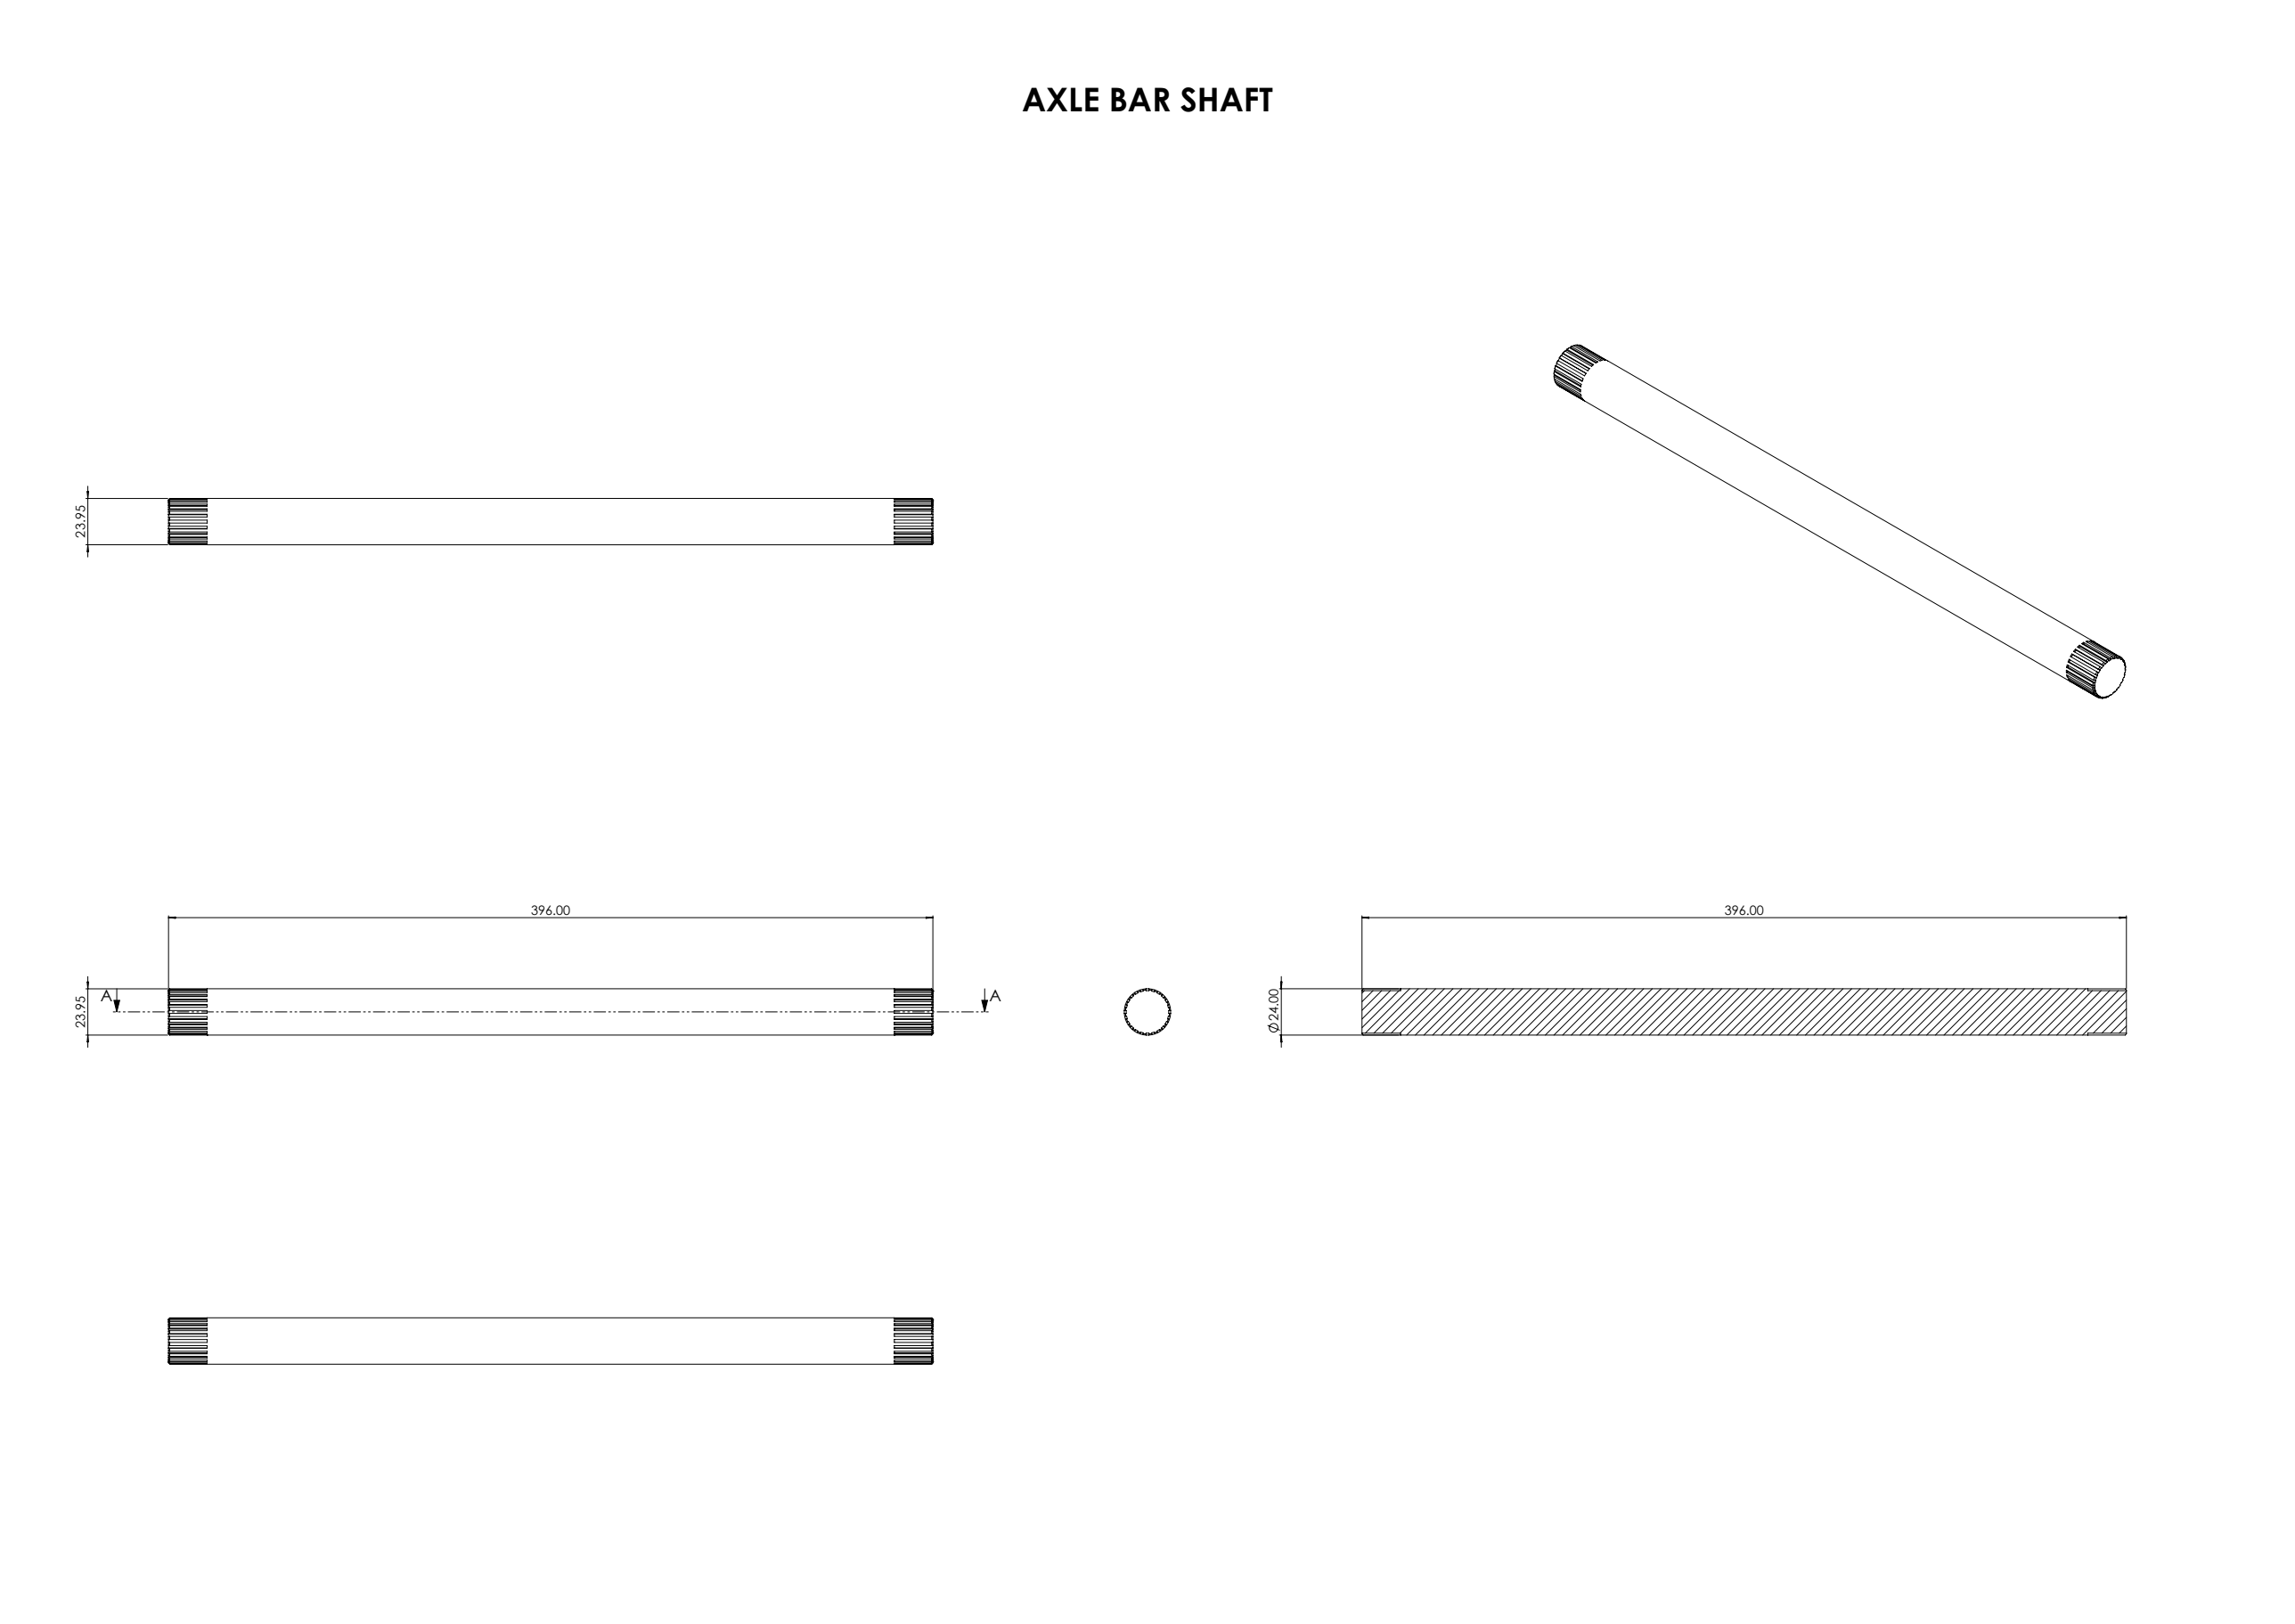
ISO-10303-21;
HEADER;
/* Generated by software containing ST-Developer
 * from STEP Tools, Inc. (www.steptools.com) 
 */

FILE_DESCRIPTION(
/* description */ (''),
/* implementation_level */ '2;1');

FILE_NAME(
/* name */ '10_Axle_Bar_Shaft.step',
/* time_stamp */ '2026-10-11T12:57:03-07:00',
/* author */ (''),
/* organization */ (''),
/* preprocessor_version */ 'ST-DEVELOPER v20.2',
/* originating_system */ 'Autodesk Translation Framework v15.15.0.0',
/* authorisation */ '');

FILE_SCHEMA (('AUTOMOTIVE_DESIGN { 1 0 10303 214 3 1 1 }'));
ENDSEC;

DATA;
#10=MECHANICAL_DESIGN_GEOMETRIC_PRESENTATION_REPRESENTATION('',(#265),#90374);
#231=SHAPE_REPRESENTATION_RELATIONSHIP('SRR','None',#90450,#248);
#248=ADVANCED_BREP_SHAPE_REPRESENTATION('',(#282),#90366);
#265=STYLED_ITEM('',(#90687),#282);
#282=MANIFOLD_SOLID_BREP('Body1',#40354);
#693=CONICAL_SURFACE('',#43949,11.7,0.785398163397428);
#694=CONICAL_SURFACE('',#43951,11.7,0.785398163397428);
#695=CONICAL_SURFACE('',#43957,11.7,0.785398163397428);
#696=CONICAL_SURFACE('',#43963,11.7,0.785398163397428);
#697=CONICAL_SURFACE('',#43969,11.7,0.785398163397428);
#698=CONICAL_SURFACE('',#43975,11.7,0.785398163397428);
#699=CONICAL_SURFACE('',#43981,11.7,0.785398163397428);
#700=CONICAL_SURFACE('',#43987,11.7,0.785398163397428);
#701=CONICAL_SURFACE('',#43993,11.7,0.785398163397428);
#702=CONICAL_SURFACE('',#43999,11.7,0.785398163397428);
#703=CONICAL_SURFACE('',#44005,11.7,0.785398163397428);
#704=CONICAL_SURFACE('',#44011,11.7,0.785398163397428);
#705=CONICAL_SURFACE('',#44017,11.7,0.785398163397428);
#706=CONICAL_SURFACE('',#44023,11.7,0.785398163397428);
#707=CONICAL_SURFACE('',#44029,11.7,0.785398163397428);
#708=CONICAL_SURFACE('',#44035,11.7,0.785398163397428);
#709=CONICAL_SURFACE('',#44041,11.7,0.785398163397428);
#710=CONICAL_SURFACE('',#44047,11.7,0.785398163397428);
#711=CONICAL_SURFACE('',#44053,11.7,0.785398163397428);
#712=CONICAL_SURFACE('',#44059,11.7,0.785398163397428);
#713=CONICAL_SURFACE('',#44065,11.7,0.785398163397428);
#714=CONICAL_SURFACE('',#44071,11.7,0.785398163397428);
#715=CONICAL_SURFACE('',#44077,11.7,0.785398163397428);
#716=CONICAL_SURFACE('',#44083,11.7,0.785398163397428);
#717=CONICAL_SURFACE('',#44118,11.7,0.785398163397457);
#718=CONICAL_SURFACE('',#44119,11.7,0.785398163397457);
#719=CONICAL_SURFACE('',#44124,11.7,0.785398163397457);
#720=CONICAL_SURFACE('',#44129,11.7,0.785398163397457);
#721=CONICAL_SURFACE('',#44134,11.7,0.785398163397457);
#722=CONICAL_SURFACE('',#44139,11.7,0.785398163397457);
#723=CONICAL_SURFACE('',#44144,11.7,0.785398163397457);
#724=CONICAL_SURFACE('',#44149,11.7,0.785398163397457);
#725=CONICAL_SURFACE('',#44154,11.7,0.785398163397457);
#726=CONICAL_SURFACE('',#44159,11.7,0.785398163397457);
#727=CONICAL_SURFACE('',#44164,11.7,0.785398163397457);
#728=CONICAL_SURFACE('',#44169,11.7,0.785398163397457);
#729=CONICAL_SURFACE('',#44174,11.7,0.785398163397457);
#730=CONICAL_SURFACE('',#44179,11.7,0.785398163397457);
#731=CONICAL_SURFACE('',#44184,11.7,0.785398163397457);
#732=CONICAL_SURFACE('',#44189,11.7,0.785398163397457);
#733=CONICAL_SURFACE('',#44194,11.7,0.785398163397457);
#734=CONICAL_SURFACE('',#44199,11.7,0.785398163397457);
#735=CONICAL_SURFACE('',#44204,11.7,0.785398163397457);
#736=CONICAL_SURFACE('',#44209,11.7,0.785398163397457);
#737=CONICAL_SURFACE('',#44214,11.7,0.785398163397457);
#738=CONICAL_SURFACE('',#44219,11.7,0.785398163397457);
#739=CONICAL_SURFACE('',#44224,11.7,0.785398163397457);
#740=CONICAL_SURFACE('',#44229,11.7,0.785398163397457);
#1443=PLANE('',#43846);
#1444=PLANE('',#43847);
#1445=PLANE('',#43849);
#1446=PLANE('',#43850);
#1447=PLANE('',#43953);
#1448=PLANE('',#43954);
#1449=PLANE('',#43955);
#1450=PLANE('',#43956);
#1451=PLANE('',#43959);
#1452=PLANE('',#43960);
#1453=PLANE('',#43961);
#1454=PLANE('',#43962);
#1455=PLANE('',#43965);
#1456=PLANE('',#43966);
#1457=PLANE('',#43967);
#1458=PLANE('',#43968);
#1459=PLANE('',#43971);
#1460=PLANE('',#43972);
#1461=PLANE('',#43973);
#1462=PLANE('',#43974);
#1463=PLANE('',#43977);
#1464=PLANE('',#43978);
#1465=PLANE('',#43979);
#1466=PLANE('',#43980);
#1467=PLANE('',#43983);
#1468=PLANE('',#43984);
#1469=PLANE('',#43985);
#1470=PLANE('',#43986);
#1471=PLANE('',#43989);
#1472=PLANE('',#43990);
#1473=PLANE('',#43991);
#1474=PLANE('',#43992);
#1475=PLANE('',#43995);
#1476=PLANE('',#43996);
#1477=PLANE('',#43997);
#1478=PLANE('',#43998);
#1479=PLANE('',#44001);
#1480=PLANE('',#44002);
#1481=PLANE('',#44003);
#1482=PLANE('',#44004);
#1483=PLANE('',#44007);
#1484=PLANE('',#44008);
#1485=PLANE('',#44009);
#1486=PLANE('',#44010);
#1487=PLANE('',#44013);
#1488=PLANE('',#44014);
#1489=PLANE('',#44015);
#1490=PLANE('',#44016);
#1491=PLANE('',#44019);
#1492=PLANE('',#44020);
#1493=PLANE('',#44021);
#1494=PLANE('',#44022);
#1495=PLANE('',#44025);
#1496=PLANE('',#44026);
#1497=PLANE('',#44027);
#1498=PLANE('',#44028);
#1499=PLANE('',#44031);
#1500=PLANE('',#44032);
#1501=PLANE('',#44033);
#1502=PLANE('',#44034);
#1503=PLANE('',#44037);
#1504=PLANE('',#44038);
#1505=PLANE('',#44039);
#1506=PLANE('',#44040);
#1507=PLANE('',#44043);
#1508=PLANE('',#44044);
#1509=PLANE('',#44045);
#1510=PLANE('',#44046);
#1511=PLANE('',#44049);
#1512=PLANE('',#44050);
#1513=PLANE('',#44051);
#1514=PLANE('',#44052);
#1515=PLANE('',#44055);
#1516=PLANE('',#44056);
#1517=PLANE('',#44057);
#1518=PLANE('',#44058);
#1519=PLANE('',#44061);
#1520=PLANE('',#44062);
#1521=PLANE('',#44063);
#1522=PLANE('',#44064);
#1523=PLANE('',#44067);
#1524=PLANE('',#44068);
#1525=PLANE('',#44069);
#1526=PLANE('',#44070);
#1527=PLANE('',#44073);
#1528=PLANE('',#44074);
#1529=PLANE('',#44075);
#1530=PLANE('',#44076);
#1531=PLANE('',#44079);
#1532=PLANE('',#44080);
#1533=PLANE('',#44081);
#1534=PLANE('',#44082);
#1535=PLANE('',#44085);
#1536=PLANE('',#44086);
#1537=PLANE('',#44087);
#1538=PLANE('',#44088);
#1539=PLANE('',#44089);
#1540=PLANE('',#44090);
#1541=PLANE('',#44091);
#1542=PLANE('',#44092);
#1543=PLANE('',#44093);
#1544=PLANE('',#44120);
#1545=PLANE('',#44121);
#1546=PLANE('',#44122);
#1547=PLANE('',#44123);
#1548=PLANE('',#44125);
#1549=PLANE('',#44126);
#1550=PLANE('',#44127);
#1551=PLANE('',#44128);
#1552=PLANE('',#44130);
#1553=PLANE('',#44131);
#1554=PLANE('',#44132);
#1555=PLANE('',#44133);
#1556=PLANE('',#44135);
#1557=PLANE('',#44136);
#1558=PLANE('',#44137);
#1559=PLANE('',#44138);
#1560=PLANE('',#44140);
#1561=PLANE('',#44141);
#1562=PLANE('',#44142);
#1563=PLANE('',#44143);
#1564=PLANE('',#44145);
#1565=PLANE('',#44146);
#1566=PLANE('',#44147);
#1567=PLANE('',#44148);
#1568=PLANE('',#44150);
#1569=PLANE('',#44151);
#1570=PLANE('',#44152);
#1571=PLANE('',#44153);
#1572=PLANE('',#44155);
#1573=PLANE('',#44156);
#1574=PLANE('',#44157);
#1575=PLANE('',#44158);
#1576=PLANE('',#44160);
#1577=PLANE('',#44161);
#1578=PLANE('',#44162);
#1579=PLANE('',#44163);
#1580=PLANE('',#44165);
#1581=PLANE('',#44166);
#1582=PLANE('',#44167);
#1583=PLANE('',#44168);
#1584=PLANE('',#44170);
#1585=PLANE('',#44171);
#1586=PLANE('',#44172);
#1587=PLANE('',#44173);
#1588=PLANE('',#44175);
#1589=PLANE('',#44176);
#1590=PLANE('',#44177);
#1591=PLANE('',#44178);
#1592=PLANE('',#44180);
#1593=PLANE('',#44181);
#1594=PLANE('',#44182);
#1595=PLANE('',#44183);
#1596=PLANE('',#44185);
#1597=PLANE('',#44186);
#1598=PLANE('',#44187);
#1599=PLANE('',#44188);
#1600=PLANE('',#44190);
#1601=PLANE('',#44191);
#1602=PLANE('',#44192);
#1603=PLANE('',#44193);
#1604=PLANE('',#44195);
#1605=PLANE('',#44196);
#1606=PLANE('',#44197);
#1607=PLANE('',#44198);
#1608=PLANE('',#44200);
#1609=PLANE('',#44201);
#1610=PLANE('',#44202);
#1611=PLANE('',#44203);
#1612=PLANE('',#44205);
#1613=PLANE('',#44206);
#1614=PLANE('',#44207);
#1615=PLANE('',#44208);
#1616=PLANE('',#44210);
#1617=PLANE('',#44211);
#1618=PLANE('',#44212);
#1619=PLANE('',#44213);
#1620=PLANE('',#44215);
#1621=PLANE('',#44216);
#1622=PLANE('',#44217);
#1623=PLANE('',#44218);
#1624=PLANE('',#44220);
#1625=PLANE('',#44221);
#1626=PLANE('',#44222);
#1627=PLANE('',#44223);
#1628=PLANE('',#44225);
#1629=PLANE('',#44226);
#1630=PLANE('',#44227);
#1631=PLANE('',#44228);
#1632=PLANE('',#44230);
#1633=PLANE('',#44231);
#1634=PLANE('',#44232);
#1635=PLANE('',#44233);
#1636=PLANE('',#44234);
#1833=(
BOUNDED_CURVE()
B_SPLINE_CURVE(2,(#83032,#83033,#83034),.UNSPECIFIED.,.F.,.F.)
B_SPLINE_CURVE_WITH_KNOTS((3,3),(0.,0.0849403543350642),.UNSPECIFIED.)
CURVE()
GEOMETRIC_REPRESENTATION_ITEM()
RATIONAL_B_SPLINE_CURVE((1.,1.00033025160276,1.))
REPRESENTATION_ITEM('')
);
#1834=(
BOUNDED_CURVE()
B_SPLINE_CURVE(2,(#83046,#83047,#83048),.UNSPECIFIED.,.F.,.F.)
B_SPLINE_CURVE_WITH_KNOTS((3,3),(0.,0.0849403543350645),.UNSPECIFIED.)
CURVE()
GEOMETRIC_REPRESENTATION_ITEM()
RATIONAL_B_SPLINE_CURVE((1.,1.00033025241417,1.))
REPRESENTATION_ITEM('')
);
#1835=(
BOUNDED_CURVE()
B_SPLINE_CURVE(2,(#83439,#83440,#83441),.UNSPECIFIED.,.F.,.F.)
B_SPLINE_CURVE_WITH_KNOTS((3,3),(0.,0.0849403543350642),.UNSPECIFIED.)
CURVE()
GEOMETRIC_REPRESENTATION_ITEM()
RATIONAL_B_SPLINE_CURVE((1.,1.00033025173132,1.))
REPRESENTATION_ITEM('')
);
#1836=(
BOUNDED_CURVE()
B_SPLINE_CURVE(2,(#83444,#83445,#83446),.UNSPECIFIED.,.F.,.F.)
B_SPLINE_CURVE_WITH_KNOTS((3,3),(0.,0.0849403543350642),.UNSPECIFIED.)
CURVE()
GEOMETRIC_REPRESENTATION_ITEM()
RATIONAL_B_SPLINE_CURVE((1.,1.00033025019403,1.))
REPRESENTATION_ITEM('')
);
#1837=(
BOUNDED_CURVE()
B_SPLINE_CURVE(2,(#83462,#83463,#83464),.UNSPECIFIED.,.F.,.F.)
B_SPLINE_CURVE_WITH_KNOTS((3,3),(0.,0.0849403543350642),.UNSPECIFIED.)
CURVE()
GEOMETRIC_REPRESENTATION_ITEM()
RATIONAL_B_SPLINE_CURVE((1.,1.00033025228575,1.))
REPRESENTATION_ITEM('')
);
#1838=(
BOUNDED_CURVE()
B_SPLINE_CURVE(2,(#83471,#83472,#83473),.UNSPECIFIED.,.F.,.F.)
B_SPLINE_CURVE_WITH_KNOTS((3,3),(0.,0.0849403543350642),.UNSPECIFIED.)
CURVE()
GEOMETRIC_REPRESENTATION_ITEM()
RATIONAL_B_SPLINE_CURVE((1.,1.00033024976505,1.))
REPRESENTATION_ITEM('')
);
#1839=(
BOUNDED_CURVE()
B_SPLINE_CURVE(2,(#83488,#83489,#83490),.UNSPECIFIED.,.F.,.F.)
B_SPLINE_CURVE_WITH_KNOTS((3,3),(0.,0.0849403543350642),.UNSPECIFIED.)
CURVE()
GEOMETRIC_REPRESENTATION_ITEM()
RATIONAL_B_SPLINE_CURVE((1.,1.00033025048873,1.))
REPRESENTATION_ITEM('')
);
#1840=(
BOUNDED_CURVE()
B_SPLINE_CURVE(2,(#83497,#83498,#83499),.UNSPECIFIED.,.F.,.F.)
B_SPLINE_CURVE_WITH_KNOTS((3,3),(0.,0.0849403543350643),.UNSPECIFIED.)
CURVE()
GEOMETRIC_REPRESENTATION_ITEM()
RATIONAL_B_SPLINE_CURVE((1.,1.00033025205034,1.))
REPRESENTATION_ITEM('')
);
#1841=(
BOUNDED_CURVE()
B_SPLINE_CURVE(2,(#83514,#83515,#83516),.UNSPECIFIED.,.F.,.F.)
B_SPLINE_CURVE_WITH_KNOTS((3,3),(0.,0.084940354335064),.UNSPECIFIED.)
CURVE()
GEOMETRIC_REPRESENTATION_ITEM()
RATIONAL_B_SPLINE_CURVE((1.,1.00033025029154,1.))
REPRESENTATION_ITEM('')
);
#1842=(
BOUNDED_CURVE()
B_SPLINE_CURVE(2,(#83523,#83524,#83525),.UNSPECIFIED.,.F.,.F.)
B_SPLINE_CURVE_WITH_KNOTS((3,3),(0.,0.0849403543350643),.UNSPECIFIED.)
CURVE()
GEOMETRIC_REPRESENTATION_ITEM()
RATIONAL_B_SPLINE_CURVE((1.,1.00033025291298,1.))
REPRESENTATION_ITEM('')
);
#1843=(
BOUNDED_CURVE()
B_SPLINE_CURVE(2,(#83540,#83541,#83542),.UNSPECIFIED.,.F.,.F.)
B_SPLINE_CURVE_WITH_KNOTS((3,3),(0.,0.0849403543350644),.UNSPECIFIED.)
CURVE()
GEOMETRIC_REPRESENTATION_ITEM()
RATIONAL_B_SPLINE_CURVE((1.,1.00033025022527,1.))
REPRESENTATION_ITEM('')
);
#1844=(
BOUNDED_CURVE()
B_SPLINE_CURVE(2,(#83549,#83550,#83551),.UNSPECIFIED.,.F.,.F.)
B_SPLINE_CURVE_WITH_KNOTS((3,3),(0.,0.0849403543350642),.UNSPECIFIED.)
CURVE()
GEOMETRIC_REPRESENTATION_ITEM()
RATIONAL_B_SPLINE_CURVE((1.,1.00033025176016,1.))
REPRESENTATION_ITEM('')
);
#1845=(
BOUNDED_CURVE()
B_SPLINE_CURVE(2,(#83566,#83567,#83568),.UNSPECIFIED.,.F.,.F.)
B_SPLINE_CURVE_WITH_KNOTS((3,3),(0.,0.0849403543350642),.UNSPECIFIED.)
CURVE()
GEOMETRIC_REPRESENTATION_ITEM()
RATIONAL_B_SPLINE_CURVE((1.,1.00033025172446,1.))
REPRESENTATION_ITEM('')
);
#1846=(
BOUNDED_CURVE()
B_SPLINE_CURVE(2,(#83575,#83576,#83577),.UNSPECIFIED.,.F.,.F.)
B_SPLINE_CURVE_WITH_KNOTS((3,3),(0.,0.0849403543350642),.UNSPECIFIED.)
CURVE()
GEOMETRIC_REPRESENTATION_ITEM()
RATIONAL_B_SPLINE_CURVE((1.,1.00033025024162,1.))
REPRESENTATION_ITEM('')
);
#1847=(
BOUNDED_CURVE()
B_SPLINE_CURVE(2,(#83592,#83593,#83594),.UNSPECIFIED.,.F.,.F.)
B_SPLINE_CURVE_WITH_KNOTS((3,3),(0.,0.0849403543350645),.UNSPECIFIED.)
CURVE()
GEOMETRIC_REPRESENTATION_ITEM()
RATIONAL_B_SPLINE_CURVE((1.,1.00033025047704,1.))
REPRESENTATION_ITEM('')
);
#1848=(
BOUNDED_CURVE()
B_SPLINE_CURVE(2,(#83601,#83602,#83603),.UNSPECIFIED.,.F.,.F.)
B_SPLINE_CURVE_WITH_KNOTS((3,3),(0.,0.0849403543350642),.UNSPECIFIED.)
CURVE()
GEOMETRIC_REPRESENTATION_ITEM()
RATIONAL_B_SPLINE_CURVE((1.,1.0003302538932,1.))
REPRESENTATION_ITEM('')
);
#1849=(
BOUNDED_CURVE()
B_SPLINE_CURVE(2,(#83618,#83619,#83620),.UNSPECIFIED.,.F.,.F.)
B_SPLINE_CURVE_WITH_KNOTS((3,3),(0.,0.0849403543350642),.UNSPECIFIED.)
CURVE()
GEOMETRIC_REPRESENTATION_ITEM()
RATIONAL_B_SPLINE_CURVE((1.,1.00033025055311,1.))
REPRESENTATION_ITEM('')
);
#1850=(
BOUNDED_CURVE()
B_SPLINE_CURVE(2,(#83627,#83628,#83629),.UNSPECIFIED.,.F.,.F.)
B_SPLINE_CURVE_WITH_KNOTS((3,3),(0.,0.0849403543350642),.UNSPECIFIED.)
CURVE()
GEOMETRIC_REPRESENTATION_ITEM()
RATIONAL_B_SPLINE_CURVE((1.,1.00033025068821,1.))
REPRESENTATION_ITEM('')
);
#1851=(
BOUNDED_CURVE()
B_SPLINE_CURVE(2,(#83644,#83645,#83646),.UNSPECIFIED.,.F.,.F.)
B_SPLINE_CURVE_WITH_KNOTS((3,3),(0.,0.0849403543350642),.UNSPECIFIED.)
CURVE()
GEOMETRIC_REPRESENTATION_ITEM()
RATIONAL_B_SPLINE_CURVE((1.,1.00033025088247,1.))
REPRESENTATION_ITEM('')
);
#1852=(
BOUNDED_CURVE()
B_SPLINE_CURVE(2,(#83653,#83654,#83655),.UNSPECIFIED.,.F.,.F.)
B_SPLINE_CURVE_WITH_KNOTS((3,3),(0.,0.0849403543350642),.UNSPECIFIED.)
CURVE()
GEOMETRIC_REPRESENTATION_ITEM()
RATIONAL_B_SPLINE_CURVE((1.,1.00033025566741,1.))
REPRESENTATION_ITEM('')
);
#1853=(
BOUNDED_CURVE()
B_SPLINE_CURVE(2,(#83670,#83671,#83672),.UNSPECIFIED.,.F.,.F.)
B_SPLINE_CURVE_WITH_KNOTS((3,3),(0.,0.0849403543350643),.UNSPECIFIED.)
CURVE()
GEOMETRIC_REPRESENTATION_ITEM()
RATIONAL_B_SPLINE_CURVE((1.,1.00033025086662,1.))
REPRESENTATION_ITEM('')
);
#1854=(
BOUNDED_CURVE()
B_SPLINE_CURVE(2,(#83679,#83680,#83681),.UNSPECIFIED.,.F.,.F.)
B_SPLINE_CURVE_WITH_KNOTS((3,3),(0.,0.0849403543350643),.UNSPECIFIED.)
CURVE()
GEOMETRIC_REPRESENTATION_ITEM()
RATIONAL_B_SPLINE_CURVE((1.,1.00033025126855,1.))
REPRESENTATION_ITEM('')
);
#1855=(
BOUNDED_CURVE()
B_SPLINE_CURVE(2,(#83696,#83697,#83698),.UNSPECIFIED.,.F.,.F.)
B_SPLINE_CURVE_WITH_KNOTS((3,3),(0.,0.0849403543350644),.UNSPECIFIED.)
CURVE()
GEOMETRIC_REPRESENTATION_ITEM()
RATIONAL_B_SPLINE_CURVE((1.,1.00033025048324,1.))
REPRESENTATION_ITEM('')
);
#1856=(
BOUNDED_CURVE()
B_SPLINE_CURVE(2,(#83705,#83706,#83707),.UNSPECIFIED.,.F.,.F.)
B_SPLINE_CURVE_WITH_KNOTS((3,3),(0.,0.0849403543350642),.UNSPECIFIED.)
CURVE()
GEOMETRIC_REPRESENTATION_ITEM()
RATIONAL_B_SPLINE_CURVE((1.,1.00033025019805,1.))
REPRESENTATION_ITEM('')
);
#1857=(
BOUNDED_CURVE()
B_SPLINE_CURVE(2,(#83722,#83723,#83724),.UNSPECIFIED.,.F.,.F.)
B_SPLINE_CURVE_WITH_KNOTS((3,3),(0.,0.0849403543350642),.UNSPECIFIED.)
CURVE()
GEOMETRIC_REPRESENTATION_ITEM()
RATIONAL_B_SPLINE_CURVE((1.,1.00033025018713,1.))
REPRESENTATION_ITEM('')
);
#1858=(
BOUNDED_CURVE()
B_SPLINE_CURVE(2,(#83731,#83732,#83733),.UNSPECIFIED.,.F.,.F.)
B_SPLINE_CURVE_WITH_KNOTS((3,3),(0.,0.0849403543350641),.UNSPECIFIED.)
CURVE()
GEOMETRIC_REPRESENTATION_ITEM()
RATIONAL_B_SPLINE_CURVE((1.,1.00033025306809,1.))
REPRESENTATION_ITEM('')
);
#1859=(
BOUNDED_CURVE()
B_SPLINE_CURVE(2,(#83748,#83749,#83750),.UNSPECIFIED.,.F.,.F.)
B_SPLINE_CURVE_WITH_KNOTS((3,3),(0.,0.0849403543350642),.UNSPECIFIED.)
CURVE()
GEOMETRIC_REPRESENTATION_ITEM()
RATIONAL_B_SPLINE_CURVE((1.,1.00033025283671,1.))
REPRESENTATION_ITEM('')
);
#1860=(
BOUNDED_CURVE()
B_SPLINE_CURVE(2,(#83757,#83758,#83759),.UNSPECIFIED.,.F.,.F.)
B_SPLINE_CURVE_WITH_KNOTS((3,3),(0.,0.0849403543350642),.UNSPECIFIED.)
CURVE()
GEOMETRIC_REPRESENTATION_ITEM()
RATIONAL_B_SPLINE_CURVE((1.,1.00033025201275,1.))
REPRESENTATION_ITEM('')
);
#1861=(
BOUNDED_CURVE()
B_SPLINE_CURVE(2,(#83774,#83775,#83776),.UNSPECIFIED.,.F.,.F.)
B_SPLINE_CURVE_WITH_KNOTS((3,3),(0.,0.0849403543350643),.UNSPECIFIED.)
CURVE()
GEOMETRIC_REPRESENTATION_ITEM()
RATIONAL_B_SPLINE_CURVE((1.,1.0003302506393,1.))
REPRESENTATION_ITEM('')
);
#1862=(
BOUNDED_CURVE()
B_SPLINE_CURVE(2,(#83783,#83784,#83785),.UNSPECIFIED.,.F.,.F.)
B_SPLINE_CURVE_WITH_KNOTS((3,3),(0.,0.0849403543350642),.UNSPECIFIED.)
CURVE()
GEOMETRIC_REPRESENTATION_ITEM()
RATIONAL_B_SPLINE_CURVE((1.,1.00033025057128,1.))
REPRESENTATION_ITEM('')
);
#1863=(
BOUNDED_CURVE()
B_SPLINE_CURVE(2,(#83800,#83801,#83802),.UNSPECIFIED.,.F.,.F.)
B_SPLINE_CURVE_WITH_KNOTS((3,3),(0.,0.0849403543350642),.UNSPECIFIED.)
CURVE()
GEOMETRIC_REPRESENTATION_ITEM()
RATIONAL_B_SPLINE_CURVE((1.,1.00033025068354,1.))
REPRESENTATION_ITEM('')
);
#1864=(
BOUNDED_CURVE()
B_SPLINE_CURVE(2,(#83809,#83810,#83811),.UNSPECIFIED.,.F.,.F.)
B_SPLINE_CURVE_WITH_KNOTS((3,3),(0.,0.0849403543350641),.UNSPECIFIED.)
CURVE()
GEOMETRIC_REPRESENTATION_ITEM()
RATIONAL_B_SPLINE_CURVE((1.,1.0003302507014,1.))
REPRESENTATION_ITEM('')
);
#1865=(
BOUNDED_CURVE()
B_SPLINE_CURVE(2,(#83826,#83827,#83828),.UNSPECIFIED.,.F.,.F.)
B_SPLINE_CURVE_WITH_KNOTS((3,3),(0.,0.0849403543350642),.UNSPECIFIED.)
CURVE()
GEOMETRIC_REPRESENTATION_ITEM()
RATIONAL_B_SPLINE_CURVE((1.,1.00033024942034,1.))
REPRESENTATION_ITEM('')
);
#1866=(
BOUNDED_CURVE()
B_SPLINE_CURVE(2,(#83835,#83836,#83837),.UNSPECIFIED.,.F.,.F.)
B_SPLINE_CURVE_WITH_KNOTS((3,3),(0.,0.0849403543350642),.UNSPECIFIED.)
CURVE()
GEOMETRIC_REPRESENTATION_ITEM()
RATIONAL_B_SPLINE_CURVE((1.,1.00033025025859,1.))
REPRESENTATION_ITEM('')
);
#1867=(
BOUNDED_CURVE()
B_SPLINE_CURVE(2,(#83852,#83853,#83854),.UNSPECIFIED.,.F.,.F.)
B_SPLINE_CURVE_WITH_KNOTS((3,3),(0.,0.0849403543350642),.UNSPECIFIED.)
CURVE()
GEOMETRIC_REPRESENTATION_ITEM()
RATIONAL_B_SPLINE_CURVE((1.,1.00033025417478,1.))
REPRESENTATION_ITEM('')
);
#1868=(
BOUNDED_CURVE()
B_SPLINE_CURVE(2,(#83861,#83862,#83863),.UNSPECIFIED.,.F.,.F.)
B_SPLINE_CURVE_WITH_KNOTS((3,3),(0.,0.0849403543350642),.UNSPECIFIED.)
CURVE()
GEOMETRIC_REPRESENTATION_ITEM()
RATIONAL_B_SPLINE_CURVE((1.,1.00033025175498,1.))
REPRESENTATION_ITEM('')
);
#1869=(
BOUNDED_CURVE()
B_SPLINE_CURVE(2,(#83878,#83879,#83880),.UNSPECIFIED.,.F.,.F.)
B_SPLINE_CURVE_WITH_KNOTS((3,3),(0.,0.0849403543350642),.UNSPECIFIED.)
CURVE()
GEOMETRIC_REPRESENTATION_ITEM()
RATIONAL_B_SPLINE_CURVE((1.,1.00033025172964,1.))
REPRESENTATION_ITEM('')
);
#1870=(
BOUNDED_CURVE()
B_SPLINE_CURVE(2,(#83887,#83888,#83889),.UNSPECIFIED.,.F.,.F.)
B_SPLINE_CURVE_WITH_KNOTS((3,3),(0.,0.0849403543350641),.UNSPECIFIED.)
CURVE()
GEOMETRIC_REPRESENTATION_ITEM()
RATIONAL_B_SPLINE_CURVE((1.,1.00033025185005,1.))
REPRESENTATION_ITEM('')
);
#1871=(
BOUNDED_CURVE()
B_SPLINE_CURVE(2,(#83904,#83905,#83906),.UNSPECIFIED.,.F.,.F.)
B_SPLINE_CURVE_WITH_KNOTS((3,3),(0.,0.0849403543350642),.UNSPECIFIED.)
CURVE()
GEOMETRIC_REPRESENTATION_ITEM()
RATIONAL_B_SPLINE_CURVE((1.,1.00033024993968,1.))
REPRESENTATION_ITEM('')
);
#1872=(
BOUNDED_CURVE()
B_SPLINE_CURVE(2,(#83913,#83914,#83915),.UNSPECIFIED.,.F.,.F.)
B_SPLINE_CURVE_WITH_KNOTS((3,3),(0.,0.084940354335064),.UNSPECIFIED.)
CURVE()
GEOMETRIC_REPRESENTATION_ITEM()
RATIONAL_B_SPLINE_CURVE((1.,1.00033025201589,1.))
REPRESENTATION_ITEM('')
);
#1873=(
BOUNDED_CURVE()
B_SPLINE_CURVE(2,(#83930,#83931,#83932),.UNSPECIFIED.,.F.,.F.)
B_SPLINE_CURVE_WITH_KNOTS((3,3),(0.,0.0849403543350641),.UNSPECIFIED.)
CURVE()
GEOMETRIC_REPRESENTATION_ITEM()
RATIONAL_B_SPLINE_CURVE((1.,1.00033025407768,1.))
REPRESENTATION_ITEM('')
);
#1874=(
BOUNDED_CURVE()
B_SPLINE_CURVE(2,(#83939,#83940,#83941),.UNSPECIFIED.,.F.,.F.)
B_SPLINE_CURVE_WITH_KNOTS((3,3),(0.,0.0849403543350642),.UNSPECIFIED.)
CURVE()
GEOMETRIC_REPRESENTATION_ITEM()
RATIONAL_B_SPLINE_CURVE((1.,1.00033025202778,1.))
REPRESENTATION_ITEM('')
);
#1875=(
BOUNDED_CURVE()
B_SPLINE_CURVE(2,(#83956,#83957,#83958),.UNSPECIFIED.,.F.,.F.)
B_SPLINE_CURVE_WITH_KNOTS((3,3),(0.,0.0849403543350642),.UNSPECIFIED.)
CURVE()
GEOMETRIC_REPRESENTATION_ITEM()
RATIONAL_B_SPLINE_CURVE((1.,1.00033025202127,1.))
REPRESENTATION_ITEM('')
);
#1876=(
BOUNDED_CURVE()
B_SPLINE_CURVE(2,(#83965,#83966,#83967),.UNSPECIFIED.,.F.,.F.)
B_SPLINE_CURVE_WITH_KNOTS((3,3),(0.,0.0849403543350642),.UNSPECIFIED.)
CURVE()
GEOMETRIC_REPRESENTATION_ITEM()
RATIONAL_B_SPLINE_CURVE((1.,1.0003302492308,1.))
REPRESENTATION_ITEM('')
);
#1877=(
BOUNDED_CURVE()
B_SPLINE_CURVE(2,(#83982,#83983,#83984),.UNSPECIFIED.,.F.,.F.)
B_SPLINE_CURVE_WITH_KNOTS((3,3),(0.,0.0849403543350642),.UNSPECIFIED.)
CURVE()
GEOMETRIC_REPRESENTATION_ITEM()
RATIONAL_B_SPLINE_CURVE((1.,1.00033024979139,1.))
REPRESENTATION_ITEM('')
);
#1878=(
BOUNDED_CURVE()
B_SPLINE_CURVE(2,(#83991,#83992,#83993),.UNSPECIFIED.,.F.,.F.)
B_SPLINE_CURVE_WITH_KNOTS((3,3),(0.,0.0849403543350642),.UNSPECIFIED.)
CURVE()
GEOMETRIC_REPRESENTATION_ITEM()
RATIONAL_B_SPLINE_CURVE((1.,1.00033024938276,1.))
REPRESENTATION_ITEM('')
);
#1879=(
BOUNDED_CURVE()
B_SPLINE_CURVE(2,(#84008,#84009,#84010),.UNSPECIFIED.,.F.,.F.)
B_SPLINE_CURVE_WITH_KNOTS((3,3),(0.,0.0849403543350641),.UNSPECIFIED.)
CURVE()
GEOMETRIC_REPRESENTATION_ITEM()
RATIONAL_B_SPLINE_CURVE((1.,1.00033025441577,1.))
REPRESENTATION_ITEM('')
);
#1880=(
BOUNDED_CURVE()
B_SPLINE_CURVE(2,(#84017,#84018,#84019),.UNSPECIFIED.,.F.,.F.)
B_SPLINE_CURVE_WITH_KNOTS((3,3),(0.,0.0849403543350642),.UNSPECIFIED.)
CURVE()
GEOMETRIC_REPRESENTATION_ITEM()
RATIONAL_B_SPLINE_CURVE((1.,1.00033025019403,1.))
REPRESENTATION_ITEM('')
);
#1881=(
BOUNDED_CURVE()
B_SPLINE_CURVE(2,(#84043,#84044,#84045),.UNSPECIFIED.,.F.,.F.)
B_SPLINE_CURVE_WITH_KNOTS((3,3),(0.,0.0849403543350617),.UNSPECIFIED.)
CURVE()
GEOMETRIC_REPRESENTATION_ITEM()
RATIONAL_B_SPLINE_CURVE((1.,1.00033025151332,1.))
REPRESENTATION_ITEM('')
);
#1882=(
BOUNDED_CURVE()
B_SPLINE_CURVE(2,(#84054,#84055,#84056),.UNSPECIFIED.,.F.,.F.)
B_SPLINE_CURVE_WITH_KNOTS((3,3),(0.,0.0849403543350617),.UNSPECIFIED.)
CURVE()
GEOMETRIC_REPRESENTATION_ITEM()
RATIONAL_B_SPLINE_CURVE((1.,1.00033025246357,1.))
REPRESENTATION_ITEM('')
);
#1883=(
BOUNDED_CURVE()
B_SPLINE_CURVE(2,(#84247,#84248,#84249),.UNSPECIFIED.,.F.,.F.)
B_SPLINE_CURVE_WITH_KNOTS((3,3),(0.,0.0849403543350617),.UNSPECIFIED.)
CURVE()
GEOMETRIC_REPRESENTATION_ITEM()
RATIONAL_B_SPLINE_CURVE((1.,1.0003302512864,1.))
REPRESENTATION_ITEM('')
);
#1884=(
BOUNDED_CURVE()
B_SPLINE_CURVE(2,(#84251,#84252,#84253),.UNSPECIFIED.,.F.,.F.)
B_SPLINE_CURVE_WITH_KNOTS((3,3),(0.,0.0849403543350617),.UNSPECIFIED.)
CURVE()
GEOMETRIC_REPRESENTATION_ITEM()
RATIONAL_B_SPLINE_CURVE((1.,1.00033025136034,1.))
REPRESENTATION_ITEM('')
);
#1885=(
BOUNDED_CURVE()
B_SPLINE_CURVE(2,(#84263,#84264,#84265),.UNSPECIFIED.,.F.,.F.)
B_SPLINE_CURVE_WITH_KNOTS((3,3),(0.,0.0849403543350619),.UNSPECIFIED.)
CURVE()
GEOMETRIC_REPRESENTATION_ITEM()
RATIONAL_B_SPLINE_CURVE((1.,1.00033025257346,1.))
REPRESENTATION_ITEM('')
);
#1886=(
BOUNDED_CURVE()
B_SPLINE_CURVE(2,(#84269,#84270,#84271),.UNSPECIFIED.,.F.,.F.)
B_SPLINE_CURVE_WITH_KNOTS((3,3),(0.,0.0849403543350618),.UNSPECIFIED.)
CURVE()
GEOMETRIC_REPRESENTATION_ITEM()
RATIONAL_B_SPLINE_CURVE((1.,1.00033025219394,1.))
REPRESENTATION_ITEM('')
);
#1887=(
BOUNDED_CURVE()
B_SPLINE_CURVE(2,(#84281,#84282,#84283),.UNSPECIFIED.,.F.,.F.)
B_SPLINE_CURVE_WITH_KNOTS((3,3),(0.,0.0849403543350616),.UNSPECIFIED.)
CURVE()
GEOMETRIC_REPRESENTATION_ITEM()
RATIONAL_B_SPLINE_CURVE((1.,1.00033025178113,1.))
REPRESENTATION_ITEM('')
);
#1888=(
BOUNDED_CURVE()
B_SPLINE_CURVE(2,(#84287,#84288,#84289),.UNSPECIFIED.,.F.,.F.)
B_SPLINE_CURVE_WITH_KNOTS((3,3),(0.,0.0849403543350617),.UNSPECIFIED.)
CURVE()
GEOMETRIC_REPRESENTATION_ITEM()
RATIONAL_B_SPLINE_CURVE((1.,1.00033025122766,1.))
REPRESENTATION_ITEM('')
);
#1889=(
BOUNDED_CURVE()
B_SPLINE_CURVE(2,(#84299,#84300,#84301),.UNSPECIFIED.,.F.,.F.)
B_SPLINE_CURVE_WITH_KNOTS((3,3),(0.,0.0849403543350618),.UNSPECIFIED.)
CURVE()
GEOMETRIC_REPRESENTATION_ITEM()
RATIONAL_B_SPLINE_CURVE((1.,1.00033025251487,1.))
REPRESENTATION_ITEM('')
);
#1890=(
BOUNDED_CURVE()
B_SPLINE_CURVE(2,(#84305,#84306,#84307),.UNSPECIFIED.,.F.,.F.)
B_SPLINE_CURVE_WITH_KNOTS((3,3),(0.,0.0849403543350618),.UNSPECIFIED.)
CURVE()
GEOMETRIC_REPRESENTATION_ITEM()
RATIONAL_B_SPLINE_CURVE((1.,1.00033025272764,1.))
REPRESENTATION_ITEM('')
);
#1891=(
BOUNDED_CURVE()
B_SPLINE_CURVE(2,(#84317,#84318,#84319),.UNSPECIFIED.,.F.,.F.)
B_SPLINE_CURVE_WITH_KNOTS((3,3),(0.,0.0849403543350617),.UNSPECIFIED.)
CURVE()
GEOMETRIC_REPRESENTATION_ITEM()
RATIONAL_B_SPLINE_CURVE((1.,1.00033025312403,1.))
REPRESENTATION_ITEM('')
);
#1892=(
BOUNDED_CURVE()
B_SPLINE_CURVE(2,(#84323,#84324,#84325),.UNSPECIFIED.,.F.,.F.)
B_SPLINE_CURVE_WITH_KNOTS((3,3),(0.,0.0849403543350617),.UNSPECIFIED.)
CURVE()
GEOMETRIC_REPRESENTATION_ITEM()
RATIONAL_B_SPLINE_CURVE((1.,1.00033025173859,1.))
REPRESENTATION_ITEM('')
);
#1893=(
BOUNDED_CURVE()
B_SPLINE_CURVE(2,(#84335,#84336,#84337),.UNSPECIFIED.,.F.,.F.)
B_SPLINE_CURVE_WITH_KNOTS((3,3),(0.,0.0849403543350618),.UNSPECIFIED.)
CURVE()
GEOMETRIC_REPRESENTATION_ITEM()
RATIONAL_B_SPLINE_CURVE((1.,1.00033025134825,1.))
REPRESENTATION_ITEM('')
);
#1894=(
BOUNDED_CURVE()
B_SPLINE_CURVE(2,(#84341,#84342,#84343),.UNSPECIFIED.,.F.,.F.)
B_SPLINE_CURVE_WITH_KNOTS((3,3),(0.,0.0849403543350617),.UNSPECIFIED.)
CURVE()
GEOMETRIC_REPRESENTATION_ITEM()
RATIONAL_B_SPLINE_CURVE((1.,1.0003302517462,1.))
REPRESENTATION_ITEM('')
);
#1895=(
BOUNDED_CURVE()
B_SPLINE_CURVE(2,(#84353,#84354,#84355),.UNSPECIFIED.,.F.,.F.)
B_SPLINE_CURVE_WITH_KNOTS((3,3),(0.,0.0849403543350617),.UNSPECIFIED.)
CURVE()
GEOMETRIC_REPRESENTATION_ITEM()
RATIONAL_B_SPLINE_CURVE((1.,1.00033025081262,1.))
REPRESENTATION_ITEM('')
);
#1896=(
BOUNDED_CURVE()
B_SPLINE_CURVE(2,(#84359,#84360,#84361),.UNSPECIFIED.,.F.,.F.)
B_SPLINE_CURVE_WITH_KNOTS((3,3),(0.,0.0849403543350616),.UNSPECIFIED.)
CURVE()
GEOMETRIC_REPRESENTATION_ITEM()
RATIONAL_B_SPLINE_CURVE((1.,1.00033025056284,1.))
REPRESENTATION_ITEM('')
);
#1897=(
BOUNDED_CURVE()
B_SPLINE_CURVE(2,(#84371,#84372,#84373),.UNSPECIFIED.,.F.,.F.)
B_SPLINE_CURVE_WITH_KNOTS((3,3),(0.,0.0849403543350619),.UNSPECIFIED.)
CURVE()
GEOMETRIC_REPRESENTATION_ITEM()
RATIONAL_B_SPLINE_CURVE((1.,1.00033025256946,1.))
REPRESENTATION_ITEM('')
);
#1898=(
BOUNDED_CURVE()
B_SPLINE_CURVE(2,(#84377,#84378,#84379),.UNSPECIFIED.,.F.,.F.)
B_SPLINE_CURVE_WITH_KNOTS((3,3),(0.,0.0849403543350618),.UNSPECIFIED.)
CURVE()
GEOMETRIC_REPRESENTATION_ITEM()
RATIONAL_B_SPLINE_CURVE((1.,1.00033025159291,1.))
REPRESENTATION_ITEM('')
);
#1899=(
BOUNDED_CURVE()
B_SPLINE_CURVE(2,(#84389,#84390,#84391),.UNSPECIFIED.,.F.,.F.)
B_SPLINE_CURVE_WITH_KNOTS((3,3),(0.,0.0849403543350618),.UNSPECIFIED.)
CURVE()
GEOMETRIC_REPRESENTATION_ITEM()
RATIONAL_B_SPLINE_CURVE((1.,1.00033025329707,1.))
REPRESENTATION_ITEM('')
);
#1900=(
BOUNDED_CURVE()
B_SPLINE_CURVE(2,(#84395,#84396,#84397),.UNSPECIFIED.,.F.,.F.)
B_SPLINE_CURVE_WITH_KNOTS((3,3),(0.,0.0849403543350619),.UNSPECIFIED.)
CURVE()
GEOMETRIC_REPRESENTATION_ITEM()
RATIONAL_B_SPLINE_CURVE((1.,1.00033025019522,1.))
REPRESENTATION_ITEM('')
);
#1901=(
BOUNDED_CURVE()
B_SPLINE_CURVE(2,(#84407,#84408,#84409),.UNSPECIFIED.,.F.,.F.)
B_SPLINE_CURVE_WITH_KNOTS((3,3),(0.,0.0849403543350617),.UNSPECIFIED.)
CURVE()
GEOMETRIC_REPRESENTATION_ITEM()
RATIONAL_B_SPLINE_CURVE((1.,1.00033025277557,1.))
REPRESENTATION_ITEM('')
);
#1902=(
BOUNDED_CURVE()
B_SPLINE_CURVE(2,(#84413,#84414,#84415),.UNSPECIFIED.,.F.,.F.)
B_SPLINE_CURVE_WITH_KNOTS((3,3),(0.,0.0849403543350618),.UNSPECIFIED.)
CURVE()
GEOMETRIC_REPRESENTATION_ITEM()
RATIONAL_B_SPLINE_CURVE((1.,1.0003302523686,1.))
REPRESENTATION_ITEM('')
);
#1903=(
BOUNDED_CURVE()
B_SPLINE_CURVE(2,(#84425,#84426,#84427),.UNSPECIFIED.,.F.,.F.)
B_SPLINE_CURVE_WITH_KNOTS((3,3),(0.,0.0849403543350618),.UNSPECIFIED.)
CURVE()
GEOMETRIC_REPRESENTATION_ITEM()
RATIONAL_B_SPLINE_CURVE((1.,1.00033025290925,1.))
REPRESENTATION_ITEM('')
);
#1904=(
BOUNDED_CURVE()
B_SPLINE_CURVE(2,(#84431,#84432,#84433),.UNSPECIFIED.,.F.,.F.)
B_SPLINE_CURVE_WITH_KNOTS((3,3),(0.,0.0849403543350617),.UNSPECIFIED.)
CURVE()
GEOMETRIC_REPRESENTATION_ITEM()
RATIONAL_B_SPLINE_CURVE((1.,1.00033025137531,1.))
REPRESENTATION_ITEM('')
);
#1905=(
BOUNDED_CURVE()
B_SPLINE_CURVE(2,(#84443,#84444,#84445),.UNSPECIFIED.,.F.,.F.)
B_SPLINE_CURVE_WITH_KNOTS((3,3),(0.,0.0849403543350617),.UNSPECIFIED.)
CURVE()
GEOMETRIC_REPRESENTATION_ITEM()
RATIONAL_B_SPLINE_CURVE((1.,1.00033025135055,1.))
REPRESENTATION_ITEM('')
);
#1906=(
BOUNDED_CURVE()
B_SPLINE_CURVE(2,(#84449,#84450,#84451),.UNSPECIFIED.,.F.,.F.)
B_SPLINE_CURVE_WITH_KNOTS((3,3),(0.,0.0849403543350615),.UNSPECIFIED.)
CURVE()
GEOMETRIC_REPRESENTATION_ITEM()
RATIONAL_B_SPLINE_CURVE((1.,1.00033025140385,1.))
REPRESENTATION_ITEM('')
);
#1907=(
BOUNDED_CURVE()
B_SPLINE_CURVE(2,(#84461,#84462,#84463),.UNSPECIFIED.,.F.,.F.)
B_SPLINE_CURVE_WITH_KNOTS((3,3),(0.,0.0849403543350617),.UNSPECIFIED.)
CURVE()
GEOMETRIC_REPRESENTATION_ITEM()
RATIONAL_B_SPLINE_CURVE((1.,1.00033025153413,1.))
REPRESENTATION_ITEM('')
);
#1908=(
BOUNDED_CURVE()
B_SPLINE_CURVE(2,(#84467,#84468,#84469),.UNSPECIFIED.,.F.,.F.)
B_SPLINE_CURVE_WITH_KNOTS((3,3),(0.,0.0849403543350615),.UNSPECIFIED.)
CURVE()
GEOMETRIC_REPRESENTATION_ITEM()
RATIONAL_B_SPLINE_CURVE((1.,1.00033025092142,1.))
REPRESENTATION_ITEM('')
);
#1909=(
BOUNDED_CURVE()
B_SPLINE_CURVE(2,(#84479,#84480,#84481),.UNSPECIFIED.,.F.,.F.)
B_SPLINE_CURVE_WITH_KNOTS((3,3),(0.,0.0849403543350618),.UNSPECIFIED.)
CURVE()
GEOMETRIC_REPRESENTATION_ITEM()
RATIONAL_B_SPLINE_CURVE((1.,1.000330251177,1.))
REPRESENTATION_ITEM('')
);
#1910=(
BOUNDED_CURVE()
B_SPLINE_CURVE(2,(#84485,#84486,#84487),.UNSPECIFIED.,.F.,.F.)
B_SPLINE_CURVE_WITH_KNOTS((3,3),(0.,0.0849403543350618),.UNSPECIFIED.)
CURVE()
GEOMETRIC_REPRESENTATION_ITEM()
RATIONAL_B_SPLINE_CURVE((1.,1.00033025300405,1.))
REPRESENTATION_ITEM('')
);
#1911=(
BOUNDED_CURVE()
B_SPLINE_CURVE(2,(#84497,#84498,#84499),.UNSPECIFIED.,.F.,.F.)
B_SPLINE_CURVE_WITH_KNOTS((3,3),(0.,0.0849403543350618),.UNSPECIFIED.)
CURVE()
GEOMETRIC_REPRESENTATION_ITEM()
RATIONAL_B_SPLINE_CURVE((1.,1.00033025163674,1.))
REPRESENTATION_ITEM('')
);
#1912=(
BOUNDED_CURVE()
B_SPLINE_CURVE(2,(#84503,#84504,#84505),.UNSPECIFIED.,.F.,.F.)
B_SPLINE_CURVE_WITH_KNOTS((3,3),(0.,0.0849403543350619),.UNSPECIFIED.)
CURVE()
GEOMETRIC_REPRESENTATION_ITEM()
RATIONAL_B_SPLINE_CURVE((1.,1.00033025048646,1.))
REPRESENTATION_ITEM('')
);
#1913=(
BOUNDED_CURVE()
B_SPLINE_CURVE(2,(#84515,#84516,#84517),.UNSPECIFIED.,.F.,.F.)
B_SPLINE_CURVE_WITH_KNOTS((3,3),(0.,0.0849403543350617),.UNSPECIFIED.)
CURVE()
GEOMETRIC_REPRESENTATION_ITEM()
RATIONAL_B_SPLINE_CURVE((1.,1.00033025119026,1.))
REPRESENTATION_ITEM('')
);
#1914=(
BOUNDED_CURVE()
B_SPLINE_CURVE(2,(#84521,#84522,#84523),.UNSPECIFIED.,.F.,.F.)
B_SPLINE_CURVE_WITH_KNOTS((3,3),(0.,0.0849403543350617),.UNSPECIFIED.)
CURVE()
GEOMETRIC_REPRESENTATION_ITEM()
RATIONAL_B_SPLINE_CURVE((1.,1.00033025150196,1.))
REPRESENTATION_ITEM('')
);
#1915=(
BOUNDED_CURVE()
B_SPLINE_CURVE(2,(#84533,#84534,#84535),.UNSPECIFIED.,.F.,.F.)
B_SPLINE_CURVE_WITH_KNOTS((3,3),(0.,0.0849403543350618),.UNSPECIFIED.)
CURVE()
GEOMETRIC_REPRESENTATION_ITEM()
RATIONAL_B_SPLINE_CURVE((1.,1.00033025273958,1.))
REPRESENTATION_ITEM('')
);
#1916=(
BOUNDED_CURVE()
B_SPLINE_CURVE(2,(#84539,#84540,#84541),.UNSPECIFIED.,.F.,.F.)
B_SPLINE_CURVE_WITH_KNOTS((3,3),(0.,0.0849403543350617),.UNSPECIFIED.)
CURVE()
GEOMETRIC_REPRESENTATION_ITEM()
RATIONAL_B_SPLINE_CURVE((1.,1.00033025172765,1.))
REPRESENTATION_ITEM('')
);
#1917=(
BOUNDED_CURVE()
B_SPLINE_CURVE(2,(#84551,#84552,#84553),.UNSPECIFIED.,.F.,.F.)
B_SPLINE_CURVE_WITH_KNOTS((3,3),(0.,0.0849403543350618),.UNSPECIFIED.)
CURVE()
GEOMETRIC_REPRESENTATION_ITEM()
RATIONAL_B_SPLINE_CURVE((1.,1.00033025171672,1.))
REPRESENTATION_ITEM('')
);
#1918=(
BOUNDED_CURVE()
B_SPLINE_CURVE(2,(#84557,#84558,#84559),.UNSPECIFIED.,.F.,.F.)
B_SPLINE_CURVE_WITH_KNOTS((3,3),(0.,0.0849403543350615),.UNSPECIFIED.)
CURVE()
GEOMETRIC_REPRESENTATION_ITEM()
RATIONAL_B_SPLINE_CURVE((1.,1.00033025219597,1.))
REPRESENTATION_ITEM('')
);
#1919=(
BOUNDED_CURVE()
B_SPLINE_CURVE(2,(#84569,#84570,#84571),.UNSPECIFIED.,.F.,.F.)
B_SPLINE_CURVE_WITH_KNOTS((3,3),(0.,0.0849403543350617),.UNSPECIFIED.)
CURVE()
GEOMETRIC_REPRESENTATION_ITEM()
RATIONAL_B_SPLINE_CURVE((1.,1.00033025202292,1.))
REPRESENTATION_ITEM('')
);
#1920=(
BOUNDED_CURVE()
B_SPLINE_CURVE(2,(#84575,#84576,#84577),.UNSPECIFIED.,.F.,.F.)
B_SPLINE_CURVE_WITH_KNOTS((3,3),(0.,0.0849403543350616),.UNSPECIFIED.)
CURVE()
GEOMETRIC_REPRESENTATION_ITEM()
RATIONAL_B_SPLINE_CURVE((1.,1.00033025287801,1.))
REPRESENTATION_ITEM('')
);
#1921=(
BOUNDED_CURVE()
B_SPLINE_CURVE(2,(#84587,#84588,#84589),.UNSPECIFIED.,.F.,.F.)
B_SPLINE_CURVE_WITH_KNOTS((3,3),(0.,0.0849403543350616),.UNSPECIFIED.)
CURVE()
GEOMETRIC_REPRESENTATION_ITEM()
RATIONAL_B_SPLINE_CURVE((1.,1.00033025091841,1.))
REPRESENTATION_ITEM('')
);
#1922=(
BOUNDED_CURVE()
B_SPLINE_CURVE(2,(#84593,#84594,#84595),.UNSPECIFIED.,.F.,.F.)
B_SPLINE_CURVE_WITH_KNOTS((3,3),(0.,0.0849403543350617),.UNSPECIFIED.)
CURVE()
GEOMETRIC_REPRESENTATION_ITEM()
RATIONAL_B_SPLINE_CURVE((1.,1.00033025267027,1.))
REPRESENTATION_ITEM('')
);
#1923=(
BOUNDED_CURVE()
B_SPLINE_CURVE(2,(#84605,#84606,#84607),.UNSPECIFIED.,.F.,.F.)
B_SPLINE_CURVE_WITH_KNOTS((3,3),(0.,0.0849403543350617),.UNSPECIFIED.)
CURVE()
GEOMETRIC_REPRESENTATION_ITEM()
RATIONAL_B_SPLINE_CURVE((1.,1.00033025267027,1.))
REPRESENTATION_ITEM('')
);
#1924=(
BOUNDED_CURVE()
B_SPLINE_CURVE(2,(#84611,#84612,#84613),.UNSPECIFIED.,.F.,.F.)
B_SPLINE_CURVE_WITH_KNOTS((3,3),(0.,0.0849403543350618),.UNSPECIFIED.)
CURVE()
GEOMETRIC_REPRESENTATION_ITEM()
RATIONAL_B_SPLINE_CURVE((1.,1.00033025117682,1.))
REPRESENTATION_ITEM('')
);
#1925=(
BOUNDED_CURVE()
B_SPLINE_CURVE(2,(#84623,#84624,#84625),.UNSPECIFIED.,.F.,.F.)
B_SPLINE_CURVE_WITH_KNOTS((3,3),(0.,0.0849403543350617),.UNSPECIFIED.)
CURVE()
GEOMETRIC_REPRESENTATION_ITEM()
RATIONAL_B_SPLINE_CURVE((1.,1.00033025218034,1.))
REPRESENTATION_ITEM('')
);
#1926=(
BOUNDED_CURVE()
B_SPLINE_CURVE(2,(#84629,#84630,#84631),.UNSPECIFIED.,.F.,.F.)
B_SPLINE_CURVE_WITH_KNOTS((3,3),(0.,0.0849403543350617),.UNSPECIFIED.)
CURVE()
GEOMETRIC_REPRESENTATION_ITEM()
RATIONAL_B_SPLINE_CURVE((1.,1.00033025187435,1.))
REPRESENTATION_ITEM('')
);
#1927=(
BOUNDED_CURVE()
B_SPLINE_CURVE(2,(#84641,#84642,#84643),.UNSPECIFIED.,.F.,.F.)
B_SPLINE_CURVE_WITH_KNOTS((3,3),(0.,0.0849403543350617),.UNSPECIFIED.)
CURVE()
GEOMETRIC_REPRESENTATION_ITEM()
RATIONAL_B_SPLINE_CURVE((1.,1.00033025297806,1.))
REPRESENTATION_ITEM('')
);
#1928=(
BOUNDED_CURVE()
B_SPLINE_CURVE(2,(#84647,#84648,#84649),.UNSPECIFIED.,.F.,.F.)
B_SPLINE_CURVE_WITH_KNOTS((3,3),(0.,0.0849403543350617),.UNSPECIFIED.)
CURVE()
GEOMETRIC_REPRESENTATION_ITEM()
RATIONAL_B_SPLINE_CURVE((1.,1.00033025136034,1.))
REPRESENTATION_ITEM('')
);
#3829=FACE_OUTER_BOUND('',#6259,.T.);
#3830=FACE_OUTER_BOUND('',#6260,.T.);
#3831=FACE_OUTER_BOUND('',#6261,.T.);
#3832=FACE_OUTER_BOUND('',#6262,.T.);
#3833=FACE_OUTER_BOUND('',#6263,.T.);
#3834=FACE_OUTER_BOUND('',#6264,.T.);
#3835=FACE_OUTER_BOUND('',#6265,.T.);
#3836=FACE_OUTER_BOUND('',#6266,.T.);
#3837=FACE_OUTER_BOUND('',#6267,.T.);
#3838=FACE_OUTER_BOUND('',#6268,.T.);
#3839=FACE_OUTER_BOUND('',#6269,.T.);
#3840=FACE_OUTER_BOUND('',#6270,.T.);
#3841=FACE_OUTER_BOUND('',#6271,.T.);
#3842=FACE_OUTER_BOUND('',#6272,.T.);
#3843=FACE_OUTER_BOUND('',#6273,.T.);
#3844=FACE_OUTER_BOUND('',#6274,.T.);
#3845=FACE_OUTER_BOUND('',#6275,.T.);
#3846=FACE_OUTER_BOUND('',#6276,.T.);
#3847=FACE_OUTER_BOUND('',#6277,.T.);
#3848=FACE_OUTER_BOUND('',#6278,.T.);
#3849=FACE_OUTER_BOUND('',#6279,.T.);
#3850=FACE_OUTER_BOUND('',#6280,.T.);
#3851=FACE_OUTER_BOUND('',#6281,.T.);
#3852=FACE_OUTER_BOUND('',#6282,.T.);
#3853=FACE_OUTER_BOUND('',#6283,.T.);
#3854=FACE_OUTER_BOUND('',#6284,.T.);
#3855=FACE_OUTER_BOUND('',#6285,.T.);
#3856=FACE_OUTER_BOUND('',#6286,.T.);
#3857=FACE_OUTER_BOUND('',#6287,.T.);
#3858=FACE_OUTER_BOUND('',#6288,.T.);
#3859=FACE_OUTER_BOUND('',#6289,.T.);
#3860=FACE_OUTER_BOUND('',#6290,.T.);
#3861=FACE_OUTER_BOUND('',#6291,.T.);
#3862=FACE_OUTER_BOUND('',#6292,.T.);
#3863=FACE_OUTER_BOUND('',#6293,.T.);
#3864=FACE_OUTER_BOUND('',#6294,.T.);
#3865=FACE_OUTER_BOUND('',#6295,.T.);
#3866=FACE_OUTER_BOUND('',#6296,.T.);
#3867=FACE_OUTER_BOUND('',#6297,.T.);
#3868=FACE_OUTER_BOUND('',#6298,.T.);
#3869=FACE_OUTER_BOUND('',#6299,.T.);
#3870=FACE_OUTER_BOUND('',#6300,.T.);
#3871=FACE_OUTER_BOUND('',#6301,.T.);
#3872=FACE_OUTER_BOUND('',#6302,.T.);
#3873=FACE_OUTER_BOUND('',#6303,.T.);
#3874=FACE_OUTER_BOUND('',#6304,.T.);
#3875=FACE_OUTER_BOUND('',#6305,.T.);
#3876=FACE_OUTER_BOUND('',#6306,.T.);
#3877=FACE_OUTER_BOUND('',#6307,.T.);
#3878=FACE_OUTER_BOUND('',#6308,.T.);
#3879=FACE_OUTER_BOUND('',#6309,.T.);
#3880=FACE_OUTER_BOUND('',#6310,.T.);
#3881=FACE_OUTER_BOUND('',#6311,.T.);
#3882=FACE_OUTER_BOUND('',#6312,.T.);
#3883=FACE_OUTER_BOUND('',#6313,.T.);
#3884=FACE_OUTER_BOUND('',#6314,.T.);
#3885=FACE_OUTER_BOUND('',#6315,.T.);
#3886=FACE_OUTER_BOUND('',#6316,.T.);
#3887=FACE_OUTER_BOUND('',#6317,.T.);
#3888=FACE_OUTER_BOUND('',#6318,.T.);
#3889=FACE_OUTER_BOUND('',#6319,.T.);
#3890=FACE_OUTER_BOUND('',#6320,.T.);
#3891=FACE_OUTER_BOUND('',#6321,.T.);
#3892=FACE_OUTER_BOUND('',#6322,.T.);
#3893=FACE_OUTER_BOUND('',#6323,.T.);
#3894=FACE_OUTER_BOUND('',#6324,.T.);
#3895=FACE_OUTER_BOUND('',#6325,.T.);
#3896=FACE_OUTER_BOUND('',#6326,.T.);
#3897=FACE_OUTER_BOUND('',#6327,.T.);
#3898=FACE_OUTER_BOUND('',#6328,.T.);
#3899=FACE_OUTER_BOUND('',#6329,.T.);
#3900=FACE_OUTER_BOUND('',#6330,.T.);
#3901=FACE_OUTER_BOUND('',#6331,.T.);
#3902=FACE_OUTER_BOUND('',#6332,.T.);
#3903=FACE_OUTER_BOUND('',#6333,.T.);
#3904=FACE_OUTER_BOUND('',#6334,.T.);
#3905=FACE_OUTER_BOUND('',#6335,.T.);
#3906=FACE_OUTER_BOUND('',#6336,.T.);
#3907=FACE_OUTER_BOUND('',#6337,.T.);
#3908=FACE_OUTER_BOUND('',#6338,.T.);
#3909=FACE_OUTER_BOUND('',#6339,.T.);
#3910=FACE_OUTER_BOUND('',#6340,.T.);
#3911=FACE_OUTER_BOUND('',#6341,.T.);
#3912=FACE_OUTER_BOUND('',#6342,.T.);
#3913=FACE_OUTER_BOUND('',#6343,.T.);
#3914=FACE_OUTER_BOUND('',#6344,.T.);
#3915=FACE_OUTER_BOUND('',#6345,.T.);
#3916=FACE_OUTER_BOUND('',#6346,.T.);
#3917=FACE_OUTER_BOUND('',#6347,.T.);
#3918=FACE_OUTER_BOUND('',#6348,.T.);
#3919=FACE_OUTER_BOUND('',#6349,.T.);
#3920=FACE_OUTER_BOUND('',#6350,.T.);
#3921=FACE_OUTER_BOUND('',#6351,.T.);
#3922=FACE_OUTER_BOUND('',#6352,.T.);
#3923=FACE_OUTER_BOUND('',#6353,.T.);
#3924=FACE_OUTER_BOUND('',#6354,.T.);
#3925=FACE_OUTER_BOUND('',#6355,.T.);
#3926=FACE_OUTER_BOUND('',#6356,.T.);
#3927=FACE_OUTER_BOUND('',#6357,.T.);
#3928=FACE_OUTER_BOUND('',#6358,.T.);
#3929=FACE_OUTER_BOUND('',#6359,.T.);
#3930=FACE_OUTER_BOUND('',#6360,.T.);
#3931=FACE_OUTER_BOUND('',#6361,.T.);
#3932=FACE_OUTER_BOUND('',#6362,.T.);
#3933=FACE_OUTER_BOUND('',#6363,.T.);
#3934=FACE_OUTER_BOUND('',#6364,.T.);
#3935=FACE_OUTER_BOUND('',#6365,.T.);
#3936=FACE_OUTER_BOUND('',#6366,.T.);
#3937=FACE_OUTER_BOUND('',#6367,.T.);
#3938=FACE_OUTER_BOUND('',#6368,.T.);
#3939=FACE_OUTER_BOUND('',#6369,.T.);
#3940=FACE_OUTER_BOUND('',#6370,.T.);
#3941=FACE_OUTER_BOUND('',#6371,.T.);
#3942=FACE_OUTER_BOUND('',#6372,.T.);
#3943=FACE_OUTER_BOUND('',#6373,.T.);
#3944=FACE_OUTER_BOUND('',#6374,.T.);
#3945=FACE_OUTER_BOUND('',#6375,.T.);
#3946=FACE_OUTER_BOUND('',#6376,.T.);
#3947=FACE_OUTER_BOUND('',#6377,.T.);
#3948=FACE_OUTER_BOUND('',#6378,.T.);
#3949=FACE_OUTER_BOUND('',#6379,.T.);
#3950=FACE_OUTER_BOUND('',#6380,.T.);
#3951=FACE_OUTER_BOUND('',#6381,.T.);
#3952=FACE_OUTER_BOUND('',#6382,.T.);
#3953=FACE_OUTER_BOUND('',#6383,.T.);
#3954=FACE_OUTER_BOUND('',#6384,.T.);
#3955=FACE_OUTER_BOUND('',#6385,.T.);
#3956=FACE_OUTER_BOUND('',#6386,.T.);
#3957=FACE_OUTER_BOUND('',#6387,.T.);
#3958=FACE_OUTER_BOUND('',#6388,.T.);
#3959=FACE_OUTER_BOUND('',#6389,.T.);
#3960=FACE_OUTER_BOUND('',#6390,.T.);
#3961=FACE_OUTER_BOUND('',#6391,.T.);
#3962=FACE_OUTER_BOUND('',#6392,.T.);
#3963=FACE_OUTER_BOUND('',#6393,.T.);
#3964=FACE_OUTER_BOUND('',#6394,.T.);
#3965=FACE_OUTER_BOUND('',#6395,.T.);
#3966=FACE_OUTER_BOUND('',#6396,.T.);
#3967=FACE_OUTER_BOUND('',#6397,.T.);
#3968=FACE_OUTER_BOUND('',#6398,.T.);
#3969=FACE_OUTER_BOUND('',#6399,.T.);
#3970=FACE_OUTER_BOUND('',#6400,.T.);
#3971=FACE_OUTER_BOUND('',#6401,.T.);
#3972=FACE_OUTER_BOUND('',#6402,.T.);
#3973=FACE_OUTER_BOUND('',#6403,.T.);
#3974=FACE_OUTER_BOUND('',#6404,.T.);
#3975=FACE_OUTER_BOUND('',#6405,.T.);
#3976=FACE_OUTER_BOUND('',#6406,.T.);
#3977=FACE_OUTER_BOUND('',#6407,.T.);
#3978=FACE_OUTER_BOUND('',#6408,.T.);
#3979=FACE_OUTER_BOUND('',#6409,.T.);
#3980=FACE_OUTER_BOUND('',#6410,.T.);
#3981=FACE_OUTER_BOUND('',#6411,.T.);
#3982=FACE_OUTER_BOUND('',#6412,.T.);
#3983=FACE_OUTER_BOUND('',#6413,.T.);
#3984=FACE_OUTER_BOUND('',#6414,.T.);
#3985=FACE_OUTER_BOUND('',#6415,.T.);
#3986=FACE_OUTER_BOUND('',#6416,.T.);
#3987=FACE_OUTER_BOUND('',#6417,.T.);
#3988=FACE_OUTER_BOUND('',#6418,.T.);
#3989=FACE_OUTER_BOUND('',#6419,.T.);
#3990=FACE_OUTER_BOUND('',#6420,.T.);
#3991=FACE_OUTER_BOUND('',#6421,.T.);
#3992=FACE_OUTER_BOUND('',#6422,.T.);
#3993=FACE_OUTER_BOUND('',#6423,.T.);
#3994=FACE_OUTER_BOUND('',#6424,.T.);
#3995=FACE_OUTER_BOUND('',#6425,.T.);
#3996=FACE_OUTER_BOUND('',#6426,.T.);
#3997=FACE_OUTER_BOUND('',#6427,.T.);
#3998=FACE_OUTER_BOUND('',#6428,.T.);
#3999=FACE_OUTER_BOUND('',#6429,.T.);
#4000=FACE_OUTER_BOUND('',#6430,.T.);
#4001=FACE_OUTER_BOUND('',#6431,.T.);
#4002=FACE_OUTER_BOUND('',#6432,.T.);
#4003=FACE_OUTER_BOUND('',#6433,.T.);
#4004=FACE_OUTER_BOUND('',#6434,.T.);
#4005=FACE_OUTER_BOUND('',#6435,.T.);
#4006=FACE_OUTER_BOUND('',#6436,.T.);
#4007=FACE_OUTER_BOUND('',#6437,.T.);
#4008=FACE_OUTER_BOUND('',#6438,.T.);
#4009=FACE_OUTER_BOUND('',#6439,.T.);
#4010=FACE_OUTER_BOUND('',#6440,.T.);
#4011=FACE_OUTER_BOUND('',#6441,.T.);
#4012=FACE_OUTER_BOUND('',#6442,.T.);
#4013=FACE_OUTER_BOUND('',#6443,.T.);
#4014=FACE_OUTER_BOUND('',#6444,.T.);
#4015=FACE_OUTER_BOUND('',#6445,.T.);
#4016=FACE_OUTER_BOUND('',#6446,.T.);
#4017=FACE_OUTER_BOUND('',#6447,.T.);
#4018=FACE_OUTER_BOUND('',#6448,.T.);
#4019=FACE_OUTER_BOUND('',#6449,.T.);
#4020=FACE_OUTER_BOUND('',#6450,.T.);
#4021=FACE_OUTER_BOUND('',#6451,.T.);
#4022=FACE_OUTER_BOUND('',#6452,.T.);
#4023=FACE_OUTER_BOUND('',#6453,.T.);
#4024=FACE_OUTER_BOUND('',#6454,.T.);
#4025=FACE_OUTER_BOUND('',#6455,.T.);
#4026=FACE_OUTER_BOUND('',#6456,.T.);
#4027=FACE_OUTER_BOUND('',#6457,.T.);
#4028=FACE_OUTER_BOUND('',#6458,.T.);
#4029=FACE_OUTER_BOUND('',#6459,.T.);
#4030=FACE_OUTER_BOUND('',#6460,.T.);
#4031=FACE_OUTER_BOUND('',#6461,.T.);
#4032=FACE_OUTER_BOUND('',#6462,.T.);
#4033=FACE_OUTER_BOUND('',#6463,.T.);
#4034=FACE_OUTER_BOUND('',#6464,.T.);
#4035=FACE_OUTER_BOUND('',#6465,.T.);
#4036=FACE_OUTER_BOUND('',#6466,.T.);
#4037=FACE_OUTER_BOUND('',#6467,.T.);
#4038=FACE_OUTER_BOUND('',#6468,.T.);
#4039=FACE_OUTER_BOUND('',#6469,.T.);
#4040=FACE_OUTER_BOUND('',#6470,.T.);
#4041=FACE_OUTER_BOUND('',#6471,.T.);
#4042=FACE_OUTER_BOUND('',#6472,.T.);
#4043=FACE_OUTER_BOUND('',#6473,.T.);
#4044=FACE_OUTER_BOUND('',#6474,.T.);
#4045=FACE_OUTER_BOUND('',#6475,.T.);
#4046=FACE_OUTER_BOUND('',#6476,.T.);
#4047=FACE_OUTER_BOUND('',#6477,.T.);
#4048=FACE_OUTER_BOUND('',#6478,.T.);
#4049=FACE_OUTER_BOUND('',#6479,.T.);
#4050=FACE_OUTER_BOUND('',#6480,.T.);
#4051=FACE_OUTER_BOUND('',#6481,.T.);
#4052=FACE_OUTER_BOUND('',#6482,.T.);
#4053=FACE_OUTER_BOUND('',#6483,.T.);
#4054=FACE_OUTER_BOUND('',#6484,.T.);
#4055=FACE_OUTER_BOUND('',#6485,.T.);
#4056=FACE_OUTER_BOUND('',#6486,.T.);
#4057=FACE_OUTER_BOUND('',#6487,.T.);
#4058=FACE_OUTER_BOUND('',#6488,.T.);
#4059=FACE_OUTER_BOUND('',#6489,.T.);
#4060=FACE_OUTER_BOUND('',#6490,.T.);
#4061=FACE_OUTER_BOUND('',#6491,.T.);
#4062=FACE_OUTER_BOUND('',#6492,.T.);
#4063=FACE_OUTER_BOUND('',#6493,.T.);
#4064=FACE_OUTER_BOUND('',#6494,.T.);
#4065=FACE_OUTER_BOUND('',#6495,.T.);
#4066=FACE_OUTER_BOUND('',#6496,.T.);
#4067=FACE_OUTER_BOUND('',#6497,.T.);
#4068=FACE_OUTER_BOUND('',#6498,.T.);
#4069=FACE_OUTER_BOUND('',#6499,.T.);
#4070=FACE_OUTER_BOUND('',#6500,.T.);
#4071=FACE_OUTER_BOUND('',#6501,.T.);
#6259=EDGE_LOOP('',(#33351,#33352,#33353,#33354,#33355));
#6260=EDGE_LOOP('',(#33356,#33357,#33358,#33359));
#6261=EDGE_LOOP('',(#33360,#33361,#33362,#33363,#33364));
#6262=EDGE_LOOP('',(#33365,#33366,#33367,#33368));
#6263=EDGE_LOOP('',(#33369,#33370,#33371,#33372,#33373,#33374,#33375,#33376,
#33377,#33378,#33379,#33380,#33381,#33382,#33383,#33384,#33385,#33386,#33387,
#33388,#33389,#33390,#33391,#33392,#33393,#33394,#33395,#33396,#33397,#33398,
#33399,#33400,#33401,#33402,#33403,#33404,#33405,#33406,#33407,#33408,#33409,
#33410,#33411,#33412,#33413,#33414,#33415,#33416,#33417,#33418,#33419,#33420,
#33421,#33422,#33423,#33424,#33425,#33426,#33427,#33428,#33429,#33430,#33431,
#33432,#33433,#33434,#33435,#33436,#33437,#33438,#33439,#33440,#33441,#33442,
#33443,#33444,#33445,#33446,#33447,#33448,#33449,#33450,#33451,#33452,#33453,
#33454,#33455,#33456,#33457,#33458,#33459,#33460,#33461,#33462,#33463,#33464,
#33465,#33466,#33467,#33468,#33469,#33470,#33471,#33472,#33473,#33474,#33475,
#33476,#33477,#33478,#33479,#33480,#33481,#33482,#33483,#33484,#33485,#33486,
#33487,#33488,#33489,#33490,#33491,#33492,#33493,#33494,#33495,#33496,#33497,
#33498,#33499,#33500,#33501,#33502,#33503,#33504,#33505,#33506,#33507,#33508,
#33509,#33510,#33511,#33512,#33513,#33514,#33515,#33516,#33517,#33518,#33519,
#33520,#33521,#33522,#33523,#33524,#33525,#33526,#33527,#33528,#33529,#33530,
#33531,#33532,#33533,#33534,#33535,#33536,#33537,#33538,#33539,#33540,#33541,
#33542,#33543,#33544,#33545,#33546,#33547,#33548,#33549,#33550,#33551,#33552,
#33553,#33554,#33555,#33556,#33557,#33558,#33559,#33560,#33561,#33562,#33563,
#33564));
#6264=EDGE_LOOP('',(#33565,#33566,#33567,#33568));
#6265=EDGE_LOOP('',(#33569,#33570,#33571,#33572));
#6266=EDGE_LOOP('',(#33573,#33574,#33575,#33576,#33577));
#6267=EDGE_LOOP('',(#33578,#33579,#33580,#33581));
#6268=EDGE_LOOP('',(#33582,#33583,#33584,#33585,#33586));
#6269=EDGE_LOOP('',(#33587,#33588,#33589,#33590));
#6270=EDGE_LOOP('',(#33591,#33592,#33593,#33594));
#6271=EDGE_LOOP('',(#33595,#33596,#33597,#33598,#33599));
#6272=EDGE_LOOP('',(#33600,#33601,#33602,#33603));
#6273=EDGE_LOOP('',(#33604,#33605,#33606,#33607,#33608));
#6274=EDGE_LOOP('',(#33609,#33610,#33611,#33612));
#6275=EDGE_LOOP('',(#33613,#33614,#33615,#33616));
#6276=EDGE_LOOP('',(#33617,#33618,#33619,#33620,#33621));
#6277=EDGE_LOOP('',(#33622,#33623,#33624,#33625));
#6278=EDGE_LOOP('',(#33626,#33627,#33628,#33629,#33630));
#6279=EDGE_LOOP('',(#33631,#33632,#33633,#33634));
#6280=EDGE_LOOP('',(#33635,#33636,#33637,#33638));
#6281=EDGE_LOOP('',(#33639,#33640,#33641,#33642,#33643));
#6282=EDGE_LOOP('',(#33644,#33645,#33646,#33647));
#6283=EDGE_LOOP('',(#33648,#33649,#33650,#33651,#33652));
#6284=EDGE_LOOP('',(#33653,#33654,#33655,#33656));
#6285=EDGE_LOOP('',(#33657,#33658,#33659,#33660));
#6286=EDGE_LOOP('',(#33661,#33662,#33663,#33664,#33665));
#6287=EDGE_LOOP('',(#33666,#33667,#33668,#33669));
#6288=EDGE_LOOP('',(#33670,#33671,#33672,#33673,#33674));
#6289=EDGE_LOOP('',(#33675,#33676,#33677,#33678));
#6290=EDGE_LOOP('',(#33679,#33680,#33681,#33682));
#6291=EDGE_LOOP('',(#33683,#33684,#33685,#33686,#33687));
#6292=EDGE_LOOP('',(#33688,#33689,#33690,#33691));
#6293=EDGE_LOOP('',(#33692,#33693,#33694,#33695,#33696));
#6294=EDGE_LOOP('',(#33697,#33698,#33699,#33700));
#6295=EDGE_LOOP('',(#33701,#33702,#33703,#33704));
#6296=EDGE_LOOP('',(#33705,#33706,#33707,#33708,#33709));
#6297=EDGE_LOOP('',(#33710,#33711,#33712,#33713));
#6298=EDGE_LOOP('',(#33714,#33715,#33716,#33717,#33718));
#6299=EDGE_LOOP('',(#33719,#33720,#33721,#33722));
#6300=EDGE_LOOP('',(#33723,#33724,#33725,#33726));
#6301=EDGE_LOOP('',(#33727,#33728,#33729,#33730,#33731));
#6302=EDGE_LOOP('',(#33732,#33733,#33734,#33735));
#6303=EDGE_LOOP('',(#33736,#33737,#33738,#33739,#33740));
#6304=EDGE_LOOP('',(#33741,#33742,#33743,#33744));
#6305=EDGE_LOOP('',(#33745,#33746,#33747,#33748));
#6306=EDGE_LOOP('',(#33749,#33750,#33751,#33752,#33753));
#6307=EDGE_LOOP('',(#33754,#33755,#33756,#33757));
#6308=EDGE_LOOP('',(#33758,#33759,#33760,#33761,#33762));
#6309=EDGE_LOOP('',(#33763,#33764,#33765,#33766));
#6310=EDGE_LOOP('',(#33767,#33768,#33769,#33770));
#6311=EDGE_LOOP('',(#33771,#33772,#33773,#33774,#33775));
#6312=EDGE_LOOP('',(#33776,#33777,#33778,#33779));
#6313=EDGE_LOOP('',(#33780,#33781,#33782,#33783,#33784));
#6314=EDGE_LOOP('',(#33785,#33786,#33787,#33788));
#6315=EDGE_LOOP('',(#33789,#33790,#33791,#33792));
#6316=EDGE_LOOP('',(#33793,#33794,#33795,#33796,#33797));
#6317=EDGE_LOOP('',(#33798,#33799,#33800,#33801,#33802));
#6318=EDGE_LOOP('',(#33803,#33804,#33805,#33806,#33807));
#6319=EDGE_LOOP('',(#33808,#33809,#33810,#33811));
#6320=EDGE_LOOP('',(#33812,#33813,#33814,#33815));
#6321=EDGE_LOOP('',(#33816,#33817,#33818,#33819,#33820));
#6322=EDGE_LOOP('',(#33821,#33822,#33823,#33824));
#6323=EDGE_LOOP('',(#33825,#33826,#33827,#33828,#33829));
#6324=EDGE_LOOP('',(#33830,#33831,#33832,#33833));
#6325=EDGE_LOOP('',(#33834,#33835,#33836,#33837));
#6326=EDGE_LOOP('',(#33838,#33839,#33840,#33841,#33842));
#6327=EDGE_LOOP('',(#33843,#33844,#33845,#33846));
#6328=EDGE_LOOP('',(#33847,#33848,#33849,#33850,#33851));
#6329=EDGE_LOOP('',(#33852,#33853,#33854,#33855));
#6330=EDGE_LOOP('',(#33856,#33857,#33858,#33859));
#6331=EDGE_LOOP('',(#33860,#33861,#33862,#33863,#33864));
#6332=EDGE_LOOP('',(#33865,#33866,#33867,#33868));
#6333=EDGE_LOOP('',(#33869,#33870,#33871,#33872,#33873));
#6334=EDGE_LOOP('',(#33874,#33875,#33876,#33877));
#6335=EDGE_LOOP('',(#33878,#33879,#33880,#33881));
#6336=EDGE_LOOP('',(#33882,#33883,#33884,#33885,#33886));
#6337=EDGE_LOOP('',(#33887,#33888,#33889,#33890));
#6338=EDGE_LOOP('',(#33891,#33892,#33893,#33894,#33895));
#6339=EDGE_LOOP('',(#33896,#33897,#33898,#33899));
#6340=EDGE_LOOP('',(#33900,#33901,#33902,#33903));
#6341=EDGE_LOOP('',(#33904,#33905,#33906,#33907,#33908));
#6342=EDGE_LOOP('',(#33909,#33910,#33911,#33912));
#6343=EDGE_LOOP('',(#33913,#33914,#33915,#33916,#33917));
#6344=EDGE_LOOP('',(#33918,#33919,#33920,#33921));
#6345=EDGE_LOOP('',(#33922,#33923,#33924,#33925));
#6346=EDGE_LOOP('',(#33926,#33927,#33928,#33929,#33930));
#6347=EDGE_LOOP('',(#33931,#33932,#33933,#33934));
#6348=EDGE_LOOP('',(#33935,#33936,#33937,#33938,#33939));
#6349=EDGE_LOOP('',(#33940,#33941,#33942,#33943));
#6350=EDGE_LOOP('',(#33944,#33945,#33946,#33947));
#6351=EDGE_LOOP('',(#33948,#33949,#33950,#33951,#33952));
#6352=EDGE_LOOP('',(#33953,#33954,#33955,#33956));
#6353=EDGE_LOOP('',(#33957,#33958,#33959,#33960,#33961));
#6354=EDGE_LOOP('',(#33962,#33963,#33964,#33965));
#6355=EDGE_LOOP('',(#33966,#33967,#33968,#33969));
#6356=EDGE_LOOP('',(#33970,#33971,#33972,#33973,#33974));
#6357=EDGE_LOOP('',(#33975,#33976,#33977,#33978));
#6358=EDGE_LOOP('',(#33979,#33980,#33981,#33982,#33983));
#6359=EDGE_LOOP('',(#33984,#33985,#33986,#33987));
#6360=EDGE_LOOP('',(#33988,#33989,#33990,#33991));
#6361=EDGE_LOOP('',(#33992,#33993,#33994,#33995,#33996));
#6362=EDGE_LOOP('',(#33997,#33998,#33999,#34000));
#6363=EDGE_LOOP('',(#34001,#34002,#34003,#34004,#34005));
#6364=EDGE_LOOP('',(#34006,#34007,#34008,#34009));
#6365=EDGE_LOOP('',(#34010,#34011,#34012,#34013));
#6366=EDGE_LOOP('',(#34014,#34015,#34016,#34017,#34018));
#6367=EDGE_LOOP('',(#34019,#34020,#34021,#34022));
#6368=EDGE_LOOP('',(#34023,#34024,#34025,#34026,#34027));
#6369=EDGE_LOOP('',(#34028,#34029,#34030,#34031));
#6370=EDGE_LOOP('',(#34032,#34033,#34034,#34035));
#6371=EDGE_LOOP('',(#34036,#34037,#34038,#34039,#34040));
#6372=EDGE_LOOP('',(#34041,#34042,#34043,#34044));
#6373=EDGE_LOOP('',(#34045,#34046,#34047,#34048,#34049));
#6374=EDGE_LOOP('',(#34050,#34051,#34052,#34053));
#6375=EDGE_LOOP('',(#34054,#34055,#34056,#34057));
#6376=EDGE_LOOP('',(#34058,#34059,#34060,#34061,#34062));
#6377=EDGE_LOOP('',(#34063,#34064,#34065,#34066));
#6378=EDGE_LOOP('',(#34067,#34068,#34069,#34070,#34071));
#6379=EDGE_LOOP('',(#34072,#34073,#34074,#34075));
#6380=EDGE_LOOP('',(#34076,#34077,#34078,#34079,#34080));
#6381=EDGE_LOOP('',(#34081,#34082,#34083,#34084));
#6382=EDGE_LOOP('',(#34085,#34086,#34087,#34088,#34089));
#6383=EDGE_LOOP('',(#34090,#34091,#34092,#34093));
#6384=EDGE_LOOP('',(#34094,#34095,#34096,#34097,#34098,#34099,#34100,#34101,
#34102,#34103,#34104,#34105,#34106,#34107,#34108,#34109,#34110,#34111,#34112,
#34113,#34114,#34115,#34116,#34117,#34118,#34119,#34120,#34121,#34122,#34123,
#34124,#34125,#34126,#34127,#34128,#34129,#34130,#34131,#34132,#34133,#34134,
#34135,#34136,#34137,#34138,#34139,#34140,#34141,#34142,#34143,#34144,#34145,
#34146,#34147,#34148,#34149,#34150,#34151,#34152,#34153,#34154,#34155,#34156,
#34157,#34158,#34159,#34160,#34161,#34162,#34163,#34164,#34165,#34166,#34167,
#34168,#34169,#34170,#34171,#34172,#34173,#34174,#34175,#34176,#34177,#34178,
#34179,#34180,#34181,#34182,#34183,#34184,#34185,#34186,#34187,#34188,#34189));
#6385=EDGE_LOOP('',(#34190,#34191,#34192,#34193));
#6386=EDGE_LOOP('',(#34194,#34195,#34196,#34197));
#6387=EDGE_LOOP('',(#34198,#34199,#34200,#34201,#34202));
#6388=EDGE_LOOP('',(#34203,#34204,#34205,#34206));
#6389=EDGE_LOOP('',(#34207,#34208,#34209,#34210,#34211));
#6390=EDGE_LOOP('',(#34212,#34213,#34214,#34215));
#6391=EDGE_LOOP('',(#34216,#34217,#34218,#34219));
#6392=EDGE_LOOP('',(#34220,#34221,#34222,#34223,#34224));
#6393=EDGE_LOOP('',(#34225,#34226,#34227,#34228));
#6394=EDGE_LOOP('',(#34229,#34230,#34231,#34232,#34233));
#6395=EDGE_LOOP('',(#34234,#34235,#34236,#34237));
#6396=EDGE_LOOP('',(#34238,#34239,#34240,#34241));
#6397=EDGE_LOOP('',(#34242,#34243,#34244,#34245,#34246));
#6398=EDGE_LOOP('',(#34247,#34248,#34249,#34250));
#6399=EDGE_LOOP('',(#34251,#34252,#34253,#34254,#34255));
#6400=EDGE_LOOP('',(#34256,#34257,#34258,#34259));
#6401=EDGE_LOOP('',(#34260,#34261,#34262,#34263));
#6402=EDGE_LOOP('',(#34264,#34265,#34266,#34267,#34268));
#6403=EDGE_LOOP('',(#34269,#34270,#34271,#34272));
#6404=EDGE_LOOP('',(#34273,#34274,#34275,#34276,#34277));
#6405=EDGE_LOOP('',(#34278,#34279,#34280,#34281));
#6406=EDGE_LOOP('',(#34282,#34283,#34284,#34285));
#6407=EDGE_LOOP('',(#34286,#34287,#34288,#34289,#34290));
#6408=EDGE_LOOP('',(#34291,#34292,#34293,#34294));
#6409=EDGE_LOOP('',(#34295,#34296,#34297,#34298,#34299));
#6410=EDGE_LOOP('',(#34300,#34301,#34302,#34303));
#6411=EDGE_LOOP('',(#34304,#34305,#34306,#34307));
#6412=EDGE_LOOP('',(#34308,#34309,#34310,#34311,#34312));
#6413=EDGE_LOOP('',(#34313,#34314,#34315,#34316));
#6414=EDGE_LOOP('',(#34317,#34318,#34319,#34320,#34321));
#6415=EDGE_LOOP('',(#34322,#34323,#34324,#34325));
#6416=EDGE_LOOP('',(#34326,#34327,#34328,#34329));
#6417=EDGE_LOOP('',(#34330,#34331,#34332,#34333,#34334));
#6418=EDGE_LOOP('',(#34335,#34336,#34337,#34338));
#6419=EDGE_LOOP('',(#34339,#34340,#34341,#34342,#34343));
#6420=EDGE_LOOP('',(#34344,#34345,#34346,#34347));
#6421=EDGE_LOOP('',(#34348,#34349,#34350,#34351));
#6422=EDGE_LOOP('',(#34352,#34353,#34354,#34355,#34356));
#6423=EDGE_LOOP('',(#34357,#34358,#34359,#34360));
#6424=EDGE_LOOP('',(#34361,#34362,#34363,#34364,#34365));
#6425=EDGE_LOOP('',(#34366,#34367,#34368,#34369));
#6426=EDGE_LOOP('',(#34370,#34371,#34372,#34373));
#6427=EDGE_LOOP('',(#34374,#34375,#34376,#34377,#34378));
#6428=EDGE_LOOP('',(#34379,#34380,#34381,#34382));
#6429=EDGE_LOOP('',(#34383,#34384,#34385,#34386,#34387));
#6430=EDGE_LOOP('',(#34388,#34389,#34390,#34391));
#6431=EDGE_LOOP('',(#34392,#34393,#34394,#34395));
#6432=EDGE_LOOP('',(#34396,#34397,#34398,#34399,#34400));
#6433=EDGE_LOOP('',(#34401,#34402,#34403,#34404));
#6434=EDGE_LOOP('',(#34405,#34406,#34407,#34408,#34409));
#6435=EDGE_LOOP('',(#34410,#34411,#34412,#34413));
#6436=EDGE_LOOP('',(#34414,#34415,#34416,#34417));
#6437=EDGE_LOOP('',(#34418,#34419,#34420,#34421,#34422));
#6438=EDGE_LOOP('',(#34423,#34424,#34425,#34426));
#6439=EDGE_LOOP('',(#34427,#34428,#34429,#34430,#34431));
#6440=EDGE_LOOP('',(#34432,#34433,#34434,#34435,#34436));
#6441=EDGE_LOOP('',(#34437,#34438,#34439,#34440));
#6442=EDGE_LOOP('',(#34441,#34442,#34443,#34444,#34445));
#6443=EDGE_LOOP('',(#34446,#34447,#34448,#34449));
#6444=EDGE_LOOP('',(#34450,#34451,#34452,#34453,#34454));
#6445=EDGE_LOOP('',(#34455,#34456,#34457,#34458));
#6446=EDGE_LOOP('',(#34459,#34460,#34461,#34462));
#6447=EDGE_LOOP('',(#34463,#34464,#34465,#34466,#34467));
#6448=EDGE_LOOP('',(#34468,#34469,#34470,#34471));
#6449=EDGE_LOOP('',(#34472,#34473,#34474,#34475,#34476));
#6450=EDGE_LOOP('',(#34477,#34478,#34479,#34480));
#6451=EDGE_LOOP('',(#34481,#34482,#34483,#34484));
#6452=EDGE_LOOP('',(#34485,#34486,#34487,#34488,#34489));
#6453=EDGE_LOOP('',(#34490,#34491,#34492,#34493));
#6454=EDGE_LOOP('',(#34494,#34495,#34496,#34497,#34498));
#6455=EDGE_LOOP('',(#34499,#34500,#34501,#34502));
#6456=EDGE_LOOP('',(#34503,#34504,#34505,#34506));
#6457=EDGE_LOOP('',(#34507,#34508,#34509,#34510,#34511));
#6458=EDGE_LOOP('',(#34512,#34513,#34514,#34515));
#6459=EDGE_LOOP('',(#34516,#34517,#34518,#34519,#34520));
#6460=EDGE_LOOP('',(#34521,#34522,#34523,#34524));
#6461=EDGE_LOOP('',(#34525,#34526,#34527,#34528));
#6462=EDGE_LOOP('',(#34529,#34530,#34531,#34532,#34533));
#6463=EDGE_LOOP('',(#34534,#34535,#34536,#34537));
#6464=EDGE_LOOP('',(#34538,#34539,#34540,#34541,#34542));
#6465=EDGE_LOOP('',(#34543,#34544,#34545,#34546));
#6466=EDGE_LOOP('',(#34547,#34548,#34549,#34550));
#6467=EDGE_LOOP('',(#34551,#34552,#34553,#34554,#34555));
#6468=EDGE_LOOP('',(#34556,#34557,#34558,#34559));
#6469=EDGE_LOOP('',(#34560,#34561,#34562,#34563,#34564));
#6470=EDGE_LOOP('',(#34565,#34566,#34567,#34568));
#6471=EDGE_LOOP('',(#34569,#34570,#34571,#34572));
#6472=EDGE_LOOP('',(#34573,#34574,#34575,#34576,#34577));
#6473=EDGE_LOOP('',(#34578,#34579,#34580,#34581));
#6474=EDGE_LOOP('',(#34582,#34583,#34584,#34585,#34586));
#6475=EDGE_LOOP('',(#34587,#34588,#34589,#34590));
#6476=EDGE_LOOP('',(#34591,#34592,#34593,#34594));
#6477=EDGE_LOOP('',(#34595,#34596,#34597,#34598,#34599));
#6478=EDGE_LOOP('',(#34600,#34601,#34602,#34603));
#6479=EDGE_LOOP('',(#34604,#34605,#34606,#34607,#34608));
#6480=EDGE_LOOP('',(#34609,#34610,#34611,#34612));
#6481=EDGE_LOOP('',(#34613,#34614,#34615,#34616));
#6482=EDGE_LOOP('',(#34617,#34618,#34619,#34620,#34621));
#6483=EDGE_LOOP('',(#34622,#34623,#34624,#34625));
#6484=EDGE_LOOP('',(#34626,#34627,#34628,#34629,#34630));
#6485=EDGE_LOOP('',(#34631,#34632,#34633,#34634));
#6486=EDGE_LOOP('',(#34635,#34636,#34637,#34638));
#6487=EDGE_LOOP('',(#34639,#34640,#34641,#34642,#34643));
#6488=EDGE_LOOP('',(#34644,#34645,#34646,#34647));
#6489=EDGE_LOOP('',(#34648,#34649,#34650,#34651,#34652));
#6490=EDGE_LOOP('',(#34653,#34654,#34655,#34656));
#6491=EDGE_LOOP('',(#34657,#34658,#34659,#34660));
#6492=EDGE_LOOP('',(#34661,#34662,#34663,#34664,#34665));
#6493=EDGE_LOOP('',(#34666,#34667,#34668,#34669));
#6494=EDGE_LOOP('',(#34670,#34671,#34672,#34673,#34674));
#6495=EDGE_LOOP('',(#34675,#34676,#34677,#34678));
#6496=EDGE_LOOP('',(#34679,#34680,#34681,#34682));
#6497=EDGE_LOOP('',(#34683,#34684,#34685,#34686,#34687));
#6498=EDGE_LOOP('',(#34688,#34689,#34690,#34691));
#6499=EDGE_LOOP('',(#34692,#34693,#34694,#34695,#34696));
#6500=EDGE_LOOP('',(#34697,#34698,#34699,#34700));
#6501=EDGE_LOOP('',(#34701,#34702,#34703,#34704,#34705,#34706,#34707,#34708,
#34709,#34710,#34711,#34712,#34713,#34714,#34715,#34716,#34717,#34718,#34719,
#34720,#34721,#34722,#34723,#34724,#34725,#34726,#34727,#34728,#34729,#34730,
#34731,#34732,#34733,#34734,#34735,#34736,#34737,#34738,#34739,#34740,#34741,
#34742,#34743,#34744,#34745,#34746,#34747,#34748,#34749,#34750,#34751,#34752,
#34753,#34754,#34755,#34756,#34757,#34758,#34759,#34760,#34761,#34762,#34763,
#34764,#34765,#34766,#34767,#34768,#34769,#34770,#34771,#34772,#34773,#34774,
#34775,#34776,#34777,#34778,#34779,#34780,#34781,#34782,#34783,#34784,#34785,
#34786,#34787,#34788,#34789,#34790,#34791,#34792,#34793,#34794,#34795,#34796));
#8705=CIRCLE('',#43848,12.);
#8706=CIRCLE('',#43852,12.);
#8707=CIRCLE('',#43853,12.);
#8708=CIRCLE('',#43854,12.);
#8709=CIRCLE('',#43855,12.);
#8710=CIRCLE('',#43856,12.);
#8711=CIRCLE('',#43857,12.);
#8712=CIRCLE('',#43858,12.);
#8713=CIRCLE('',#43859,12.);
#8714=CIRCLE('',#43860,12.);
#8715=CIRCLE('',#43861,12.);
#8716=CIRCLE('',#43862,12.);
#8717=CIRCLE('',#43863,12.);
#8718=CIRCLE('',#43864,12.);
#8719=CIRCLE('',#43865,12.);
#8720=CIRCLE('',#43866,12.);
#8721=CIRCLE('',#43867,12.);
#8722=CIRCLE('',#43868,12.);
#8723=CIRCLE('',#43869,12.);
#8724=CIRCLE('',#43870,12.);
#8725=CIRCLE('',#43871,12.);
#8726=CIRCLE('',#43872,12.);
#8727=CIRCLE('',#43873,12.);
#8728=CIRCLE('',#43874,12.);
#8729=CIRCLE('',#43875,12.);
#8730=CIRCLE('',#43876,12.);
#8731=CIRCLE('',#43877,12.);
#8732=CIRCLE('',#43878,12.);
#8733=CIRCLE('',#43879,12.);
#8734=CIRCLE('',#43880,12.);
#8735=CIRCLE('',#43881,12.);
#8736=CIRCLE('',#43882,12.);
#8737=CIRCLE('',#43883,12.);
#8738=CIRCLE('',#43884,12.);
#8739=CIRCLE('',#43885,12.);
#8740=CIRCLE('',#43886,12.);
#8741=CIRCLE('',#43887,12.);
#8742=CIRCLE('',#43888,12.);
#8743=CIRCLE('',#43889,12.);
#8744=CIRCLE('',#43890,12.);
#8745=CIRCLE('',#43891,12.);
#8746=CIRCLE('',#43892,12.);
#8747=CIRCLE('',#43893,12.);
#8748=CIRCLE('',#43894,12.);
#8749=CIRCLE('',#43895,12.);
#8750=CIRCLE('',#43896,12.);
#8751=CIRCLE('',#43897,12.);
#8752=CIRCLE('',#43898,12.);
#8753=CIRCLE('',#43899,12.);
#8754=CIRCLE('',#43900,12.);
#8755=CIRCLE('',#43901,12.);
#8756=CIRCLE('',#43902,12.);
#8757=CIRCLE('',#43903,12.);
#8758=CIRCLE('',#43904,12.);
#8759=CIRCLE('',#43905,12.);
#8760=CIRCLE('',#43906,12.);
#8761=CIRCLE('',#43907,12.);
#8762=CIRCLE('',#43908,12.);
#8763=CIRCLE('',#43909,12.);
#8764=CIRCLE('',#43910,12.);
#8765=CIRCLE('',#43911,12.);
#8766=CIRCLE('',#43912,12.);
#8767=CIRCLE('',#43913,12.);
#8768=CIRCLE('',#43914,12.);
#8769=CIRCLE('',#43915,12.);
#8770=CIRCLE('',#43916,12.);
#8771=CIRCLE('',#43917,12.);
#8772=CIRCLE('',#43918,12.);
#8773=CIRCLE('',#43919,12.);
#8774=CIRCLE('',#43920,12.);
#8775=CIRCLE('',#43921,12.);
#8776=CIRCLE('',#43922,12.);
#8777=CIRCLE('',#43923,12.);
#8778=CIRCLE('',#43924,12.);
#8779=CIRCLE('',#43925,12.);
#8780=CIRCLE('',#43926,12.);
#8781=CIRCLE('',#43927,12.);
#8782=CIRCLE('',#43928,12.);
#8783=CIRCLE('',#43929,12.);
#8784=CIRCLE('',#43930,12.);
#8785=CIRCLE('',#43931,12.);
#8786=CIRCLE('',#43932,12.);
#8787=CIRCLE('',#43933,12.);
#8788=CIRCLE('',#43934,12.);
#8789=CIRCLE('',#43935,12.);
#8790=CIRCLE('',#43936,12.);
#8791=CIRCLE('',#43937,12.);
#8792=CIRCLE('',#43938,12.);
#8793=CIRCLE('',#43939,12.);
#8794=CIRCLE('',#43940,12.);
#8795=CIRCLE('',#43941,12.);
#8796=CIRCLE('',#43942,12.);
#8797=CIRCLE('',#43943,12.);
#8798=CIRCLE('',#43944,12.);
#8799=CIRCLE('',#43945,12.);
#8800=CIRCLE('',#43946,12.);
#8801=CIRCLE('',#43947,12.);
#8802=CIRCLE('',#43948,12.);
#8803=CIRCLE('',#43950,11.4);
#8804=CIRCLE('',#43952,11.4);
#8805=CIRCLE('',#43958,11.4);
#8806=CIRCLE('',#43964,11.4);
#8807=CIRCLE('',#43970,11.4);
#8808=CIRCLE('',#43976,11.4);
#8809=CIRCLE('',#43982,11.4);
#8810=CIRCLE('',#43988,11.4);
#8811=CIRCLE('',#43994,11.4);
#8812=CIRCLE('',#44000,11.4);
#8813=CIRCLE('',#44006,11.4);
#8814=CIRCLE('',#44012,11.4);
#8815=CIRCLE('',#44018,11.4);
#8816=CIRCLE('',#44024,11.4);
#8817=CIRCLE('',#44030,11.4);
#8818=CIRCLE('',#44036,11.4);
#8819=CIRCLE('',#44042,11.4);
#8820=CIRCLE('',#44048,11.4);
#8821=CIRCLE('',#44054,11.4);
#8822=CIRCLE('',#44060,11.4);
#8823=CIRCLE('',#44066,11.4);
#8824=CIRCLE('',#44072,11.4);
#8825=CIRCLE('',#44078,11.4);
#8826=CIRCLE('',#44084,11.4);
#8827=CIRCLE('',#44094,11.4);
#8828=CIRCLE('',#44095,11.4);
#8829=CIRCLE('',#44096,11.4);
#8830=CIRCLE('',#44097,11.4);
#8831=CIRCLE('',#44098,11.4);
#8832=CIRCLE('',#44099,11.4);
#8833=CIRCLE('',#44100,11.4);
#8834=CIRCLE('',#44101,11.4);
#8835=CIRCLE('',#44102,11.4);
#8836=CIRCLE('',#44103,11.4);
#8837=CIRCLE('',#44104,11.4);
#8838=CIRCLE('',#44105,11.4);
#8839=CIRCLE('',#44106,11.4);
#8840=CIRCLE('',#44107,11.4);
#8841=CIRCLE('',#44108,11.4);
#8842=CIRCLE('',#44109,11.4);
#8843=CIRCLE('',#44110,11.4);
#8844=CIRCLE('',#44111,11.4);
#8845=CIRCLE('',#44112,11.4);
#8846=CIRCLE('',#44113,11.4);
#8847=CIRCLE('',#44114,11.4);
#8848=CIRCLE('',#44115,11.4);
#8849=CIRCLE('',#44116,11.4);
#8850=CIRCLE('',#44117,11.4);
#11855=LINE('',#83025,#14349);
#11856=LINE('',#83027,#14350);
#11857=LINE('',#83029,#14351);
#11858=LINE('',#83031,#14352);
#11859=LINE('',#83039,#14353);
#11860=LINE('',#83040,#14354);
#11861=LINE('',#83044,#14355);
#11862=LINE('',#83049,#14356);
#11863=LINE('',#83050,#14357);
#11864=LINE('',#83052,#14358);
#11865=LINE('',#83057,#14359);
#11866=LINE('',#83061,#14360);
#11867=LINE('',#83065,#14361);
#11868=LINE('',#83069,#14362);
#11869=LINE('',#83073,#14363);
#11870=LINE('',#83077,#14364);
#11871=LINE('',#83081,#14365);
#11872=LINE('',#83085,#14366);
#11873=LINE('',#83089,#14367);
#11874=LINE('',#83093,#14368);
#11875=LINE('',#83097,#14369);
#11876=LINE('',#83101,#14370);
#11877=LINE('',#83105,#14371);
#11878=LINE('',#83109,#14372);
#11879=LINE('',#83113,#14373);
#11880=LINE('',#83117,#14374);
#11881=LINE('',#83121,#14375);
#11882=LINE('',#83125,#14376);
#11883=LINE('',#83129,#14377);
#11884=LINE('',#83133,#14378);
#11885=LINE('',#83137,#14379);
#11886=LINE('',#83141,#14380);
#11887=LINE('',#83145,#14381);
#11888=LINE('',#83149,#14382);
#11889=LINE('',#83153,#14383);
#11890=LINE('',#83157,#14384);
#11891=LINE('',#83161,#14385);
#11892=LINE('',#83165,#14386);
#11893=LINE('',#83169,#14387);
#11894=LINE('',#83173,#14388);
#11895=LINE('',#83177,#14389);
#11896=LINE('',#83181,#14390);
#11897=LINE('',#83185,#14391);
#11898=LINE('',#83189,#14392);
#11899=LINE('',#83193,#14393);
#11900=LINE('',#83197,#14394);
#11901=LINE('',#83201,#14395);
#11902=LINE('',#83205,#14396);
#11903=LINE('',#83209,#14397);
#11904=LINE('',#83213,#14398);
#11905=LINE('',#83217,#14399);
#11906=LINE('',#83221,#14400);
#11907=LINE('',#83225,#14401);
#11908=LINE('',#83229,#14402);
#11909=LINE('',#83233,#14403);
#11910=LINE('',#83237,#14404);
#11911=LINE('',#83241,#14405);
#11912=LINE('',#83245,#14406);
#11913=LINE('',#83249,#14407);
#11914=LINE('',#83253,#14408);
#11915=LINE('',#83257,#14409);
#11916=LINE('',#83261,#14410);
#11917=LINE('',#83265,#14411);
#11918=LINE('',#83269,#14412);
#11919=LINE('',#83273,#14413);
#11920=LINE('',#83277,#14414);
#11921=LINE('',#83281,#14415);
#11922=LINE('',#83285,#14416);
#11923=LINE('',#83289,#14417);
#11924=LINE('',#83293,#14418);
#11925=LINE('',#83297,#14419);
#11926=LINE('',#83301,#14420);
#11927=LINE('',#83305,#14421);
#11928=LINE('',#83309,#14422);
#11929=LINE('',#83313,#14423);
#11930=LINE('',#83317,#14424);
#11931=LINE('',#83321,#14425);
#11932=LINE('',#83325,#14426);
#11933=LINE('',#83329,#14427);
#11934=LINE('',#83333,#14428);
#11935=LINE('',#83338,#14429);
#11936=LINE('',#83342,#14430);
#11937=LINE('',#83346,#14431);
#11938=LINE('',#83350,#14432);
#11939=LINE('',#83354,#14433);
#11940=LINE('',#83358,#14434);
#11941=LINE('',#83362,#14435);
#11942=LINE('',#83366,#14436);
#11943=LINE('',#83370,#14437);
#11944=LINE('',#83374,#14438);
#11945=LINE('',#83378,#14439);
#11946=LINE('',#83382,#14440);
#11947=LINE('',#83386,#14441);
#11948=LINE('',#83390,#14442);
#11949=LINE('',#83394,#14443);
#11950=LINE('',#83398,#14444);
#11951=LINE('',#83402,#14445);
#11952=LINE('',#83406,#14446);
#11953=LINE('',#83410,#14447);
#11954=LINE('',#83414,#14448);
#11955=LINE('',#83418,#14449);
#11956=LINE('',#83422,#14450);
#11957=LINE('',#83426,#14451);
#11958=LINE('',#83430,#14452);
#11959=LINE('',#83434,#14453);
#11960=LINE('',#83450,#14454);
#11961=LINE('',#83452,#14455);
#11962=LINE('',#83453,#14456);
#11963=LINE('',#83456,#14457);
#11964=LINE('',#83457,#14458);
#11965=LINE('',#83461,#14459);
#11966=LINE('',#83465,#14460);
#11967=LINE('',#83467,#14461);
#11968=LINE('',#83476,#14462);
#11969=LINE('',#83478,#14463);
#11970=LINE('',#83479,#14464);
#11971=LINE('',#83482,#14465);
#11972=LINE('',#83483,#14466);
#11973=LINE('',#83487,#14467);
#11974=LINE('',#83491,#14468);
#11975=LINE('',#83493,#14469);
#11976=LINE('',#83502,#14470);
#11977=LINE('',#83504,#14471);
#11978=LINE('',#83505,#14472);
#11979=LINE('',#83508,#14473);
#11980=LINE('',#83509,#14474);
#11981=LINE('',#83513,#14475);
#11982=LINE('',#83517,#14476);
#11983=LINE('',#83519,#14477);
#11984=LINE('',#83528,#14478);
#11985=LINE('',#83530,#14479);
#11986=LINE('',#83531,#14480);
#11987=LINE('',#83534,#14481);
#11988=LINE('',#83535,#14482);
#11989=LINE('',#83539,#14483);
#11990=LINE('',#83543,#14484);
#11991=LINE('',#83545,#14485);
#11992=LINE('',#83554,#14486);
#11993=LINE('',#83556,#14487);
#11994=LINE('',#83557,#14488);
#11995=LINE('',#83560,#14489);
#11996=LINE('',#83561,#14490);
#11997=LINE('',#83565,#14491);
#11998=LINE('',#83569,#14492);
#11999=LINE('',#83571,#14493);
#12000=LINE('',#83580,#14494);
#12001=LINE('',#83582,#14495);
#12002=LINE('',#83583,#14496);
#12003=LINE('',#83586,#14497);
#12004=LINE('',#83587,#14498);
#12005=LINE('',#83591,#14499);
#12006=LINE('',#83595,#14500);
#12007=LINE('',#83597,#14501);
#12008=LINE('',#83606,#14502);
#12009=LINE('',#83608,#14503);
#12010=LINE('',#83609,#14504);
#12011=LINE('',#83612,#14505);
#12012=LINE('',#83613,#14506);
#12013=LINE('',#83617,#14507);
#12014=LINE('',#83621,#14508);
#12015=LINE('',#83623,#14509);
#12016=LINE('',#83632,#14510);
#12017=LINE('',#83634,#14511);
#12018=LINE('',#83635,#14512);
#12019=LINE('',#83638,#14513);
#12020=LINE('',#83639,#14514);
#12021=LINE('',#83643,#14515);
#12022=LINE('',#83647,#14516);
#12023=LINE('',#83649,#14517);
#12024=LINE('',#83658,#14518);
#12025=LINE('',#83660,#14519);
#12026=LINE('',#83661,#14520);
#12027=LINE('',#83664,#14521);
#12028=LINE('',#83665,#14522);
#12029=LINE('',#83669,#14523);
#12030=LINE('',#83673,#14524);
#12031=LINE('',#83675,#14525);
#12032=LINE('',#83684,#14526);
#12033=LINE('',#83686,#14527);
#12034=LINE('',#83687,#14528);
#12035=LINE('',#83690,#14529);
#12036=LINE('',#83691,#14530);
#12037=LINE('',#83695,#14531);
#12038=LINE('',#83699,#14532);
#12039=LINE('',#83701,#14533);
#12040=LINE('',#83710,#14534);
#12041=LINE('',#83712,#14535);
#12042=LINE('',#83713,#14536);
#12043=LINE('',#83716,#14537);
#12044=LINE('',#83717,#14538);
#12045=LINE('',#83721,#14539);
#12046=LINE('',#83725,#14540);
#12047=LINE('',#83727,#14541);
#12048=LINE('',#83736,#14542);
#12049=LINE('',#83738,#14543);
#12050=LINE('',#83739,#14544);
#12051=LINE('',#83742,#14545);
#12052=LINE('',#83743,#14546);
#12053=LINE('',#83747,#14547);
#12054=LINE('',#83751,#14548);
#12055=LINE('',#83753,#14549);
#12056=LINE('',#83762,#14550);
#12057=LINE('',#83764,#14551);
#12058=LINE('',#83765,#14552);
#12059=LINE('',#83768,#14553);
#12060=LINE('',#83769,#14554);
#12061=LINE('',#83773,#14555);
#12062=LINE('',#83777,#14556);
#12063=LINE('',#83779,#14557);
#12064=LINE('',#83788,#14558);
#12065=LINE('',#83790,#14559);
#12066=LINE('',#83791,#14560);
#12067=LINE('',#83794,#14561);
#12068=LINE('',#83795,#14562);
#12069=LINE('',#83799,#14563);
#12070=LINE('',#83803,#14564);
#12071=LINE('',#83805,#14565);
#12072=LINE('',#83814,#14566);
#12073=LINE('',#83816,#14567);
#12074=LINE('',#83817,#14568);
#12075=LINE('',#83820,#14569);
#12076=LINE('',#83821,#14570);
#12077=LINE('',#83825,#14571);
#12078=LINE('',#83829,#14572);
#12079=LINE('',#83831,#14573);
#12080=LINE('',#83840,#14574);
#12081=LINE('',#83842,#14575);
#12082=LINE('',#83843,#14576);
#12083=LINE('',#83846,#14577);
#12084=LINE('',#83847,#14578);
#12085=LINE('',#83851,#14579);
#12086=LINE('',#83855,#14580);
#12087=LINE('',#83857,#14581);
#12088=LINE('',#83866,#14582);
#12089=LINE('',#83868,#14583);
#12090=LINE('',#83869,#14584);
#12091=LINE('',#83872,#14585);
#12092=LINE('',#83873,#14586);
#12093=LINE('',#83877,#14587);
#12094=LINE('',#83881,#14588);
#12095=LINE('',#83883,#14589);
#12096=LINE('',#83892,#14590);
#12097=LINE('',#83894,#14591);
#12098=LINE('',#83895,#14592);
#12099=LINE('',#83898,#14593);
#12100=LINE('',#83899,#14594);
#12101=LINE('',#83903,#14595);
#12102=LINE('',#83907,#14596);
#12103=LINE('',#83909,#14597);
#12104=LINE('',#83918,#14598);
#12105=LINE('',#83920,#14599);
#12106=LINE('',#83921,#14600);
#12107=LINE('',#83924,#14601);
#12108=LINE('',#83925,#14602);
#12109=LINE('',#83929,#14603);
#12110=LINE('',#83933,#14604);
#12111=LINE('',#83935,#14605);
#12112=LINE('',#83944,#14606);
#12113=LINE('',#83946,#14607);
#12114=LINE('',#83947,#14608);
#12115=LINE('',#83950,#14609);
#12116=LINE('',#83951,#14610);
#12117=LINE('',#83955,#14611);
#12118=LINE('',#83959,#14612);
#12119=LINE('',#83961,#14613);
#12120=LINE('',#83970,#14614);
#12121=LINE('',#83972,#14615);
#12122=LINE('',#83973,#14616);
#12123=LINE('',#83976,#14617);
#12124=LINE('',#83977,#14618);
#12125=LINE('',#83981,#14619);
#12126=LINE('',#83985,#14620);
#12127=LINE('',#83987,#14621);
#12128=LINE('',#83996,#14622);
#12129=LINE('',#83998,#14623);
#12130=LINE('',#83999,#14624);
#12131=LINE('',#84002,#14625);
#12132=LINE('',#84003,#14626);
#12133=LINE('',#84007,#14627);
#12134=LINE('',#84011,#14628);
#12135=LINE('',#84013,#14629);
#12136=LINE('',#84022,#14630);
#12137=LINE('',#84024,#14631);
#12138=LINE('',#84025,#14632);
#12139=LINE('',#84028,#14633);
#12140=LINE('',#84029,#14634);
#12141=LINE('',#84032,#14635);
#12142=LINE('',#84033,#14636);
#12143=LINE('',#84035,#14637);
#12144=LINE('',#84038,#14638);
#12145=LINE('',#84040,#14639);
#12146=LINE('',#84042,#14640);
#12147=LINE('',#84048,#14641);
#12148=LINE('',#84050,#14642);
#12149=LINE('',#84051,#14643);
#12150=LINE('',#84057,#14644);
#12151=LINE('',#84058,#14645);
#12152=LINE('',#84064,#14646);
#12153=LINE('',#84066,#14647);
#12154=LINE('',#84068,#14648);
#12155=LINE('',#84072,#14649);
#12156=LINE('',#84074,#14650);
#12157=LINE('',#84076,#14651);
#12158=LINE('',#84080,#14652);
#12159=LINE('',#84082,#14653);
#12160=LINE('',#84084,#14654);
#12161=LINE('',#84088,#14655);
#12162=LINE('',#84090,#14656);
#12163=LINE('',#84092,#14657);
#12164=LINE('',#84096,#14658);
#12165=LINE('',#84098,#14659);
#12166=LINE('',#84100,#14660);
#12167=LINE('',#84104,#14661);
#12168=LINE('',#84106,#14662);
#12169=LINE('',#84108,#14663);
#12170=LINE('',#84112,#14664);
#12171=LINE('',#84114,#14665);
#12172=LINE('',#84116,#14666);
#12173=LINE('',#84120,#14667);
#12174=LINE('',#84122,#14668);
#12175=LINE('',#84124,#14669);
#12176=LINE('',#84128,#14670);
#12177=LINE('',#84130,#14671);
#12178=LINE('',#84132,#14672);
#12179=LINE('',#84136,#14673);
#12180=LINE('',#84138,#14674);
#12181=LINE('',#84140,#14675);
#12182=LINE('',#84144,#14676);
#12183=LINE('',#84146,#14677);
#12184=LINE('',#84148,#14678);
#12185=LINE('',#84152,#14679);
#12186=LINE('',#84154,#14680);
#12187=LINE('',#84156,#14681);
#12188=LINE('',#84160,#14682);
#12189=LINE('',#84162,#14683);
#12190=LINE('',#84164,#14684);
#12191=LINE('',#84168,#14685);
#12192=LINE('',#84170,#14686);
#12193=LINE('',#84172,#14687);
#12194=LINE('',#84176,#14688);
#12195=LINE('',#84178,#14689);
#12196=LINE('',#84180,#14690);
#12197=LINE('',#84184,#14691);
#12198=LINE('',#84186,#14692);
#12199=LINE('',#84188,#14693);
#12200=LINE('',#84192,#14694);
#12201=LINE('',#84194,#14695);
#12202=LINE('',#84196,#14696);
#12203=LINE('',#84200,#14697);
#12204=LINE('',#84202,#14698);
#12205=LINE('',#84204,#14699);
#12206=LINE('',#84208,#14700);
#12207=LINE('',#84210,#14701);
#12208=LINE('',#84212,#14702);
#12209=LINE('',#84216,#14703);
#12210=LINE('',#84218,#14704);
#12211=LINE('',#84220,#14705);
#12212=LINE('',#84224,#14706);
#12213=LINE('',#84226,#14707);
#12214=LINE('',#84228,#14708);
#12215=LINE('',#84232,#14709);
#12216=LINE('',#84234,#14710);
#12217=LINE('',#84236,#14711);
#12218=LINE('',#84240,#14712);
#12219=LINE('',#84242,#14713);
#12220=LINE('',#84244,#14714);
#12221=LINE('',#84256,#14715);
#12222=LINE('',#84257,#14716);
#12223=LINE('',#84260,#14717);
#12224=LINE('',#84261,#14718);
#12225=LINE('',#84266,#14719);
#12226=LINE('',#84274,#14720);
#12227=LINE('',#84275,#14721);
#12228=LINE('',#84278,#14722);
#12229=LINE('',#84279,#14723);
#12230=LINE('',#84284,#14724);
#12231=LINE('',#84292,#14725);
#12232=LINE('',#84293,#14726);
#12233=LINE('',#84296,#14727);
#12234=LINE('',#84297,#14728);
#12235=LINE('',#84302,#14729);
#12236=LINE('',#84310,#14730);
#12237=LINE('',#84311,#14731);
#12238=LINE('',#84314,#14732);
#12239=LINE('',#84315,#14733);
#12240=LINE('',#84320,#14734);
#12241=LINE('',#84328,#14735);
#12242=LINE('',#84329,#14736);
#12243=LINE('',#84332,#14737);
#12244=LINE('',#84333,#14738);
#12245=LINE('',#84338,#14739);
#12246=LINE('',#84346,#14740);
#12247=LINE('',#84347,#14741);
#12248=LINE('',#84350,#14742);
#12249=LINE('',#84351,#14743);
#12250=LINE('',#84356,#14744);
#12251=LINE('',#84364,#14745);
#12252=LINE('',#84365,#14746);
#12253=LINE('',#84368,#14747);
#12254=LINE('',#84369,#14748);
#12255=LINE('',#84374,#14749);
#12256=LINE('',#84382,#14750);
#12257=LINE('',#84383,#14751);
#12258=LINE('',#84386,#14752);
#12259=LINE('',#84387,#14753);
#12260=LINE('',#84392,#14754);
#12261=LINE('',#84400,#14755);
#12262=LINE('',#84401,#14756);
#12263=LINE('',#84404,#14757);
#12264=LINE('',#84405,#14758);
#12265=LINE('',#84410,#14759);
#12266=LINE('',#84418,#14760);
#12267=LINE('',#84419,#14761);
#12268=LINE('',#84422,#14762);
#12269=LINE('',#84423,#14763);
#12270=LINE('',#84428,#14764);
#12271=LINE('',#84436,#14765);
#12272=LINE('',#84437,#14766);
#12273=LINE('',#84440,#14767);
#12274=LINE('',#84441,#14768);
#12275=LINE('',#84446,#14769);
#12276=LINE('',#84454,#14770);
#12277=LINE('',#84455,#14771);
#12278=LINE('',#84458,#14772);
#12279=LINE('',#84459,#14773);
#12280=LINE('',#84464,#14774);
#12281=LINE('',#84472,#14775);
#12282=LINE('',#84473,#14776);
#12283=LINE('',#84476,#14777);
#12284=LINE('',#84477,#14778);
#12285=LINE('',#84482,#14779);
#12286=LINE('',#84490,#14780);
#12287=LINE('',#84491,#14781);
#12288=LINE('',#84494,#14782);
#12289=LINE('',#84495,#14783);
#12290=LINE('',#84500,#14784);
#12291=LINE('',#84508,#14785);
#12292=LINE('',#84509,#14786);
#12293=LINE('',#84512,#14787);
#12294=LINE('',#84513,#14788);
#12295=LINE('',#84518,#14789);
#12296=LINE('',#84526,#14790);
#12297=LINE('',#84527,#14791);
#12298=LINE('',#84530,#14792);
#12299=LINE('',#84531,#14793);
#12300=LINE('',#84536,#14794);
#12301=LINE('',#84544,#14795);
#12302=LINE('',#84545,#14796);
#12303=LINE('',#84548,#14797);
#12304=LINE('',#84549,#14798);
#12305=LINE('',#84554,#14799);
#12306=LINE('',#84562,#14800);
#12307=LINE('',#84563,#14801);
#12308=LINE('',#84566,#14802);
#12309=LINE('',#84567,#14803);
#12310=LINE('',#84572,#14804);
#12311=LINE('',#84580,#14805);
#12312=LINE('',#84581,#14806);
#12313=LINE('',#84584,#14807);
#12314=LINE('',#84585,#14808);
#12315=LINE('',#84590,#14809);
#12316=LINE('',#84598,#14810);
#12317=LINE('',#84599,#14811);
#12318=LINE('',#84602,#14812);
#12319=LINE('',#84603,#14813);
#12320=LINE('',#84608,#14814);
#12321=LINE('',#84616,#14815);
#12322=LINE('',#84617,#14816);
#12323=LINE('',#84620,#14817);
#12324=LINE('',#84621,#14818);
#12325=LINE('',#84626,#14819);
#12326=LINE('',#84634,#14820);
#12327=LINE('',#84635,#14821);
#12328=LINE('',#84638,#14822);
#12329=LINE('',#84639,#14823);
#12330=LINE('',#84644,#14824);
#12331=LINE('',#84652,#14825);
#12332=LINE('',#84653,#14826);
#12333=LINE('',#84656,#14827);
#12334=LINE('',#84657,#14828);
#12335=LINE('',#84659,#14829);
#14349=VECTOR('',#53387,10.);
#14350=VECTOR('',#53388,10.);
#14351=VECTOR('',#53389,10.);
#14352=VECTOR('',#53390,10.);
#14353=VECTOR('',#53395,10.);
#14354=VECTOR('',#53396,10.);
#14355=VECTOR('',#53399,10.);
#14356=VECTOR('',#53400,10.);
#14357=VECTOR('',#53401,10.);
#14358=VECTOR('',#53404,10.);
#14359=VECTOR('',#53409,10.);
#14360=VECTOR('',#53412,10.);
#14361=VECTOR('',#53415,10.);
#14362=VECTOR('',#53418,10.);
#14363=VECTOR('',#53421,10.);
#14364=VECTOR('',#53424,10.);
#14365=VECTOR('',#53427,10.);
#14366=VECTOR('',#53430,10.);
#14367=VECTOR('',#53433,10.);
#14368=VECTOR('',#53436,10.);
#14369=VECTOR('',#53439,10.);
#14370=VECTOR('',#53442,10.);
#14371=VECTOR('',#53445,10.);
#14372=VECTOR('',#53448,10.);
#14373=VECTOR('',#53451,10.);
#14374=VECTOR('',#53454,10.);
#14375=VECTOR('',#53457,10.);
#14376=VECTOR('',#53460,10.);
#14377=VECTOR('',#53463,10.);
#14378=VECTOR('',#53466,10.);
#14379=VECTOR('',#53469,10.);
#14380=VECTOR('',#53472,12.);
#14381=VECTOR('',#53475,10.);
#14382=VECTOR('',#53478,10.);
#14383=VECTOR('',#53481,10.);
#14384=VECTOR('',#53484,10.);
#14385=VECTOR('',#53487,10.);
#14386=VECTOR('',#53490,10.);
#14387=VECTOR('',#53493,10.);
#14388=VECTOR('',#53496,10.);
#14389=VECTOR('',#53499,10.);
#14390=VECTOR('',#53502,10.);
#14391=VECTOR('',#53505,10.);
#14392=VECTOR('',#53508,10.);
#14393=VECTOR('',#53511,10.);
#14394=VECTOR('',#53514,10.);
#14395=VECTOR('',#53517,10.);
#14396=VECTOR('',#53520,10.);
#14397=VECTOR('',#53523,10.);
#14398=VECTOR('',#53526,10.);
#14399=VECTOR('',#53529,10.);
#14400=VECTOR('',#53532,10.);
#14401=VECTOR('',#53535,10.);
#14402=VECTOR('',#53538,10.);
#14403=VECTOR('',#53541,10.);
#14404=VECTOR('',#53544,10.);
#14405=VECTOR('',#53547,10.);
#14406=VECTOR('',#53550,10.);
#14407=VECTOR('',#53553,10.);
#14408=VECTOR('',#53556,10.);
#14409=VECTOR('',#53559,10.);
#14410=VECTOR('',#53562,10.);
#14411=VECTOR('',#53565,10.);
#14412=VECTOR('',#53568,10.);
#14413=VECTOR('',#53571,10.);
#14414=VECTOR('',#53574,10.);
#14415=VECTOR('',#53577,10.);
#14416=VECTOR('',#53580,10.);
#14417=VECTOR('',#53583,10.);
#14418=VECTOR('',#53586,10.);
#14419=VECTOR('',#53589,10.);
#14420=VECTOR('',#53592,10.);
#14421=VECTOR('',#53595,10.);
#14422=VECTOR('',#53598,10.);
#14423=VECTOR('',#53601,10.);
#14424=VECTOR('',#53604,10.);
#14425=VECTOR('',#53607,10.);
#14426=VECTOR('',#53610,10.);
#14427=VECTOR('',#53613,10.);
#14428=VECTOR('',#53616,10.);
#14429=VECTOR('',#53621,10.);
#14430=VECTOR('',#53624,10.);
#14431=VECTOR('',#53627,10.);
#14432=VECTOR('',#53630,10.);
#14433=VECTOR('',#53633,10.);
#14434=VECTOR('',#53636,10.);
#14435=VECTOR('',#53639,10.);
#14436=VECTOR('',#53642,10.);
#14437=VECTOR('',#53645,10.);
#14438=VECTOR('',#53648,10.);
#14439=VECTOR('',#53651,10.);
#14440=VECTOR('',#53654,10.);
#14441=VECTOR('',#53657,10.);
#14442=VECTOR('',#53660,10.);
#14443=VECTOR('',#53663,10.);
#14444=VECTOR('',#53666,10.);
#14445=VECTOR('',#53669,10.);
#14446=VECTOR('',#53672,10.);
#14447=VECTOR('',#53675,10.);
#14448=VECTOR('',#53678,10.);
#14449=VECTOR('',#53681,10.);
#14450=VECTOR('',#53684,10.);
#14451=VECTOR('',#53687,10.);
#14452=VECTOR('',#53690,10.);
#14453=VECTOR('',#53693,10.);
#14454=VECTOR('',#53706,10.);
#14455=VECTOR('',#53707,10.);
#14456=VECTOR('',#53708,10.);
#14457=VECTOR('',#53711,10.);
#14458=VECTOR('',#53712,10.);
#14459=VECTOR('',#53715,10.);
#14460=VECTOR('',#53716,10.);
#14461=VECTOR('',#53719,10.);
#14462=VECTOR('',#53726,10.);
#14463=VECTOR('',#53727,10.);
#14464=VECTOR('',#53728,10.);
#14465=VECTOR('',#53731,10.);
#14466=VECTOR('',#53732,10.);
#14467=VECTOR('',#53735,10.);
#14468=VECTOR('',#53736,10.);
#14469=VECTOR('',#53739,10.);
#14470=VECTOR('',#53746,10.);
#14471=VECTOR('',#53747,10.);
#14472=VECTOR('',#53748,10.);
#14473=VECTOR('',#53751,10.);
#14474=VECTOR('',#53752,10.);
#14475=VECTOR('',#53755,10.);
#14476=VECTOR('',#53756,10.);
#14477=VECTOR('',#53759,10.);
#14478=VECTOR('',#53766,10.);
#14479=VECTOR('',#53767,10.);
#14480=VECTOR('',#53768,10.);
#14481=VECTOR('',#53771,10.);
#14482=VECTOR('',#53772,10.);
#14483=VECTOR('',#53775,10.);
#14484=VECTOR('',#53776,10.);
#14485=VECTOR('',#53779,10.);
#14486=VECTOR('',#53786,10.);
#14487=VECTOR('',#53787,10.);
#14488=VECTOR('',#53788,10.);
#14489=VECTOR('',#53791,10.);
#14490=VECTOR('',#53792,10.);
#14491=VECTOR('',#53795,10.);
#14492=VECTOR('',#53796,10.);
#14493=VECTOR('',#53799,10.);
#14494=VECTOR('',#53806,10.);
#14495=VECTOR('',#53807,10.);
#14496=VECTOR('',#53808,10.);
#14497=VECTOR('',#53811,10.);
#14498=VECTOR('',#53812,10.);
#14499=VECTOR('',#53815,10.);
#14500=VECTOR('',#53816,10.);
#14501=VECTOR('',#53819,10.);
#14502=VECTOR('',#53826,10.);
#14503=VECTOR('',#53827,10.);
#14504=VECTOR('',#53828,10.);
#14505=VECTOR('',#53831,10.);
#14506=VECTOR('',#53832,10.);
#14507=VECTOR('',#53835,10.);
#14508=VECTOR('',#53836,10.);
#14509=VECTOR('',#53839,10.);
#14510=VECTOR('',#53846,10.);
#14511=VECTOR('',#53847,10.);
#14512=VECTOR('',#53848,10.);
#14513=VECTOR('',#53851,10.);
#14514=VECTOR('',#53852,10.);
#14515=VECTOR('',#53855,10.);
#14516=VECTOR('',#53856,10.);
#14517=VECTOR('',#53859,10.);
#14518=VECTOR('',#53866,10.);
#14519=VECTOR('',#53867,10.);
#14520=VECTOR('',#53868,10.);
#14521=VECTOR('',#53871,10.);
#14522=VECTOR('',#53872,10.);
#14523=VECTOR('',#53875,10.);
#14524=VECTOR('',#53876,10.);
#14525=VECTOR('',#53879,10.);
#14526=VECTOR('',#53886,10.);
#14527=VECTOR('',#53887,10.);
#14528=VECTOR('',#53888,10.);
#14529=VECTOR('',#53891,10.);
#14530=VECTOR('',#53892,10.);
#14531=VECTOR('',#53895,10.);
#14532=VECTOR('',#53896,10.);
#14533=VECTOR('',#53899,10.);
#14534=VECTOR('',#53906,10.);
#14535=VECTOR('',#53907,10.);
#14536=VECTOR('',#53908,10.);
#14537=VECTOR('',#53911,10.);
#14538=VECTOR('',#53912,10.);
#14539=VECTOR('',#53915,10.);
#14540=VECTOR('',#53916,10.);
#14541=VECTOR('',#53919,10.);
#14542=VECTOR('',#53926,10.);
#14543=VECTOR('',#53927,10.);
#14544=VECTOR('',#53928,10.);
#14545=VECTOR('',#53931,10.);
#14546=VECTOR('',#53932,10.);
#14547=VECTOR('',#53935,10.);
#14548=VECTOR('',#53936,10.);
#14549=VECTOR('',#53939,10.);
#14550=VECTOR('',#53946,10.);
#14551=VECTOR('',#53947,10.);
#14552=VECTOR('',#53948,10.);
#14553=VECTOR('',#53951,10.);
#14554=VECTOR('',#53952,10.);
#14555=VECTOR('',#53955,10.);
#14556=VECTOR('',#53956,10.);
#14557=VECTOR('',#53959,10.);
#14558=VECTOR('',#53966,10.);
#14559=VECTOR('',#53967,10.);
#14560=VECTOR('',#53968,10.);
#14561=VECTOR('',#53971,10.);
#14562=VECTOR('',#53972,10.);
#14563=VECTOR('',#53975,10.);
#14564=VECTOR('',#53976,10.);
#14565=VECTOR('',#53979,10.);
#14566=VECTOR('',#53986,10.);
#14567=VECTOR('',#53987,10.);
#14568=VECTOR('',#53988,10.);
#14569=VECTOR('',#53991,10.);
#14570=VECTOR('',#53992,10.);
#14571=VECTOR('',#53995,10.);
#14572=VECTOR('',#53996,10.);
#14573=VECTOR('',#53999,10.);
#14574=VECTOR('',#54006,10.);
#14575=VECTOR('',#54007,10.);
#14576=VECTOR('',#54008,10.);
#14577=VECTOR('',#54011,10.);
#14578=VECTOR('',#54012,10.);
#14579=VECTOR('',#54015,10.);
#14580=VECTOR('',#54016,10.);
#14581=VECTOR('',#54019,10.);
#14582=VECTOR('',#54026,10.);
#14583=VECTOR('',#54027,10.);
#14584=VECTOR('',#54028,10.);
#14585=VECTOR('',#54031,10.);
#14586=VECTOR('',#54032,10.);
#14587=VECTOR('',#54035,10.);
#14588=VECTOR('',#54036,10.);
#14589=VECTOR('',#54039,10.);
#14590=VECTOR('',#54046,10.);
#14591=VECTOR('',#54047,10.);
#14592=VECTOR('',#54048,10.);
#14593=VECTOR('',#54051,10.);
#14594=VECTOR('',#54052,10.);
#14595=VECTOR('',#54055,10.);
#14596=VECTOR('',#54056,10.);
#14597=VECTOR('',#54059,10.);
#14598=VECTOR('',#54066,10.);
#14599=VECTOR('',#54067,10.);
#14600=VECTOR('',#54068,10.);
#14601=VECTOR('',#54071,10.);
#14602=VECTOR('',#54072,10.);
#14603=VECTOR('',#54075,10.);
#14604=VECTOR('',#54076,10.);
#14605=VECTOR('',#54079,10.);
#14606=VECTOR('',#54086,10.);
#14607=VECTOR('',#54087,10.);
#14608=VECTOR('',#54088,10.);
#14609=VECTOR('',#54091,10.);
#14610=VECTOR('',#54092,10.);
#14611=VECTOR('',#54095,10.);
#14612=VECTOR('',#54096,10.);
#14613=VECTOR('',#54099,10.);
#14614=VECTOR('',#54106,10.);
#14615=VECTOR('',#54107,10.);
#14616=VECTOR('',#54108,10.);
#14617=VECTOR('',#54111,10.);
#14618=VECTOR('',#54112,10.);
#14619=VECTOR('',#54115,10.);
#14620=VECTOR('',#54116,10.);
#14621=VECTOR('',#54119,10.);
#14622=VECTOR('',#54126,10.);
#14623=VECTOR('',#54127,10.);
#14624=VECTOR('',#54128,10.);
#14625=VECTOR('',#54131,10.);
#14626=VECTOR('',#54132,10.);
#14627=VECTOR('',#54135,10.);
#14628=VECTOR('',#54136,10.);
#14629=VECTOR('',#54139,10.);
#14630=VECTOR('',#54146,10.);
#14631=VECTOR('',#54147,10.);
#14632=VECTOR('',#54148,10.);
#14633=VECTOR('',#54151,10.);
#14634=VECTOR('',#54152,10.);
#14635=VECTOR('',#54155,10.);
#14636=VECTOR('',#54156,10.);
#14637=VECTOR('',#54159,10.);
#14638=VECTOR('',#54162,10.);
#14639=VECTOR('',#54163,10.);
#14640=VECTOR('',#54164,10.);
#14641=VECTOR('',#54167,10.);
#14642=VECTOR('',#54168,10.);
#14643=VECTOR('',#54169,10.);
#14644=VECTOR('',#54172,10.);
#14645=VECTOR('',#54173,10.);
#14646=VECTOR('',#54180,10.);
#14647=VECTOR('',#54181,10.);
#14648=VECTOR('',#54182,10.);
#14649=VECTOR('',#54185,10.);
#14650=VECTOR('',#54186,10.);
#14651=VECTOR('',#54187,10.);
#14652=VECTOR('',#54190,10.);
#14653=VECTOR('',#54191,10.);
#14654=VECTOR('',#54192,10.);
#14655=VECTOR('',#54195,10.);
#14656=VECTOR('',#54196,10.);
#14657=VECTOR('',#54197,10.);
#14658=VECTOR('',#54200,10.);
#14659=VECTOR('',#54201,10.);
#14660=VECTOR('',#54202,10.);
#14661=VECTOR('',#54205,10.);
#14662=VECTOR('',#54206,10.);
#14663=VECTOR('',#54207,10.);
#14664=VECTOR('',#54210,10.);
#14665=VECTOR('',#54211,10.);
#14666=VECTOR('',#54212,10.);
#14667=VECTOR('',#54215,10.);
#14668=VECTOR('',#54216,10.);
#14669=VECTOR('',#54217,10.);
#14670=VECTOR('',#54220,10.);
#14671=VECTOR('',#54221,10.);
#14672=VECTOR('',#54222,10.);
#14673=VECTOR('',#54225,10.);
#14674=VECTOR('',#54226,10.);
#14675=VECTOR('',#54227,10.);
#14676=VECTOR('',#54230,10.);
#14677=VECTOR('',#54231,10.);
#14678=VECTOR('',#54232,10.);
#14679=VECTOR('',#54235,10.);
#14680=VECTOR('',#54236,10.);
#14681=VECTOR('',#54237,10.);
#14682=VECTOR('',#54240,10.);
#14683=VECTOR('',#54241,10.);
#14684=VECTOR('',#54242,10.);
#14685=VECTOR('',#54245,10.);
#14686=VECTOR('',#54246,10.);
#14687=VECTOR('',#54247,10.);
#14688=VECTOR('',#54250,10.);
#14689=VECTOR('',#54251,10.);
#14690=VECTOR('',#54252,10.);
#14691=VECTOR('',#54255,10.);
#14692=VECTOR('',#54256,10.);
#14693=VECTOR('',#54257,10.);
#14694=VECTOR('',#54260,10.);
#14695=VECTOR('',#54261,10.);
#14696=VECTOR('',#54262,10.);
#14697=VECTOR('',#54265,10.);
#14698=VECTOR('',#54266,10.);
#14699=VECTOR('',#54267,10.);
#14700=VECTOR('',#54270,10.);
#14701=VECTOR('',#54271,10.);
#14702=VECTOR('',#54272,10.);
#14703=VECTOR('',#54275,10.);
#14704=VECTOR('',#54276,10.);
#14705=VECTOR('',#54277,10.);
#14706=VECTOR('',#54280,10.);
#14707=VECTOR('',#54281,10.);
#14708=VECTOR('',#54282,10.);
#14709=VECTOR('',#54285,10.);
#14710=VECTOR('',#54286,10.);
#14711=VECTOR('',#54287,10.);
#14712=VECTOR('',#54290,10.);
#14713=VECTOR('',#54291,10.);
#14714=VECTOR('',#54292,10.);
#14715=VECTOR('',#54301,10.);
#14716=VECTOR('',#54302,10.);
#14717=VECTOR('',#54305,10.);
#14718=VECTOR('',#54306,10.);
#14719=VECTOR('',#54309,10.);
#14720=VECTOR('',#54316,10.);
#14721=VECTOR('',#54317,10.);
#14722=VECTOR('',#54320,10.);
#14723=VECTOR('',#54321,10.);
#14724=VECTOR('',#54324,10.);
#14725=VECTOR('',#54331,10.);
#14726=VECTOR('',#54332,10.);
#14727=VECTOR('',#54335,10.);
#14728=VECTOR('',#54336,10.);
#14729=VECTOR('',#54339,10.);
#14730=VECTOR('',#54346,10.);
#14731=VECTOR('',#54347,10.);
#14732=VECTOR('',#54350,10.);
#14733=VECTOR('',#54351,10.);
#14734=VECTOR('',#54354,10.);
#14735=VECTOR('',#54361,10.);
#14736=VECTOR('',#54362,10.);
#14737=VECTOR('',#54365,10.);
#14738=VECTOR('',#54366,10.);
#14739=VECTOR('',#54369,10.);
#14740=VECTOR('',#54376,10.);
#14741=VECTOR('',#54377,10.);
#14742=VECTOR('',#54380,10.);
#14743=VECTOR('',#54381,10.);
#14744=VECTOR('',#54384,10.);
#14745=VECTOR('',#54391,10.);
#14746=VECTOR('',#54392,10.);
#14747=VECTOR('',#54395,10.);
#14748=VECTOR('',#54396,10.);
#14749=VECTOR('',#54399,10.);
#14750=VECTOR('',#54406,10.);
#14751=VECTOR('',#54407,10.);
#14752=VECTOR('',#54410,10.);
#14753=VECTOR('',#54411,10.);
#14754=VECTOR('',#54414,10.);
#14755=VECTOR('',#54421,10.);
#14756=VECTOR('',#54422,10.);
#14757=VECTOR('',#54425,10.);
#14758=VECTOR('',#54426,10.);
#14759=VECTOR('',#54429,10.);
#14760=VECTOR('',#54436,10.);
#14761=VECTOR('',#54437,10.);
#14762=VECTOR('',#54440,10.);
#14763=VECTOR('',#54441,10.);
#14764=VECTOR('',#54444,10.);
#14765=VECTOR('',#54451,10.);
#14766=VECTOR('',#54452,10.);
#14767=VECTOR('',#54455,10.);
#14768=VECTOR('',#54456,10.);
#14769=VECTOR('',#54459,10.);
#14770=VECTOR('',#54466,10.);
#14771=VECTOR('',#54467,10.);
#14772=VECTOR('',#54470,10.);
#14773=VECTOR('',#54471,10.);
#14774=VECTOR('',#54474,10.);
#14775=VECTOR('',#54481,10.);
#14776=VECTOR('',#54482,10.);
#14777=VECTOR('',#54485,10.);
#14778=VECTOR('',#54486,10.);
#14779=VECTOR('',#54489,10.);
#14780=VECTOR('',#54496,10.);
#14781=VECTOR('',#54497,10.);
#14782=VECTOR('',#54500,10.);
#14783=VECTOR('',#54501,10.);
#14784=VECTOR('',#54504,10.);
#14785=VECTOR('',#54511,10.);
#14786=VECTOR('',#54512,10.);
#14787=VECTOR('',#54515,10.);
#14788=VECTOR('',#54516,10.);
#14789=VECTOR('',#54519,10.);
#14790=VECTOR('',#54526,10.);
#14791=VECTOR('',#54527,10.);
#14792=VECTOR('',#54530,10.);
#14793=VECTOR('',#54531,10.);
#14794=VECTOR('',#54534,10.);
#14795=VECTOR('',#54541,10.);
#14796=VECTOR('',#54542,10.);
#14797=VECTOR('',#54545,10.);
#14798=VECTOR('',#54546,10.);
#14799=VECTOR('',#54549,10.);
#14800=VECTOR('',#54556,10.);
#14801=VECTOR('',#54557,10.);
#14802=VECTOR('',#54560,10.);
#14803=VECTOR('',#54561,10.);
#14804=VECTOR('',#54564,10.);
#14805=VECTOR('',#54571,10.);
#14806=VECTOR('',#54572,10.);
#14807=VECTOR('',#54575,10.);
#14808=VECTOR('',#54576,10.);
#14809=VECTOR('',#54579,10.);
#14810=VECTOR('',#54586,10.);
#14811=VECTOR('',#54587,10.);
#14812=VECTOR('',#54590,10.);
#14813=VECTOR('',#54591,10.);
#14814=VECTOR('',#54594,10.);
#14815=VECTOR('',#54601,10.);
#14816=VECTOR('',#54602,10.);
#14817=VECTOR('',#54605,10.);
#14818=VECTOR('',#54606,10.);
#14819=VECTOR('',#54609,10.);
#14820=VECTOR('',#54616,10.);
#14821=VECTOR('',#54617,10.);
#14822=VECTOR('',#54620,10.);
#14823=VECTOR('',#54621,10.);
#14824=VECTOR('',#54624,10.);
#14825=VECTOR('',#54631,10.);
#14826=VECTOR('',#54632,10.);
#14827=VECTOR('',#54635,10.);
#14828=VECTOR('',#54636,10.);
#14829=VECTOR('',#54639,10.);
#17800=VERTEX_POINT('',#83023);
#17801=VERTEX_POINT('',#83024);
#17802=VERTEX_POINT('',#83026);
#17803=VERTEX_POINT('',#83028);
#17804=VERTEX_POINT('',#83030);
#17805=VERTEX_POINT('',#83036);
#17806=VERTEX_POINT('',#83038);
#17807=VERTEX_POINT('',#83042);
#17808=VERTEX_POINT('',#83043);
#17809=VERTEX_POINT('',#83045);
#17810=VERTEX_POINT('',#83054);
#17811=VERTEX_POINT('',#83056);
#17812=VERTEX_POINT('',#83058);
#17813=VERTEX_POINT('',#83060);
#17814=VERTEX_POINT('',#83062);
#17815=VERTEX_POINT('',#83064);
#17816=VERTEX_POINT('',#83066);
#17817=VERTEX_POINT('',#83068);
#17818=VERTEX_POINT('',#83070);
#17819=VERTEX_POINT('',#83072);
#17820=VERTEX_POINT('',#83074);
#17821=VERTEX_POINT('',#83076);
#17822=VERTEX_POINT('',#83078);
#17823=VERTEX_POINT('',#83080);
#17824=VERTEX_POINT('',#83082);
#17825=VERTEX_POINT('',#83084);
#17826=VERTEX_POINT('',#83086);
#17827=VERTEX_POINT('',#83088);
#17828=VERTEX_POINT('',#83090);
#17829=VERTEX_POINT('',#83092);
#17830=VERTEX_POINT('',#83094);
#17831=VERTEX_POINT('',#83096);
#17832=VERTEX_POINT('',#83098);
#17833=VERTEX_POINT('',#83100);
#17834=VERTEX_POINT('',#83102);
#17835=VERTEX_POINT('',#83104);
#17836=VERTEX_POINT('',#83106);
#17837=VERTEX_POINT('',#83108);
#17838=VERTEX_POINT('',#83110);
#17839=VERTEX_POINT('',#83112);
#17840=VERTEX_POINT('',#83114);
#17841=VERTEX_POINT('',#83116);
#17842=VERTEX_POINT('',#83118);
#17843=VERTEX_POINT('',#83120);
#17844=VERTEX_POINT('',#83122);
#17845=VERTEX_POINT('',#83124);
#17846=VERTEX_POINT('',#83126);
#17847=VERTEX_POINT('',#83128);
#17848=VERTEX_POINT('',#83130);
#17849=VERTEX_POINT('',#83132);
#17850=VERTEX_POINT('',#83134);
#17851=VERTEX_POINT('',#83136);
#17852=VERTEX_POINT('',#83138);
#17853=VERTEX_POINT('',#83140);
#17854=VERTEX_POINT('',#83142);
#17855=VERTEX_POINT('',#83144);
#17856=VERTEX_POINT('',#83146);
#17857=VERTEX_POINT('',#83148);
#17858=VERTEX_POINT('',#83150);
#17859=VERTEX_POINT('',#83152);
#17860=VERTEX_POINT('',#83154);
#17861=VERTEX_POINT('',#83156);
#17862=VERTEX_POINT('',#83158);
#17863=VERTEX_POINT('',#83160);
#17864=VERTEX_POINT('',#83162);
#17865=VERTEX_POINT('',#83164);
#17866=VERTEX_POINT('',#83166);
#17867=VERTEX_POINT('',#83168);
#17868=VERTEX_POINT('',#83170);
#17869=VERTEX_POINT('',#83172);
#17870=VERTEX_POINT('',#83174);
#17871=VERTEX_POINT('',#83176);
#17872=VERTEX_POINT('',#83178);
#17873=VERTEX_POINT('',#83180);
#17874=VERTEX_POINT('',#83182);
#17875=VERTEX_POINT('',#83184);
#17876=VERTEX_POINT('',#83186);
#17877=VERTEX_POINT('',#83188);
#17878=VERTEX_POINT('',#83190);
#17879=VERTEX_POINT('',#83192);
#17880=VERTEX_POINT('',#83194);
#17881=VERTEX_POINT('',#83196);
#17882=VERTEX_POINT('',#83198);
#17883=VERTEX_POINT('',#83200);
#17884=VERTEX_POINT('',#83202);
#17885=VERTEX_POINT('',#83204);
#17886=VERTEX_POINT('',#83206);
#17887=VERTEX_POINT('',#83208);
#17888=VERTEX_POINT('',#83210);
#17889=VERTEX_POINT('',#83212);
#17890=VERTEX_POINT('',#83214);
#17891=VERTEX_POINT('',#83216);
#17892=VERTEX_POINT('',#83218);
#17893=VERTEX_POINT('',#83220);
#17894=VERTEX_POINT('',#83222);
#17895=VERTEX_POINT('',#83224);
#17896=VERTEX_POINT('',#83226);
#17897=VERTEX_POINT('',#83228);
#17898=VERTEX_POINT('',#83230);
#17899=VERTEX_POINT('',#83232);
#17900=VERTEX_POINT('',#83234);
#17901=VERTEX_POINT('',#83236);
#17902=VERTEX_POINT('',#83238);
#17903=VERTEX_POINT('',#83240);
#17904=VERTEX_POINT('',#83242);
#17905=VERTEX_POINT('',#83244);
#17906=VERTEX_POINT('',#83246);
#17907=VERTEX_POINT('',#83248);
#17908=VERTEX_POINT('',#83250);
#17909=VERTEX_POINT('',#83252);
#17910=VERTEX_POINT('',#83254);
#17911=VERTEX_POINT('',#83256);
#17912=VERTEX_POINT('',#83258);
#17913=VERTEX_POINT('',#83260);
#17914=VERTEX_POINT('',#83262);
#17915=VERTEX_POINT('',#83264);
#17916=VERTEX_POINT('',#83266);
#17917=VERTEX_POINT('',#83268);
#17918=VERTEX_POINT('',#83270);
#17919=VERTEX_POINT('',#83272);
#17920=VERTEX_POINT('',#83274);
#17921=VERTEX_POINT('',#83276);
#17922=VERTEX_POINT('',#83278);
#17923=VERTEX_POINT('',#83280);
#17924=VERTEX_POINT('',#83282);
#17925=VERTEX_POINT('',#83284);
#17926=VERTEX_POINT('',#83286);
#17927=VERTEX_POINT('',#83288);
#17928=VERTEX_POINT('',#83290);
#17929=VERTEX_POINT('',#83292);
#17930=VERTEX_POINT('',#83294);
#17931=VERTEX_POINT('',#83296);
#17932=VERTEX_POINT('',#83298);
#17933=VERTEX_POINT('',#83300);
#17934=VERTEX_POINT('',#83302);
#17935=VERTEX_POINT('',#83304);
#17936=VERTEX_POINT('',#83306);
#17937=VERTEX_POINT('',#83308);
#17938=VERTEX_POINT('',#83310);
#17939=VERTEX_POINT('',#83312);
#17940=VERTEX_POINT('',#83314);
#17941=VERTEX_POINT('',#83316);
#17942=VERTEX_POINT('',#83318);
#17943=VERTEX_POINT('',#83320);
#17944=VERTEX_POINT('',#83322);
#17945=VERTEX_POINT('',#83324);
#17946=VERTEX_POINT('',#83326);
#17947=VERTEX_POINT('',#83328);
#17948=VERTEX_POINT('',#83330);
#17949=VERTEX_POINT('',#83332);
#17950=VERTEX_POINT('',#83335);
#17951=VERTEX_POINT('',#83337);
#17952=VERTEX_POINT('',#83339);
#17953=VERTEX_POINT('',#83341);
#17954=VERTEX_POINT('',#83343);
#17955=VERTEX_POINT('',#83345);
#17956=VERTEX_POINT('',#83347);
#17957=VERTEX_POINT('',#83349);
#17958=VERTEX_POINT('',#83351);
#17959=VERTEX_POINT('',#83353);
#17960=VERTEX_POINT('',#83355);
#17961=VERTEX_POINT('',#83357);
#17962=VERTEX_POINT('',#83359);
#17963=VERTEX_POINT('',#83361);
#17964=VERTEX_POINT('',#83363);
#17965=VERTEX_POINT('',#83365);
#17966=VERTEX_POINT('',#83367);
#17967=VERTEX_POINT('',#83369);
#17968=VERTEX_POINT('',#83371);
#17969=VERTEX_POINT('',#83373);
#17970=VERTEX_POINT('',#83375);
#17971=VERTEX_POINT('',#83377);
#17972=VERTEX_POINT('',#83379);
#17973=VERTEX_POINT('',#83381);
#17974=VERTEX_POINT('',#83383);
#17975=VERTEX_POINT('',#83385);
#17976=VERTEX_POINT('',#83387);
#17977=VERTEX_POINT('',#83389);
#17978=VERTEX_POINT('',#83391);
#17979=VERTEX_POINT('',#83393);
#17980=VERTEX_POINT('',#83395);
#17981=VERTEX_POINT('',#83397);
#17982=VERTEX_POINT('',#83399);
#17983=VERTEX_POINT('',#83401);
#17984=VERTEX_POINT('',#83403);
#17985=VERTEX_POINT('',#83405);
#17986=VERTEX_POINT('',#83407);
#17987=VERTEX_POINT('',#83409);
#17988=VERTEX_POINT('',#83411);
#17989=VERTEX_POINT('',#83413);
#17990=VERTEX_POINT('',#83415);
#17991=VERTEX_POINT('',#83417);
#17992=VERTEX_POINT('',#83419);
#17993=VERTEX_POINT('',#83421);
#17994=VERTEX_POINT('',#83423);
#17995=VERTEX_POINT('',#83425);
#17996=VERTEX_POINT('',#83427);
#17997=VERTEX_POINT('',#83429);
#17998=VERTEX_POINT('',#83431);
#17999=VERTEX_POINT('',#83433);
#18000=VERTEX_POINT('',#83437);
#18001=VERTEX_POINT('',#83443);
#18002=VERTEX_POINT('',#83449);
#18003=VERTEX_POINT('',#83451);
#18004=VERTEX_POINT('',#83455);
#18005=VERTEX_POINT('',#83459);
#18006=VERTEX_POINT('',#83460);
#18007=VERTEX_POINT('',#83469);
#18008=VERTEX_POINT('',#83475);
#18009=VERTEX_POINT('',#83477);
#18010=VERTEX_POINT('',#83481);
#18011=VERTEX_POINT('',#83485);
#18012=VERTEX_POINT('',#83486);
#18013=VERTEX_POINT('',#83495);
#18014=VERTEX_POINT('',#83501);
#18015=VERTEX_POINT('',#83503);
#18016=VERTEX_POINT('',#83507);
#18017=VERTEX_POINT('',#83511);
#18018=VERTEX_POINT('',#83512);
#18019=VERTEX_POINT('',#83521);
#18020=VERTEX_POINT('',#83527);
#18021=VERTEX_POINT('',#83529);
#18022=VERTEX_POINT('',#83533);
#18023=VERTEX_POINT('',#83537);
#18024=VERTEX_POINT('',#83538);
#18025=VERTEX_POINT('',#83547);
#18026=VERTEX_POINT('',#83553);
#18027=VERTEX_POINT('',#83555);
#18028=VERTEX_POINT('',#83559);
#18029=VERTEX_POINT('',#83563);
#18030=VERTEX_POINT('',#83564);
#18031=VERTEX_POINT('',#83573);
#18032=VERTEX_POINT('',#83579);
#18033=VERTEX_POINT('',#83581);
#18034=VERTEX_POINT('',#83585);
#18035=VERTEX_POINT('',#83589);
#18036=VERTEX_POINT('',#83590);
#18037=VERTEX_POINT('',#83599);
#18038=VERTEX_POINT('',#83605);
#18039=VERTEX_POINT('',#83607);
#18040=VERTEX_POINT('',#83611);
#18041=VERTEX_POINT('',#83615);
#18042=VERTEX_POINT('',#83616);
#18043=VERTEX_POINT('',#83625);
#18044=VERTEX_POINT('',#83631);
#18045=VERTEX_POINT('',#83633);
#18046=VERTEX_POINT('',#83637);
#18047=VERTEX_POINT('',#83641);
#18048=VERTEX_POINT('',#83642);
#18049=VERTEX_POINT('',#83651);
#18050=VERTEX_POINT('',#83657);
#18051=VERTEX_POINT('',#83659);
#18052=VERTEX_POINT('',#83663);
#18053=VERTEX_POINT('',#83667);
#18054=VERTEX_POINT('',#83668);
#18055=VERTEX_POINT('',#83677);
#18056=VERTEX_POINT('',#83683);
#18057=VERTEX_POINT('',#83685);
#18058=VERTEX_POINT('',#83689);
#18059=VERTEX_POINT('',#83693);
#18060=VERTEX_POINT('',#83694);
#18061=VERTEX_POINT('',#83703);
#18062=VERTEX_POINT('',#83709);
#18063=VERTEX_POINT('',#83711);
#18064=VERTEX_POINT('',#83715);
#18065=VERTEX_POINT('',#83719);
#18066=VERTEX_POINT('',#83720);
#18067=VERTEX_POINT('',#83729);
#18068=VERTEX_POINT('',#83735);
#18069=VERTEX_POINT('',#83737);
#18070=VERTEX_POINT('',#83741);
#18071=VERTEX_POINT('',#83745);
#18072=VERTEX_POINT('',#83746);
#18073=VERTEX_POINT('',#83755);
#18074=VERTEX_POINT('',#83761);
#18075=VERTEX_POINT('',#83763);
#18076=VERTEX_POINT('',#83767);
#18077=VERTEX_POINT('',#83771);
#18078=VERTEX_POINT('',#83772);
#18079=VERTEX_POINT('',#83781);
#18080=VERTEX_POINT('',#83787);
#18081=VERTEX_POINT('',#83789);
#18082=VERTEX_POINT('',#83793);
#18083=VERTEX_POINT('',#83797);
#18084=VERTEX_POINT('',#83798);
#18085=VERTEX_POINT('',#83807);
#18086=VERTEX_POINT('',#83813);
#18087=VERTEX_POINT('',#83815);
#18088=VERTEX_POINT('',#83819);
#18089=VERTEX_POINT('',#83823);
#18090=VERTEX_POINT('',#83824);
#18091=VERTEX_POINT('',#83833);
#18092=VERTEX_POINT('',#83839);
#18093=VERTEX_POINT('',#83841);
#18094=VERTEX_POINT('',#83845);
#18095=VERTEX_POINT('',#83849);
#18096=VERTEX_POINT('',#83850);
#18097=VERTEX_POINT('',#83859);
#18098=VERTEX_POINT('',#83865);
#18099=VERTEX_POINT('',#83867);
#18100=VERTEX_POINT('',#83871);
#18101=VERTEX_POINT('',#83875);
#18102=VERTEX_POINT('',#83876);
#18103=VERTEX_POINT('',#83885);
#18104=VERTEX_POINT('',#83891);
#18105=VERTEX_POINT('',#83893);
#18106=VERTEX_POINT('',#83897);
#18107=VERTEX_POINT('',#83901);
#18108=VERTEX_POINT('',#83902);
#18109=VERTEX_POINT('',#83911);
#18110=VERTEX_POINT('',#83917);
#18111=VERTEX_POINT('',#83919);
#18112=VERTEX_POINT('',#83923);
#18113=VERTEX_POINT('',#83927);
#18114=VERTEX_POINT('',#83928);
#18115=VERTEX_POINT('',#83937);
#18116=VERTEX_POINT('',#83943);
#18117=VERTEX_POINT('',#83945);
#18118=VERTEX_POINT('',#83949);
#18119=VERTEX_POINT('',#83953);
#18120=VERTEX_POINT('',#83954);
#18121=VERTEX_POINT('',#83963);
#18122=VERTEX_POINT('',#83969);
#18123=VERTEX_POINT('',#83971);
#18124=VERTEX_POINT('',#83975);
#18125=VERTEX_POINT('',#83979);
#18126=VERTEX_POINT('',#83980);
#18127=VERTEX_POINT('',#83989);
#18128=VERTEX_POINT('',#83995);
#18129=VERTEX_POINT('',#83997);
#18130=VERTEX_POINT('',#84001);
#18131=VERTEX_POINT('',#84005);
#18132=VERTEX_POINT('',#84006);
#18133=VERTEX_POINT('',#84015);
#18134=VERTEX_POINT('',#84021);
#18135=VERTEX_POINT('',#84023);
#18136=VERTEX_POINT('',#84027);
#18137=VERTEX_POINT('',#84031);
#18138=VERTEX_POINT('',#84037);
#18139=VERTEX_POINT('',#84039);
#18140=VERTEX_POINT('',#84041);
#18141=VERTEX_POINT('',#84047);
#18142=VERTEX_POINT('',#84049);
#18143=VERTEX_POINT('',#84053);
#18144=VERTEX_POINT('',#84061);
#18145=VERTEX_POINT('',#84063);
#18146=VERTEX_POINT('',#84065);
#18147=VERTEX_POINT('',#84067);
#18148=VERTEX_POINT('',#84069);
#18149=VERTEX_POINT('',#84071);
#18150=VERTEX_POINT('',#84073);
#18151=VERTEX_POINT('',#84075);
#18152=VERTEX_POINT('',#84077);
#18153=VERTEX_POINT('',#84079);
#18154=VERTEX_POINT('',#84081);
#18155=VERTEX_POINT('',#84083);
#18156=VERTEX_POINT('',#84085);
#18157=VERTEX_POINT('',#84087);
#18158=VERTEX_POINT('',#84089);
#18159=VERTEX_POINT('',#84091);
#18160=VERTEX_POINT('',#84093);
#18161=VERTEX_POINT('',#84095);
#18162=VERTEX_POINT('',#84097);
#18163=VERTEX_POINT('',#84099);
#18164=VERTEX_POINT('',#84101);
#18165=VERTEX_POINT('',#84103);
#18166=VERTEX_POINT('',#84105);
#18167=VERTEX_POINT('',#84107);
#18168=VERTEX_POINT('',#84109);
#18169=VERTEX_POINT('',#84111);
#18170=VERTEX_POINT('',#84113);
#18171=VERTEX_POINT('',#84115);
#18172=VERTEX_POINT('',#84117);
#18173=VERTEX_POINT('',#84119);
#18174=VERTEX_POINT('',#84121);
#18175=VERTEX_POINT('',#84123);
#18176=VERTEX_POINT('',#84125);
#18177=VERTEX_POINT('',#84127);
#18178=VERTEX_POINT('',#84129);
#18179=VERTEX_POINT('',#84131);
#18180=VERTEX_POINT('',#84133);
#18181=VERTEX_POINT('',#84135);
#18182=VERTEX_POINT('',#84137);
#18183=VERTEX_POINT('',#84139);
#18184=VERTEX_POINT('',#84141);
#18185=VERTEX_POINT('',#84143);
#18186=VERTEX_POINT('',#84145);
#18187=VERTEX_POINT('',#84147);
#18188=VERTEX_POINT('',#84149);
#18189=VERTEX_POINT('',#84151);
#18190=VERTEX_POINT('',#84153);
#18191=VERTEX_POINT('',#84155);
#18192=VERTEX_POINT('',#84157);
#18193=VERTEX_POINT('',#84159);
#18194=VERTEX_POINT('',#84161);
#18195=VERTEX_POINT('',#84163);
#18196=VERTEX_POINT('',#84165);
#18197=VERTEX_POINT('',#84167);
#18198=VERTEX_POINT('',#84169);
#18199=VERTEX_POINT('',#84171);
#18200=VERTEX_POINT('',#84173);
#18201=VERTEX_POINT('',#84175);
#18202=VERTEX_POINT('',#84177);
#18203=VERTEX_POINT('',#84179);
#18204=VERTEX_POINT('',#84181);
#18205=VERTEX_POINT('',#84183);
#18206=VERTEX_POINT('',#84185);
#18207=VERTEX_POINT('',#84187);
#18208=VERTEX_POINT('',#84189);
#18209=VERTEX_POINT('',#84191);
#18210=VERTEX_POINT('',#84193);
#18211=VERTEX_POINT('',#84195);
#18212=VERTEX_POINT('',#84197);
#18213=VERTEX_POINT('',#84199);
#18214=VERTEX_POINT('',#84201);
#18215=VERTEX_POINT('',#84203);
#18216=VERTEX_POINT('',#84205);
#18217=VERTEX_POINT('',#84207);
#18218=VERTEX_POINT('',#84209);
#18219=VERTEX_POINT('',#84211);
#18220=VERTEX_POINT('',#84213);
#18221=VERTEX_POINT('',#84215);
#18222=VERTEX_POINT('',#84217);
#18223=VERTEX_POINT('',#84219);
#18224=VERTEX_POINT('',#84221);
#18225=VERTEX_POINT('',#84223);
#18226=VERTEX_POINT('',#84225);
#18227=VERTEX_POINT('',#84227);
#18228=VERTEX_POINT('',#84229);
#18229=VERTEX_POINT('',#84231);
#18230=VERTEX_POINT('',#84233);
#18231=VERTEX_POINT('',#84235);
#18232=VERTEX_POINT('',#84237);
#18233=VERTEX_POINT('',#84239);
#18234=VERTEX_POINT('',#84241);
#18235=VERTEX_POINT('',#84243);
#18236=VERTEX_POINT('',#84255);
#18237=VERTEX_POINT('',#84259);
#18238=VERTEX_POINT('',#84273);
#18239=VERTEX_POINT('',#84277);
#18240=VERTEX_POINT('',#84291);
#18241=VERTEX_POINT('',#84295);
#18242=VERTEX_POINT('',#84309);
#18243=VERTEX_POINT('',#84313);
#18244=VERTEX_POINT('',#84327);
#18245=VERTEX_POINT('',#84331);
#18246=VERTEX_POINT('',#84345);
#18247=VERTEX_POINT('',#84349);
#18248=VERTEX_POINT('',#84363);
#18249=VERTEX_POINT('',#84367);
#18250=VERTEX_POINT('',#84381);
#18251=VERTEX_POINT('',#84385);
#18252=VERTEX_POINT('',#84399);
#18253=VERTEX_POINT('',#84403);
#18254=VERTEX_POINT('',#84417);
#18255=VERTEX_POINT('',#84421);
#18256=VERTEX_POINT('',#84435);
#18257=VERTEX_POINT('',#84439);
#18258=VERTEX_POINT('',#84453);
#18259=VERTEX_POINT('',#84457);
#18260=VERTEX_POINT('',#84471);
#18261=VERTEX_POINT('',#84475);
#18262=VERTEX_POINT('',#84489);
#18263=VERTEX_POINT('',#84493);
#18264=VERTEX_POINT('',#84507);
#18265=VERTEX_POINT('',#84511);
#18266=VERTEX_POINT('',#84525);
#18267=VERTEX_POINT('',#84529);
#18268=VERTEX_POINT('',#84543);
#18269=VERTEX_POINT('',#84547);
#18270=VERTEX_POINT('',#84561);
#18271=VERTEX_POINT('',#84565);
#18272=VERTEX_POINT('',#84579);
#18273=VERTEX_POINT('',#84583);
#18274=VERTEX_POINT('',#84597);
#18275=VERTEX_POINT('',#84601);
#18276=VERTEX_POINT('',#84615);
#18277=VERTEX_POINT('',#84619);
#18278=VERTEX_POINT('',#84633);
#18279=VERTEX_POINT('',#84637);
#18280=VERTEX_POINT('',#84651);
#18281=VERTEX_POINT('',#84655);
#23187=EDGE_CURVE('',#17800,#17801,#11855,.T.);
#23188=EDGE_CURVE('',#17802,#17800,#11856,.T.);
#23189=EDGE_CURVE('',#17803,#17802,#11857,.T.);
#23190=EDGE_CURVE('',#17804,#17803,#11858,.T.);
#23191=EDGE_CURVE('',#17801,#17804,#1833,.T.);
#23192=EDGE_CURVE('',#17803,#17805,#8705,.T.);
#23193=EDGE_CURVE('',#17802,#17806,#11859,.T.);
#23194=EDGE_CURVE('',#17806,#17805,#11860,.T.);
#23195=EDGE_CURVE('',#17807,#17808,#11861,.T.);
#23196=EDGE_CURVE('',#17809,#17807,#1834,.T.);
#23197=EDGE_CURVE('',#17805,#17809,#11862,.T.);
#23198=EDGE_CURVE('',#17806,#17808,#11863,.T.);
#23199=EDGE_CURVE('',#17808,#17800,#11864,.T.);
#23200=EDGE_CURVE('',#17810,#17809,#8706,.T.);
#23201=EDGE_CURVE('',#17810,#17811,#11865,.T.);
#23202=EDGE_CURVE('',#17811,#17812,#8707,.T.);
#23203=EDGE_CURVE('',#17812,#17813,#11866,.T.);
#23204=EDGE_CURVE('',#17814,#17813,#8708,.T.);
#23205=EDGE_CURVE('',#17814,#17815,#11867,.T.);
#23206=EDGE_CURVE('',#17815,#17816,#8709,.T.);
#23207=EDGE_CURVE('',#17816,#17817,#11868,.T.);
#23208=EDGE_CURVE('',#17818,#17817,#8710,.T.);
#23209=EDGE_CURVE('',#17818,#17819,#11869,.T.);
#23210=EDGE_CURVE('',#17819,#17820,#8711,.T.);
#23211=EDGE_CURVE('',#17820,#17821,#11870,.T.);
#23212=EDGE_CURVE('',#17822,#17821,#8712,.T.);
#23213=EDGE_CURVE('',#17822,#17823,#11871,.T.);
#23214=EDGE_CURVE('',#17823,#17824,#8713,.T.);
#23215=EDGE_CURVE('',#17824,#17825,#11872,.T.);
#23216=EDGE_CURVE('',#17826,#17825,#8714,.T.);
#23217=EDGE_CURVE('',#17826,#17827,#11873,.T.);
#23218=EDGE_CURVE('',#17827,#17828,#8715,.T.);
#23219=EDGE_CURVE('',#17828,#17829,#11874,.T.);
#23220=EDGE_CURVE('',#17830,#17829,#8716,.T.);
#23221=EDGE_CURVE('',#17830,#17831,#11875,.T.);
#23222=EDGE_CURVE('',#17831,#17832,#8717,.T.);
#23223=EDGE_CURVE('',#17832,#17833,#11876,.T.);
#23224=EDGE_CURVE('',#17834,#17833,#8718,.T.);
#23225=EDGE_CURVE('',#17834,#17835,#11877,.T.);
#23226=EDGE_CURVE('',#17835,#17836,#8719,.T.);
#23227=EDGE_CURVE('',#17836,#17837,#11878,.T.);
#23228=EDGE_CURVE('',#17838,#17837,#8720,.T.);
#23229=EDGE_CURVE('',#17838,#17839,#11879,.T.);
#23230=EDGE_CURVE('',#17839,#17840,#8721,.T.);
#23231=EDGE_CURVE('',#17840,#17841,#11880,.T.);
#23232=EDGE_CURVE('',#17842,#17841,#8722,.T.);
#23233=EDGE_CURVE('',#17842,#17843,#11881,.T.);
#23234=EDGE_CURVE('',#17843,#17844,#8723,.T.);
#23235=EDGE_CURVE('',#17844,#17845,#11882,.T.);
#23236=EDGE_CURVE('',#17846,#17845,#8724,.T.);
#23237=EDGE_CURVE('',#17846,#17847,#11883,.T.);
#23238=EDGE_CURVE('',#17847,#17848,#8725,.T.);
#23239=EDGE_CURVE('',#17848,#17849,#11884,.T.);
#23240=EDGE_CURVE('',#17850,#17849,#8726,.T.);
#23241=EDGE_CURVE('',#17850,#17851,#11885,.T.);
#23242=EDGE_CURVE('',#17851,#17852,#8727,.T.);
#23243=EDGE_CURVE('',#17852,#17853,#11886,.T.);
#23244=EDGE_CURVE('',#17853,#17854,#8728,.T.);
#23245=EDGE_CURVE('',#17854,#17855,#11887,.T.);
#23246=EDGE_CURVE('',#17855,#17856,#8729,.T.);
#23247=EDGE_CURVE('',#17856,#17857,#11888,.T.);
#23248=EDGE_CURVE('',#17857,#17858,#8730,.T.);
#23249=EDGE_CURVE('',#17858,#17859,#11889,.T.);
#23250=EDGE_CURVE('',#17859,#17860,#8731,.T.);
#23251=EDGE_CURVE('',#17860,#17861,#11890,.T.);
#23252=EDGE_CURVE('',#17861,#17862,#8732,.T.);
#23253=EDGE_CURVE('',#17862,#17863,#11891,.T.);
#23254=EDGE_CURVE('',#17863,#17864,#8733,.T.);
#23255=EDGE_CURVE('',#17864,#17865,#11892,.T.);
#23256=EDGE_CURVE('',#17865,#17866,#8734,.T.);
#23257=EDGE_CURVE('',#17866,#17867,#11893,.T.);
#23258=EDGE_CURVE('',#17867,#17868,#8735,.T.);
#23259=EDGE_CURVE('',#17868,#17869,#11894,.T.);
#23260=EDGE_CURVE('',#17869,#17870,#8736,.T.);
#23261=EDGE_CURVE('',#17870,#17871,#11895,.T.);
#23262=EDGE_CURVE('',#17871,#17872,#8737,.T.);
#23263=EDGE_CURVE('',#17872,#17873,#11896,.T.);
#23264=EDGE_CURVE('',#17873,#17874,#8738,.T.);
#23265=EDGE_CURVE('',#17874,#17875,#11897,.T.);
#23266=EDGE_CURVE('',#17875,#17876,#8739,.T.);
#23267=EDGE_CURVE('',#17876,#17877,#11898,.T.);
#23268=EDGE_CURVE('',#17877,#17878,#8740,.T.);
#23269=EDGE_CURVE('',#17878,#17879,#11899,.T.);
#23270=EDGE_CURVE('',#17879,#17880,#8741,.T.);
#23271=EDGE_CURVE('',#17880,#17881,#11900,.T.);
#23272=EDGE_CURVE('',#17881,#17882,#8742,.T.);
#23273=EDGE_CURVE('',#17882,#17883,#11901,.T.);
#23274=EDGE_CURVE('',#17883,#17884,#8743,.T.);
#23275=EDGE_CURVE('',#17884,#17885,#11902,.T.);
#23276=EDGE_CURVE('',#17885,#17886,#8744,.T.);
#23277=EDGE_CURVE('',#17886,#17887,#11903,.T.);
#23278=EDGE_CURVE('',#17887,#17888,#8745,.T.);
#23279=EDGE_CURVE('',#17888,#17889,#11904,.T.);
#23280=EDGE_CURVE('',#17889,#17890,#8746,.T.);
#23281=EDGE_CURVE('',#17890,#17891,#11905,.T.);
#23282=EDGE_CURVE('',#17891,#17892,#8747,.T.);
#23283=EDGE_CURVE('',#17892,#17893,#11906,.T.);
#23284=EDGE_CURVE('',#17893,#17894,#8748,.T.);
#23285=EDGE_CURVE('',#17894,#17895,#11907,.T.);
#23286=EDGE_CURVE('',#17895,#17896,#8749,.T.);
#23287=EDGE_CURVE('',#17896,#17897,#11908,.T.);
#23288=EDGE_CURVE('',#17897,#17898,#8750,.T.);
#23289=EDGE_CURVE('',#17898,#17899,#11909,.T.);
#23290=EDGE_CURVE('',#17899,#17900,#8751,.T.);
#23291=EDGE_CURVE('',#17900,#17901,#11910,.T.);
#23292=EDGE_CURVE('',#17901,#17902,#8752,.T.);
#23293=EDGE_CURVE('',#17902,#17903,#11911,.T.);
#23294=EDGE_CURVE('',#17903,#17904,#8753,.T.);
#23295=EDGE_CURVE('',#17904,#17905,#11912,.T.);
#23296=EDGE_CURVE('',#17905,#17906,#8754,.T.);
#23297=EDGE_CURVE('',#17906,#17907,#11913,.T.);
#23298=EDGE_CURVE('',#17907,#17908,#8755,.T.);
#23299=EDGE_CURVE('',#17908,#17909,#11914,.T.);
#23300=EDGE_CURVE('',#17909,#17910,#8756,.T.);
#23301=EDGE_CURVE('',#17910,#17911,#11915,.T.);
#23302=EDGE_CURVE('',#17911,#17912,#8757,.T.);
#23303=EDGE_CURVE('',#17912,#17913,#11916,.T.);
#23304=EDGE_CURVE('',#17913,#17914,#8758,.T.);
#23305=EDGE_CURVE('',#17914,#17915,#11917,.T.);
#23306=EDGE_CURVE('',#17915,#17916,#8759,.T.);
#23307=EDGE_CURVE('',#17916,#17917,#11918,.T.);
#23308=EDGE_CURVE('',#17917,#17918,#8760,.T.);
#23309=EDGE_CURVE('',#17918,#17919,#11919,.T.);
#23310=EDGE_CURVE('',#17919,#17920,#8761,.T.);
#23311=EDGE_CURVE('',#17920,#17921,#11920,.T.);
#23312=EDGE_CURVE('',#17921,#17922,#8762,.T.);
#23313=EDGE_CURVE('',#17922,#17923,#11921,.T.);
#23314=EDGE_CURVE('',#17923,#17924,#8763,.T.);
#23315=EDGE_CURVE('',#17924,#17925,#11922,.T.);
#23316=EDGE_CURVE('',#17925,#17926,#8764,.T.);
#23317=EDGE_CURVE('',#17926,#17927,#11923,.T.);
#23318=EDGE_CURVE('',#17927,#17928,#8765,.T.);
#23319=EDGE_CURVE('',#17928,#17929,#11924,.T.);
#23320=EDGE_CURVE('',#17929,#17930,#8766,.T.);
#23321=EDGE_CURVE('',#17930,#17931,#11925,.T.);
#23322=EDGE_CURVE('',#17931,#17932,#8767,.T.);
#23323=EDGE_CURVE('',#17932,#17933,#11926,.T.);
#23324=EDGE_CURVE('',#17933,#17934,#8768,.T.);
#23325=EDGE_CURVE('',#17934,#17935,#11927,.T.);
#23326=EDGE_CURVE('',#17935,#17936,#8769,.T.);
#23327=EDGE_CURVE('',#17936,#17937,#11928,.T.);
#23328=EDGE_CURVE('',#17937,#17938,#8770,.T.);
#23329=EDGE_CURVE('',#17938,#17939,#11929,.T.);
#23330=EDGE_CURVE('',#17939,#17940,#8771,.T.);
#23331=EDGE_CURVE('',#17940,#17941,#11930,.T.);
#23332=EDGE_CURVE('',#17941,#17942,#8772,.T.);
#23333=EDGE_CURVE('',#17942,#17943,#11931,.T.);
#23334=EDGE_CURVE('',#17943,#17944,#8773,.T.);
#23335=EDGE_CURVE('',#17944,#17945,#11932,.T.);
#23336=EDGE_CURVE('',#17945,#17946,#8774,.T.);
#23337=EDGE_CURVE('',#17946,#17947,#11933,.T.);
#23338=EDGE_CURVE('',#17947,#17948,#8775,.T.);
#23339=EDGE_CURVE('',#17948,#17949,#11934,.T.);
#23340=EDGE_CURVE('',#17949,#17853,#8776,.T.);
#23341=EDGE_CURVE('',#17852,#17950,#8777,.T.);
#23342=EDGE_CURVE('',#17950,#17951,#11935,.T.);
#23343=EDGE_CURVE('',#17952,#17951,#8778,.T.);
#23344=EDGE_CURVE('',#17952,#17953,#11936,.T.);
#23345=EDGE_CURVE('',#17953,#17954,#8779,.T.);
#23346=EDGE_CURVE('',#17954,#17955,#11937,.T.);
#23347=EDGE_CURVE('',#17956,#17955,#8780,.T.);
#23348=EDGE_CURVE('',#17956,#17957,#11938,.T.);
#23349=EDGE_CURVE('',#17957,#17958,#8781,.T.);
#23350=EDGE_CURVE('',#17958,#17959,#11939,.T.);
#23351=EDGE_CURVE('',#17960,#17959,#8782,.T.);
#23352=EDGE_CURVE('',#17960,#17961,#11940,.T.);
#23353=EDGE_CURVE('',#17961,#17962,#8783,.T.);
#23354=EDGE_CURVE('',#17962,#17963,#11941,.T.);
#23355=EDGE_CURVE('',#17964,#17963,#8784,.T.);
#23356=EDGE_CURVE('',#17964,#17965,#11942,.T.);
#23357=EDGE_CURVE('',#17965,#17966,#8785,.T.);
#23358=EDGE_CURVE('',#17966,#17967,#11943,.T.);
#23359=EDGE_CURVE('',#17968,#17967,#8786,.T.);
#23360=EDGE_CURVE('',#17968,#17969,#11944,.T.);
#23361=EDGE_CURVE('',#17969,#17970,#8787,.T.);
#23362=EDGE_CURVE('',#17970,#17971,#11945,.T.);
#23363=EDGE_CURVE('',#17972,#17971,#8788,.T.);
#23364=EDGE_CURVE('',#17972,#17973,#11946,.T.);
#23365=EDGE_CURVE('',#17973,#17974,#8789,.T.);
#23366=EDGE_CURVE('',#17974,#17975,#11947,.T.);
#23367=EDGE_CURVE('',#17976,#17975,#8790,.T.);
#23368=EDGE_CURVE('',#17976,#17977,#11948,.T.);
#23369=EDGE_CURVE('',#17977,#17978,#8791,.T.);
#23370=EDGE_CURVE('',#17978,#17979,#11949,.T.);
#23371=EDGE_CURVE('',#17980,#17979,#8792,.T.);
#23372=EDGE_CURVE('',#17980,#17981,#11950,.T.);
#23373=EDGE_CURVE('',#17981,#17982,#8793,.T.);
#23374=EDGE_CURVE('',#17982,#17983,#11951,.T.);
#23375=EDGE_CURVE('',#17984,#17983,#8794,.T.);
#23376=EDGE_CURVE('',#17984,#17985,#11952,.T.);
#23377=EDGE_CURVE('',#17985,#17986,#8795,.T.);
#23378=EDGE_CURVE('',#17986,#17987,#11953,.T.);
#23379=EDGE_CURVE('',#17988,#17987,#8796,.T.);
#23380=EDGE_CURVE('',#17988,#17989,#11954,.T.);
#23381=EDGE_CURVE('',#17989,#17990,#8797,.T.);
#23382=EDGE_CURVE('',#17990,#17991,#11955,.T.);
#23383=EDGE_CURVE('',#17992,#17991,#8798,.T.);
#23384=EDGE_CURVE('',#17992,#17993,#11956,.T.);
#23385=EDGE_CURVE('',#17993,#17994,#8799,.T.);
#23386=EDGE_CURVE('',#17994,#17995,#11957,.T.);
#23387=EDGE_CURVE('',#17996,#17995,#8800,.T.);
#23388=EDGE_CURVE('',#17996,#17997,#11958,.T.);
#23389=EDGE_CURVE('',#17997,#17998,#8801,.T.);
#23390=EDGE_CURVE('',#17998,#17999,#11959,.T.);
#23391=EDGE_CURVE('',#17804,#17999,#8802,.T.);
#23392=EDGE_CURVE('',#18000,#17807,#8803,.T.);
#23393=EDGE_CURVE('',#18000,#17810,#1835,.T.);
#23394=EDGE_CURVE('',#17999,#18001,#1836,.T.);
#23395=EDGE_CURVE('',#17801,#18001,#8804,.T.);
#23396=EDGE_CURVE('',#18002,#18000,#11960,.T.);
#23397=EDGE_CURVE('',#18003,#18002,#11961,.T.);
#23398=EDGE_CURVE('',#17811,#18003,#11962,.T.);
#23399=EDGE_CURVE('',#18003,#18004,#11963,.T.);
#23400=EDGE_CURVE('',#18004,#17812,#11964,.T.);
#23401=EDGE_CURVE('',#18005,#18006,#11965,.T.);
#23402=EDGE_CURVE('',#17813,#18005,#1837,.T.);
#23403=EDGE_CURVE('',#18004,#18006,#11966,.T.);
#23404=EDGE_CURVE('',#18006,#18002,#11967,.T.);
#23405=EDGE_CURVE('',#18007,#18005,#8805,.T.);
#23406=EDGE_CURVE('',#18007,#17814,#1838,.T.);
#23407=EDGE_CURVE('',#18008,#18007,#11968,.T.);
#23408=EDGE_CURVE('',#18009,#18008,#11969,.T.);
#23409=EDGE_CURVE('',#17815,#18009,#11970,.T.);
#23410=EDGE_CURVE('',#18009,#18010,#11971,.T.);
#23411=EDGE_CURVE('',#18010,#17816,#11972,.T.);
#23412=EDGE_CURVE('',#18011,#18012,#11973,.T.);
#23413=EDGE_CURVE('',#17817,#18011,#1839,.T.);
#23414=EDGE_CURVE('',#18010,#18012,#11974,.T.);
#23415=EDGE_CURVE('',#18012,#18008,#11975,.T.);
#23416=EDGE_CURVE('',#18013,#18011,#8806,.T.);
#23417=EDGE_CURVE('',#18013,#17818,#1840,.T.);
#23418=EDGE_CURVE('',#18014,#18013,#11976,.T.);
#23419=EDGE_CURVE('',#18015,#18014,#11977,.T.);
#23420=EDGE_CURVE('',#17819,#18015,#11978,.T.);
#23421=EDGE_CURVE('',#18015,#18016,#11979,.T.);
#23422=EDGE_CURVE('',#18016,#17820,#11980,.T.);
#23423=EDGE_CURVE('',#18017,#18018,#11981,.T.);
#23424=EDGE_CURVE('',#17821,#18017,#1841,.T.);
#23425=EDGE_CURVE('',#18016,#18018,#11982,.T.);
#23426=EDGE_CURVE('',#18018,#18014,#11983,.T.);
#23427=EDGE_CURVE('',#18019,#18017,#8807,.T.);
#23428=EDGE_CURVE('',#18019,#17822,#1842,.T.);
#23429=EDGE_CURVE('',#18020,#18019,#11984,.T.);
#23430=EDGE_CURVE('',#18021,#18020,#11985,.T.);
#23431=EDGE_CURVE('',#17823,#18021,#11986,.T.);
#23432=EDGE_CURVE('',#18021,#18022,#11987,.T.);
#23433=EDGE_CURVE('',#18022,#17824,#11988,.T.);
#23434=EDGE_CURVE('',#18023,#18024,#11989,.T.);
#23435=EDGE_CURVE('',#17825,#18023,#1843,.T.);
#23436=EDGE_CURVE('',#18022,#18024,#11990,.T.);
#23437=EDGE_CURVE('',#18024,#18020,#11991,.T.);
#23438=EDGE_CURVE('',#18025,#18023,#8808,.T.);
#23439=EDGE_CURVE('',#18025,#17826,#1844,.T.);
#23440=EDGE_CURVE('',#18026,#18025,#11992,.T.);
#23441=EDGE_CURVE('',#18027,#18026,#11993,.T.);
#23442=EDGE_CURVE('',#17827,#18027,#11994,.T.);
#23443=EDGE_CURVE('',#18027,#18028,#11995,.T.);
#23444=EDGE_CURVE('',#18028,#17828,#11996,.T.);
#23445=EDGE_CURVE('',#18029,#18030,#11997,.T.);
#23446=EDGE_CURVE('',#17829,#18029,#1845,.T.);
#23447=EDGE_CURVE('',#18028,#18030,#11998,.T.);
#23448=EDGE_CURVE('',#18030,#18026,#11999,.T.);
#23449=EDGE_CURVE('',#18031,#18029,#8809,.T.);
#23450=EDGE_CURVE('',#18031,#17830,#1846,.T.);
#23451=EDGE_CURVE('',#18032,#18031,#12000,.T.);
#23452=EDGE_CURVE('',#18033,#18032,#12001,.T.);
#23453=EDGE_CURVE('',#17831,#18033,#12002,.T.);
#23454=EDGE_CURVE('',#18033,#18034,#12003,.T.);
#23455=EDGE_CURVE('',#18034,#17832,#12004,.T.);
#23456=EDGE_CURVE('',#18035,#18036,#12005,.T.);
#23457=EDGE_CURVE('',#17833,#18035,#1847,.T.);
#23458=EDGE_CURVE('',#18034,#18036,#12006,.T.);
#23459=EDGE_CURVE('',#18036,#18032,#12007,.T.);
#23460=EDGE_CURVE('',#18037,#18035,#8810,.T.);
#23461=EDGE_CURVE('',#18037,#17834,#1848,.T.);
#23462=EDGE_CURVE('',#18038,#18037,#12008,.T.);
#23463=EDGE_CURVE('',#18039,#18038,#12009,.T.);
#23464=EDGE_CURVE('',#17835,#18039,#12010,.T.);
#23465=EDGE_CURVE('',#18039,#18040,#12011,.T.);
#23466=EDGE_CURVE('',#18040,#17836,#12012,.T.);
#23467=EDGE_CURVE('',#18041,#18042,#12013,.T.);
#23468=EDGE_CURVE('',#17837,#18041,#1849,.T.);
#23469=EDGE_CURVE('',#18040,#18042,#12014,.T.);
#23470=EDGE_CURVE('',#18042,#18038,#12015,.T.);
#23471=EDGE_CURVE('',#18043,#18041,#8811,.T.);
#23472=EDGE_CURVE('',#18043,#17838,#1850,.T.);
#23473=EDGE_CURVE('',#18044,#18043,#12016,.T.);
#23474=EDGE_CURVE('',#18045,#18044,#12017,.T.);
#23475=EDGE_CURVE('',#17839,#18045,#12018,.T.);
#23476=EDGE_CURVE('',#18045,#18046,#12019,.T.);
#23477=EDGE_CURVE('',#18046,#17840,#12020,.T.);
#23478=EDGE_CURVE('',#18047,#18048,#12021,.T.);
#23479=EDGE_CURVE('',#17841,#18047,#1851,.T.);
#23480=EDGE_CURVE('',#18046,#18048,#12022,.T.);
#23481=EDGE_CURVE('',#18048,#18044,#12023,.T.);
#23482=EDGE_CURVE('',#18049,#18047,#8812,.T.);
#23483=EDGE_CURVE('',#18049,#17842,#1852,.T.);
#23484=EDGE_CURVE('',#18050,#18049,#12024,.T.);
#23485=EDGE_CURVE('',#18051,#18050,#12025,.T.);
#23486=EDGE_CURVE('',#17843,#18051,#12026,.T.);
#23487=EDGE_CURVE('',#18051,#18052,#12027,.T.);
#23488=EDGE_CURVE('',#18052,#17844,#12028,.T.);
#23489=EDGE_CURVE('',#18053,#18054,#12029,.T.);
#23490=EDGE_CURVE('',#17845,#18053,#1853,.T.);
#23491=EDGE_CURVE('',#18052,#18054,#12030,.T.);
#23492=EDGE_CURVE('',#18054,#18050,#12031,.T.);
#23493=EDGE_CURVE('',#18055,#18053,#8813,.T.);
#23494=EDGE_CURVE('',#18055,#17846,#1854,.T.);
#23495=EDGE_CURVE('',#18056,#18055,#12032,.T.);
#23496=EDGE_CURVE('',#18057,#18056,#12033,.T.);
#23497=EDGE_CURVE('',#17847,#18057,#12034,.T.);
#23498=EDGE_CURVE('',#18057,#18058,#12035,.T.);
#23499=EDGE_CURVE('',#18058,#17848,#12036,.T.);
#23500=EDGE_CURVE('',#18059,#18060,#12037,.T.);
#23501=EDGE_CURVE('',#17849,#18059,#1855,.T.);
#23502=EDGE_CURVE('',#18058,#18060,#12038,.T.);
#23503=EDGE_CURVE('',#18060,#18056,#12039,.T.);
#23504=EDGE_CURVE('',#18061,#18059,#8814,.T.);
#23505=EDGE_CURVE('',#18061,#17850,#1856,.T.);
#23506=EDGE_CURVE('',#18062,#18061,#12040,.T.);
#23507=EDGE_CURVE('',#18063,#18062,#12041,.T.);
#23508=EDGE_CURVE('',#17851,#18063,#12042,.T.);
#23509=EDGE_CURVE('',#18063,#18064,#12043,.T.);
#23510=EDGE_CURVE('',#18064,#17950,#12044,.T.);
#23511=EDGE_CURVE('',#18065,#18066,#12045,.T.);
#23512=EDGE_CURVE('',#17951,#18065,#1857,.T.);
#23513=EDGE_CURVE('',#18064,#18066,#12046,.T.);
#23514=EDGE_CURVE('',#18066,#18062,#12047,.T.);
#23515=EDGE_CURVE('',#18067,#18065,#8815,.T.);
#23516=EDGE_CURVE('',#18067,#17952,#1858,.T.);
#23517=EDGE_CURVE('',#18068,#18067,#12048,.T.);
#23518=EDGE_CURVE('',#18069,#18068,#12049,.T.);
#23519=EDGE_CURVE('',#17953,#18069,#12050,.T.);
#23520=EDGE_CURVE('',#18069,#18070,#12051,.T.);
#23521=EDGE_CURVE('',#18070,#17954,#12052,.T.);
#23522=EDGE_CURVE('',#18071,#18072,#12053,.T.);
#23523=EDGE_CURVE('',#17955,#18071,#1859,.T.);
#23524=EDGE_CURVE('',#18070,#18072,#12054,.T.);
#23525=EDGE_CURVE('',#18072,#18068,#12055,.T.);
#23526=EDGE_CURVE('',#18073,#18071,#8816,.T.);
#23527=EDGE_CURVE('',#18073,#17956,#1860,.T.);
#23528=EDGE_CURVE('',#18074,#18073,#12056,.T.);
#23529=EDGE_CURVE('',#18075,#18074,#12057,.T.);
#23530=EDGE_CURVE('',#17957,#18075,#12058,.T.);
#23531=EDGE_CURVE('',#18075,#18076,#12059,.T.);
#23532=EDGE_CURVE('',#18076,#17958,#12060,.T.);
#23533=EDGE_CURVE('',#18077,#18078,#12061,.T.);
#23534=EDGE_CURVE('',#17959,#18077,#1861,.T.);
#23535=EDGE_CURVE('',#18076,#18078,#12062,.T.);
#23536=EDGE_CURVE('',#18078,#18074,#12063,.T.);
#23537=EDGE_CURVE('',#18079,#18077,#8817,.T.);
#23538=EDGE_CURVE('',#18079,#17960,#1862,.T.);
#23539=EDGE_CURVE('',#18080,#18079,#12064,.T.);
#23540=EDGE_CURVE('',#18081,#18080,#12065,.T.);
#23541=EDGE_CURVE('',#17961,#18081,#12066,.T.);
#23542=EDGE_CURVE('',#18081,#18082,#12067,.T.);
#23543=EDGE_CURVE('',#18082,#17962,#12068,.T.);
#23544=EDGE_CURVE('',#18083,#18084,#12069,.T.);
#23545=EDGE_CURVE('',#17963,#18083,#1863,.T.);
#23546=EDGE_CURVE('',#18082,#18084,#12070,.T.);
#23547=EDGE_CURVE('',#18084,#18080,#12071,.T.);
#23548=EDGE_CURVE('',#18085,#18083,#8818,.T.);
#23549=EDGE_CURVE('',#18085,#17964,#1864,.T.);
#23550=EDGE_CURVE('',#18086,#18085,#12072,.T.);
#23551=EDGE_CURVE('',#18087,#18086,#12073,.T.);
#23552=EDGE_CURVE('',#17965,#18087,#12074,.T.);
#23553=EDGE_CURVE('',#18087,#18088,#12075,.T.);
#23554=EDGE_CURVE('',#18088,#17966,#12076,.T.);
#23555=EDGE_CURVE('',#18089,#18090,#12077,.T.);
#23556=EDGE_CURVE('',#17967,#18089,#1865,.T.);
#23557=EDGE_CURVE('',#18088,#18090,#12078,.T.);
#23558=EDGE_CURVE('',#18090,#18086,#12079,.T.);
#23559=EDGE_CURVE('',#18091,#18089,#8819,.T.);
#23560=EDGE_CURVE('',#18091,#17968,#1866,.T.);
#23561=EDGE_CURVE('',#18092,#18091,#12080,.T.);
#23562=EDGE_CURVE('',#18093,#18092,#12081,.T.);
#23563=EDGE_CURVE('',#17969,#18093,#12082,.T.);
#23564=EDGE_CURVE('',#18093,#18094,#12083,.T.);
#23565=EDGE_CURVE('',#18094,#17970,#12084,.T.);
#23566=EDGE_CURVE('',#18095,#18096,#12085,.T.);
#23567=EDGE_CURVE('',#17971,#18095,#1867,.T.);
#23568=EDGE_CURVE('',#18094,#18096,#12086,.T.);
#23569=EDGE_CURVE('',#18096,#18092,#12087,.T.);
#23570=EDGE_CURVE('',#18097,#18095,#8820,.T.);
#23571=EDGE_CURVE('',#18097,#17972,#1868,.T.);
#23572=EDGE_CURVE('',#18098,#18097,#12088,.T.);
#23573=EDGE_CURVE('',#18099,#18098,#12089,.T.);
#23574=EDGE_CURVE('',#17973,#18099,#12090,.T.);
#23575=EDGE_CURVE('',#18099,#18100,#12091,.T.);
#23576=EDGE_CURVE('',#18100,#17974,#12092,.T.);
#23577=EDGE_CURVE('',#18101,#18102,#12093,.T.);
#23578=EDGE_CURVE('',#17975,#18101,#1869,.T.);
#23579=EDGE_CURVE('',#18100,#18102,#12094,.T.);
#23580=EDGE_CURVE('',#18102,#18098,#12095,.T.);
#23581=EDGE_CURVE('',#18103,#18101,#8821,.T.);
#23582=EDGE_CURVE('',#18103,#17976,#1870,.T.);
#23583=EDGE_CURVE('',#18104,#18103,#12096,.T.);
#23584=EDGE_CURVE('',#18105,#18104,#12097,.T.);
#23585=EDGE_CURVE('',#17977,#18105,#12098,.T.);
#23586=EDGE_CURVE('',#18105,#18106,#12099,.T.);
#23587=EDGE_CURVE('',#18106,#17978,#12100,.T.);
#23588=EDGE_CURVE('',#18107,#18108,#12101,.T.);
#23589=EDGE_CURVE('',#17979,#18107,#1871,.T.);
#23590=EDGE_CURVE('',#18106,#18108,#12102,.T.);
#23591=EDGE_CURVE('',#18108,#18104,#12103,.T.);
#23592=EDGE_CURVE('',#18109,#18107,#8822,.T.);
#23593=EDGE_CURVE('',#18109,#17980,#1872,.T.);
#23594=EDGE_CURVE('',#18110,#18109,#12104,.T.);
#23595=EDGE_CURVE('',#18111,#18110,#12105,.T.);
#23596=EDGE_CURVE('',#17981,#18111,#12106,.T.);
#23597=EDGE_CURVE('',#18111,#18112,#12107,.T.);
#23598=EDGE_CURVE('',#18112,#17982,#12108,.T.);
#23599=EDGE_CURVE('',#18113,#18114,#12109,.T.);
#23600=EDGE_CURVE('',#17983,#18113,#1873,.T.);
#23601=EDGE_CURVE('',#18112,#18114,#12110,.T.);
#23602=EDGE_CURVE('',#18114,#18110,#12111,.T.);
#23603=EDGE_CURVE('',#18115,#18113,#8823,.T.);
#23604=EDGE_CURVE('',#18115,#17984,#1874,.T.);
#23605=EDGE_CURVE('',#18116,#18115,#12112,.T.);
#23606=EDGE_CURVE('',#18117,#18116,#12113,.T.);
#23607=EDGE_CURVE('',#17985,#18117,#12114,.T.);
#23608=EDGE_CURVE('',#18117,#18118,#12115,.T.);
#23609=EDGE_CURVE('',#18118,#17986,#12116,.T.);
#23610=EDGE_CURVE('',#18119,#18120,#12117,.T.);
#23611=EDGE_CURVE('',#17987,#18119,#1875,.T.);
#23612=EDGE_CURVE('',#18118,#18120,#12118,.T.);
#23613=EDGE_CURVE('',#18120,#18116,#12119,.T.);
#23614=EDGE_CURVE('',#18121,#18119,#8824,.T.);
#23615=EDGE_CURVE('',#18121,#17988,#1876,.T.);
#23616=EDGE_CURVE('',#18122,#18121,#12120,.T.);
#23617=EDGE_CURVE('',#18123,#18122,#12121,.T.);
#23618=EDGE_CURVE('',#17989,#18123,#12122,.T.);
#23619=EDGE_CURVE('',#18123,#18124,#12123,.T.);
#23620=EDGE_CURVE('',#18124,#17990,#12124,.T.);
#23621=EDGE_CURVE('',#18125,#18126,#12125,.T.);
#23622=EDGE_CURVE('',#17991,#18125,#1877,.T.);
#23623=EDGE_CURVE('',#18124,#18126,#12126,.T.);
#23624=EDGE_CURVE('',#18126,#18122,#12127,.T.);
#23625=EDGE_CURVE('',#18127,#18125,#8825,.T.);
#23626=EDGE_CURVE('',#18127,#17992,#1878,.T.);
#23627=EDGE_CURVE('',#18128,#18127,#12128,.T.);
#23628=EDGE_CURVE('',#18129,#18128,#12129,.T.);
#23629=EDGE_CURVE('',#17993,#18129,#12130,.T.);
#23630=EDGE_CURVE('',#18129,#18130,#12131,.T.);
#23631=EDGE_CURVE('',#18130,#17994,#12132,.T.);
#23632=EDGE_CURVE('',#18131,#18132,#12133,.T.);
#23633=EDGE_CURVE('',#17995,#18131,#1879,.T.);
#23634=EDGE_CURVE('',#18130,#18132,#12134,.T.);
#23635=EDGE_CURVE('',#18132,#18128,#12135,.T.);
#23636=EDGE_CURVE('',#18133,#18131,#8826,.T.);
#23637=EDGE_CURVE('',#18133,#17996,#1880,.T.);
#23638=EDGE_CURVE('',#18134,#18133,#12136,.T.);
#23639=EDGE_CURVE('',#18135,#18134,#12137,.T.);
#23640=EDGE_CURVE('',#17997,#18135,#12138,.T.);
#23641=EDGE_CURVE('',#18135,#18136,#12139,.T.);
#23642=EDGE_CURVE('',#18136,#17998,#12140,.T.);
#23643=EDGE_CURVE('',#18001,#18137,#12141,.T.);
#23644=EDGE_CURVE('',#18136,#18137,#12142,.T.);
#23645=EDGE_CURVE('',#18137,#18134,#12143,.T.);
#23646=EDGE_CURVE('',#17898,#18138,#12144,.T.);
#23647=EDGE_CURVE('',#18139,#18138,#12145,.T.);
#23648=EDGE_CURVE('',#18140,#18139,#12146,.T.);
#23649=EDGE_CURVE('',#17899,#18140,#1881,.T.);
#23650=EDGE_CURVE('',#18139,#18141,#12147,.T.);
#23651=EDGE_CURVE('',#18138,#18142,#12148,.T.);
#23652=EDGE_CURVE('',#18141,#18142,#12149,.T.);
#23653=EDGE_CURVE('',#18143,#17896,#1882,.T.);
#23654=EDGE_CURVE('',#18141,#18143,#12150,.T.);
#23655=EDGE_CURVE('',#18142,#17897,#12151,.T.);
#23656=EDGE_CURVE('',#18144,#18143,#8827,.T.);
#23657=EDGE_CURVE('',#18144,#18145,#12152,.T.);
#23658=EDGE_CURVE('',#18145,#18146,#12153,.T.);
#23659=EDGE_CURVE('',#18146,#18147,#12154,.T.);
#23660=EDGE_CURVE('',#18148,#18147,#8828,.T.);
#23661=EDGE_CURVE('',#18148,#18149,#12155,.T.);
#23662=EDGE_CURVE('',#18149,#18150,#12156,.T.);
#23663=EDGE_CURVE('',#18150,#18151,#12157,.T.);
#23664=EDGE_CURVE('',#18152,#18151,#8829,.T.);
#23665=EDGE_CURVE('',#18152,#18153,#12158,.T.);
#23666=EDGE_CURVE('',#18153,#18154,#12159,.T.);
#23667=EDGE_CURVE('',#18154,#18155,#12160,.T.);
#23668=EDGE_CURVE('',#18156,#18155,#8830,.T.);
#23669=EDGE_CURVE('',#18156,#18157,#12161,.T.);
#23670=EDGE_CURVE('',#18157,#18158,#12162,.T.);
#23671=EDGE_CURVE('',#18158,#18159,#12163,.T.);
#23672=EDGE_CURVE('',#18160,#18159,#8831,.T.);
#23673=EDGE_CURVE('',#18160,#18161,#12164,.T.);
#23674=EDGE_CURVE('',#18161,#18162,#12165,.T.);
#23675=EDGE_CURVE('',#18162,#18163,#12166,.T.);
#23676=EDGE_CURVE('',#18164,#18163,#8832,.T.);
#23677=EDGE_CURVE('',#18164,#18165,#12167,.T.);
#23678=EDGE_CURVE('',#18165,#18166,#12168,.T.);
#23679=EDGE_CURVE('',#18166,#18167,#12169,.T.);
#23680=EDGE_CURVE('',#18168,#18167,#8833,.T.);
#23681=EDGE_CURVE('',#18168,#18169,#12170,.T.);
#23682=EDGE_CURVE('',#18169,#18170,#12171,.T.);
#23683=EDGE_CURVE('',#18170,#18171,#12172,.T.);
#23684=EDGE_CURVE('',#18172,#18171,#8834,.T.);
#23685=EDGE_CURVE('',#18172,#18173,#12173,.T.);
#23686=EDGE_CURVE('',#18173,#18174,#12174,.T.);
#23687=EDGE_CURVE('',#18174,#18175,#12175,.T.);
#23688=EDGE_CURVE('',#18176,#18175,#8835,.T.);
#23689=EDGE_CURVE('',#18176,#18177,#12176,.T.);
#23690=EDGE_CURVE('',#18177,#18178,#12177,.T.);
#23691=EDGE_CURVE('',#18178,#18179,#12178,.T.);
#23692=EDGE_CURVE('',#18180,#18179,#8836,.T.);
#23693=EDGE_CURVE('',#18180,#18181,#12179,.T.);
#23694=EDGE_CURVE('',#18181,#18182,#12180,.T.);
#23695=EDGE_CURVE('',#18182,#18183,#12181,.T.);
#23696=EDGE_CURVE('',#18184,#18183,#8837,.T.);
#23697=EDGE_CURVE('',#18184,#18185,#12182,.T.);
#23698=EDGE_CURVE('',#18185,#18186,#12183,.T.);
#23699=EDGE_CURVE('',#18186,#18187,#12184,.T.);
#23700=EDGE_CURVE('',#18188,#18187,#8838,.T.);
#23701=EDGE_CURVE('',#18188,#18189,#12185,.T.);
#23702=EDGE_CURVE('',#18189,#18190,#12186,.T.);
#23703=EDGE_CURVE('',#18190,#18191,#12187,.T.);
#23704=EDGE_CURVE('',#18192,#18191,#8839,.T.);
#23705=EDGE_CURVE('',#18192,#18193,#12188,.T.);
#23706=EDGE_CURVE('',#18193,#18194,#12189,.T.);
#23707=EDGE_CURVE('',#18194,#18195,#12190,.T.);
#23708=EDGE_CURVE('',#18196,#18195,#8840,.T.);
#23709=EDGE_CURVE('',#18196,#18197,#12191,.T.);
#23710=EDGE_CURVE('',#18197,#18198,#12192,.T.);
#23711=EDGE_CURVE('',#18198,#18199,#12193,.T.);
#23712=EDGE_CURVE('',#18200,#18199,#8841,.T.);
#23713=EDGE_CURVE('',#18200,#18201,#12194,.T.);
#23714=EDGE_CURVE('',#18201,#18202,#12195,.T.);
#23715=EDGE_CURVE('',#18202,#18203,#12196,.T.);
#23716=EDGE_CURVE('',#18204,#18203,#8842,.T.);
#23717=EDGE_CURVE('',#18204,#18205,#12197,.T.);
#23718=EDGE_CURVE('',#18205,#18206,#12198,.T.);
#23719=EDGE_CURVE('',#18206,#18207,#12199,.T.);
#23720=EDGE_CURVE('',#18208,#18207,#8843,.T.);
#23721=EDGE_CURVE('',#18208,#18209,#12200,.T.);
#23722=EDGE_CURVE('',#18209,#18210,#12201,.T.);
#23723=EDGE_CURVE('',#18210,#18211,#12202,.T.);
#23724=EDGE_CURVE('',#18212,#18211,#8844,.T.);
#23725=EDGE_CURVE('',#18212,#18213,#12203,.T.);
#23726=EDGE_CURVE('',#18213,#18214,#12204,.T.);
#23727=EDGE_CURVE('',#18214,#18215,#12205,.T.);
#23728=EDGE_CURVE('',#18216,#18215,#8845,.T.);
#23729=EDGE_CURVE('',#18216,#18217,#12206,.T.);
#23730=EDGE_CURVE('',#18217,#18218,#12207,.T.);
#23731=EDGE_CURVE('',#18218,#18219,#12208,.T.);
#23732=EDGE_CURVE('',#18220,#18219,#8846,.T.);
#23733=EDGE_CURVE('',#18220,#18221,#12209,.T.);
#23734=EDGE_CURVE('',#18221,#18222,#12210,.T.);
#23735=EDGE_CURVE('',#18222,#18223,#12211,.T.);
#23736=EDGE_CURVE('',#18224,#18223,#8847,.T.);
#23737=EDGE_CURVE('',#18224,#18225,#12212,.T.);
#23738=EDGE_CURVE('',#18225,#18226,#12213,.T.);
#23739=EDGE_CURVE('',#18226,#18227,#12214,.T.);
#23740=EDGE_CURVE('',#18228,#18227,#8848,.T.);
#23741=EDGE_CURVE('',#18228,#18229,#12215,.T.);
#23742=EDGE_CURVE('',#18229,#18230,#12216,.T.);
#23743=EDGE_CURVE('',#18230,#18231,#12217,.T.);
#23744=EDGE_CURVE('',#18232,#18231,#8849,.T.);
#23745=EDGE_CURVE('',#18232,#18233,#12218,.T.);
#23746=EDGE_CURVE('',#18233,#18234,#12219,.T.);
#23747=EDGE_CURVE('',#18234,#18235,#12220,.T.);
#23748=EDGE_CURVE('',#18140,#18235,#8850,.T.);
#23749=EDGE_CURVE('',#17895,#18144,#1883,.T.);
#23750=EDGE_CURVE('',#18235,#17900,#1884,.T.);
#23751=EDGE_CURVE('',#17894,#18236,#12221,.T.);
#23752=EDGE_CURVE('',#18145,#18236,#12222,.T.);
#23753=EDGE_CURVE('',#18236,#18237,#12223,.T.);
#23754=EDGE_CURVE('',#18146,#18237,#12224,.T.);
#23755=EDGE_CURVE('',#18147,#17892,#1885,.T.);
#23756=EDGE_CURVE('',#18237,#17893,#12225,.T.);
#23757=EDGE_CURVE('',#17891,#18148,#1886,.T.);
#23758=EDGE_CURVE('',#17890,#18238,#12226,.T.);
#23759=EDGE_CURVE('',#18149,#18238,#12227,.T.);
#23760=EDGE_CURVE('',#18238,#18239,#12228,.T.);
#23761=EDGE_CURVE('',#18150,#18239,#12229,.T.);
#23762=EDGE_CURVE('',#18151,#17888,#1887,.T.);
#23763=EDGE_CURVE('',#18239,#17889,#12230,.T.);
#23764=EDGE_CURVE('',#17887,#18152,#1888,.T.);
#23765=EDGE_CURVE('',#17886,#18240,#12231,.T.);
#23766=EDGE_CURVE('',#18153,#18240,#12232,.T.);
#23767=EDGE_CURVE('',#18240,#18241,#12233,.T.);
#23768=EDGE_CURVE('',#18154,#18241,#12234,.T.);
#23769=EDGE_CURVE('',#18155,#17884,#1889,.T.);
#23770=EDGE_CURVE('',#18241,#17885,#12235,.T.);
#23771=EDGE_CURVE('',#17883,#18156,#1890,.T.);
#23772=EDGE_CURVE('',#17882,#18242,#12236,.T.);
#23773=EDGE_CURVE('',#18157,#18242,#12237,.T.);
#23774=EDGE_CURVE('',#18242,#18243,#12238,.T.);
#23775=EDGE_CURVE('',#18158,#18243,#12239,.T.);
#23776=EDGE_CURVE('',#18159,#17880,#1891,.T.);
#23777=EDGE_CURVE('',#18243,#17881,#12240,.T.);
#23778=EDGE_CURVE('',#17879,#18160,#1892,.T.);
#23779=EDGE_CURVE('',#17878,#18244,#12241,.T.);
#23780=EDGE_CURVE('',#18161,#18244,#12242,.T.);
#23781=EDGE_CURVE('',#18244,#18245,#12243,.T.);
#23782=EDGE_CURVE('',#18162,#18245,#12244,.T.);
#23783=EDGE_CURVE('',#18163,#17876,#1893,.T.);
#23784=EDGE_CURVE('',#18245,#17877,#12245,.T.);
#23785=EDGE_CURVE('',#17875,#18164,#1894,.T.);
#23786=EDGE_CURVE('',#17874,#18246,#12246,.T.);
#23787=EDGE_CURVE('',#18165,#18246,#12247,.T.);
#23788=EDGE_CURVE('',#18246,#18247,#12248,.T.);
#23789=EDGE_CURVE('',#18166,#18247,#12249,.T.);
#23790=EDGE_CURVE('',#18167,#17872,#1895,.T.);
#23791=EDGE_CURVE('',#18247,#17873,#12250,.T.);
#23792=EDGE_CURVE('',#17871,#18168,#1896,.T.);
#23793=EDGE_CURVE('',#17870,#18248,#12251,.T.);
#23794=EDGE_CURVE('',#18169,#18248,#12252,.T.);
#23795=EDGE_CURVE('',#18248,#18249,#12253,.T.);
#23796=EDGE_CURVE('',#18170,#18249,#12254,.T.);
#23797=EDGE_CURVE('',#18171,#17868,#1897,.T.);
#23798=EDGE_CURVE('',#18249,#17869,#12255,.T.);
#23799=EDGE_CURVE('',#17867,#18172,#1898,.T.);
#23800=EDGE_CURVE('',#17866,#18250,#12256,.T.);
#23801=EDGE_CURVE('',#18173,#18250,#12257,.T.);
#23802=EDGE_CURVE('',#18250,#18251,#12258,.T.);
#23803=EDGE_CURVE('',#18174,#18251,#12259,.T.);
#23804=EDGE_CURVE('',#18175,#17864,#1899,.T.);
#23805=EDGE_CURVE('',#18251,#17865,#12260,.T.);
#23806=EDGE_CURVE('',#17863,#18176,#1900,.T.);
#23807=EDGE_CURVE('',#17862,#18252,#12261,.T.);
#23808=EDGE_CURVE('',#18177,#18252,#12262,.T.);
#23809=EDGE_CURVE('',#18252,#18253,#12263,.T.);
#23810=EDGE_CURVE('',#18178,#18253,#12264,.T.);
#23811=EDGE_CURVE('',#18179,#17860,#1901,.T.);
#23812=EDGE_CURVE('',#18253,#17861,#12265,.T.);
#23813=EDGE_CURVE('',#17859,#18180,#1902,.T.);
#23814=EDGE_CURVE('',#17858,#18254,#12266,.T.);
#23815=EDGE_CURVE('',#18181,#18254,#12267,.T.);
#23816=EDGE_CURVE('',#18254,#18255,#12268,.T.);
#23817=EDGE_CURVE('',#18182,#18255,#12269,.T.);
#23818=EDGE_CURVE('',#18183,#17856,#1903,.T.);
#23819=EDGE_CURVE('',#18255,#17857,#12270,.T.);
#23820=EDGE_CURVE('',#17855,#18184,#1904,.T.);
#23821=EDGE_CURVE('',#17854,#18256,#12271,.T.);
#23822=EDGE_CURVE('',#18185,#18256,#12272,.T.);
#23823=EDGE_CURVE('',#18256,#18257,#12273,.T.);
#23824=EDGE_CURVE('',#18186,#18257,#12274,.T.);
#23825=EDGE_CURVE('',#18187,#17948,#1905,.T.);
#23826=EDGE_CURVE('',#18257,#17949,#12275,.T.);
#23827=EDGE_CURVE('',#17947,#18188,#1906,.T.);
#23828=EDGE_CURVE('',#17946,#18258,#12276,.T.);
#23829=EDGE_CURVE('',#18189,#18258,#12277,.T.);
#23830=EDGE_CURVE('',#18258,#18259,#12278,.T.);
#23831=EDGE_CURVE('',#18190,#18259,#12279,.T.);
#23832=EDGE_CURVE('',#18191,#17944,#1907,.T.);
#23833=EDGE_CURVE('',#18259,#17945,#12280,.T.);
#23834=EDGE_CURVE('',#17943,#18192,#1908,.T.);
#23835=EDGE_CURVE('',#17942,#18260,#12281,.T.);
#23836=EDGE_CURVE('',#18193,#18260,#12282,.T.);
#23837=EDGE_CURVE('',#18260,#18261,#12283,.T.);
#23838=EDGE_CURVE('',#18194,#18261,#12284,.T.);
#23839=EDGE_CURVE('',#18195,#17940,#1909,.T.);
#23840=EDGE_CURVE('',#18261,#17941,#12285,.T.);
#23841=EDGE_CURVE('',#17939,#18196,#1910,.T.);
#23842=EDGE_CURVE('',#17938,#18262,#12286,.T.);
#23843=EDGE_CURVE('',#18197,#18262,#12287,.T.);
#23844=EDGE_CURVE('',#18262,#18263,#12288,.T.);
#23845=EDGE_CURVE('',#18198,#18263,#12289,.T.);
#23846=EDGE_CURVE('',#18199,#17936,#1911,.T.);
#23847=EDGE_CURVE('',#18263,#17937,#12290,.T.);
#23848=EDGE_CURVE('',#17935,#18200,#1912,.T.);
#23849=EDGE_CURVE('',#17934,#18264,#12291,.T.);
#23850=EDGE_CURVE('',#18201,#18264,#12292,.T.);
#23851=EDGE_CURVE('',#18264,#18265,#12293,.T.);
#23852=EDGE_CURVE('',#18202,#18265,#12294,.T.);
#23853=EDGE_CURVE('',#18203,#17932,#1913,.T.);
#23854=EDGE_CURVE('',#18265,#17933,#12295,.T.);
#23855=EDGE_CURVE('',#17931,#18204,#1914,.T.);
#23856=EDGE_CURVE('',#17930,#18266,#12296,.T.);
#23857=EDGE_CURVE('',#18205,#18266,#12297,.T.);
#23858=EDGE_CURVE('',#18266,#18267,#12298,.T.);
#23859=EDGE_CURVE('',#18206,#18267,#12299,.T.);
#23860=EDGE_CURVE('',#18207,#17928,#1915,.T.);
#23861=EDGE_CURVE('',#18267,#17929,#12300,.T.);
#23862=EDGE_CURVE('',#17927,#18208,#1916,.T.);
#23863=EDGE_CURVE('',#17926,#18268,#12301,.T.);
#23864=EDGE_CURVE('',#18209,#18268,#12302,.T.);
#23865=EDGE_CURVE('',#18268,#18269,#12303,.T.);
#23866=EDGE_CURVE('',#18210,#18269,#12304,.T.);
#23867=EDGE_CURVE('',#18211,#17924,#1917,.T.);
#23868=EDGE_CURVE('',#18269,#17925,#12305,.T.);
#23869=EDGE_CURVE('',#17923,#18212,#1918,.T.);
#23870=EDGE_CURVE('',#17922,#18270,#12306,.T.);
#23871=EDGE_CURVE('',#18213,#18270,#12307,.T.);
#23872=EDGE_CURVE('',#18270,#18271,#12308,.T.);
#23873=EDGE_CURVE('',#18214,#18271,#12309,.T.);
#23874=EDGE_CURVE('',#18215,#17920,#1919,.T.);
#23875=EDGE_CURVE('',#18271,#17921,#12310,.T.);
#23876=EDGE_CURVE('',#17919,#18216,#1920,.T.);
#23877=EDGE_CURVE('',#17918,#18272,#12311,.T.);
#23878=EDGE_CURVE('',#18217,#18272,#12312,.T.);
#23879=EDGE_CURVE('',#18272,#18273,#12313,.T.);
#23880=EDGE_CURVE('',#18218,#18273,#12314,.T.);
#23881=EDGE_CURVE('',#18219,#17916,#1921,.T.);
#23882=EDGE_CURVE('',#18273,#17917,#12315,.T.);
#23883=EDGE_CURVE('',#17915,#18220,#1922,.T.);
#23884=EDGE_CURVE('',#17914,#18274,#12316,.T.);
#23885=EDGE_CURVE('',#18221,#18274,#12317,.T.);
#23886=EDGE_CURVE('',#18274,#18275,#12318,.T.);
#23887=EDGE_CURVE('',#18222,#18275,#12319,.T.);
#23888=EDGE_CURVE('',#18223,#17912,#1923,.T.);
#23889=EDGE_CURVE('',#18275,#17913,#12320,.T.);
#23890=EDGE_CURVE('',#17911,#18224,#1924,.T.);
#23891=EDGE_CURVE('',#17910,#18276,#12321,.T.);
#23892=EDGE_CURVE('',#18225,#18276,#12322,.T.);
#23893=EDGE_CURVE('',#18276,#18277,#12323,.T.);
#23894=EDGE_CURVE('',#18226,#18277,#12324,.T.);
#23895=EDGE_CURVE('',#18227,#17908,#1925,.T.);
#23896=EDGE_CURVE('',#18277,#17909,#12325,.T.);
#23897=EDGE_CURVE('',#17907,#18228,#1926,.T.);
#23898=EDGE_CURVE('',#17906,#18278,#12326,.T.);
#23899=EDGE_CURVE('',#18229,#18278,#12327,.T.);
#23900=EDGE_CURVE('',#18278,#18279,#12328,.T.);
#23901=EDGE_CURVE('',#18230,#18279,#12329,.T.);
#23902=EDGE_CURVE('',#18231,#17904,#1927,.T.);
#23903=EDGE_CURVE('',#18279,#17905,#12330,.T.);
#23904=EDGE_CURVE('',#17903,#18232,#1928,.T.);
#23905=EDGE_CURVE('',#17902,#18280,#12331,.T.);
#23906=EDGE_CURVE('',#18233,#18280,#12332,.T.);
#23907=EDGE_CURVE('',#18280,#18281,#12333,.T.);
#23908=EDGE_CURVE('',#18234,#18281,#12334,.T.);
#23909=EDGE_CURVE('',#18281,#17901,#12335,.T.);
#33351=ORIENTED_EDGE('',*,*,#23187,.F.);
#33352=ORIENTED_EDGE('',*,*,#23188,.F.);
#33353=ORIENTED_EDGE('',*,*,#23189,.F.);
#33354=ORIENTED_EDGE('',*,*,#23190,.F.);
#33355=ORIENTED_EDGE('',*,*,#23191,.F.);
#33356=ORIENTED_EDGE('',*,*,#23192,.F.);
#33357=ORIENTED_EDGE('',*,*,#23189,.T.);
#33358=ORIENTED_EDGE('',*,*,#23193,.T.);
#33359=ORIENTED_EDGE('',*,*,#23194,.T.);
#33360=ORIENTED_EDGE('',*,*,#23195,.F.);
#33361=ORIENTED_EDGE('',*,*,#23196,.F.);
#33362=ORIENTED_EDGE('',*,*,#23197,.F.);
#33363=ORIENTED_EDGE('',*,*,#23194,.F.);
#33364=ORIENTED_EDGE('',*,*,#23198,.T.);
#33365=ORIENTED_EDGE('',*,*,#23199,.F.);
#33366=ORIENTED_EDGE('',*,*,#23198,.F.);
#33367=ORIENTED_EDGE('',*,*,#23193,.F.);
#33368=ORIENTED_EDGE('',*,*,#23188,.T.);
#33369=ORIENTED_EDGE('',*,*,#23190,.T.);
#33370=ORIENTED_EDGE('',*,*,#23192,.T.);
#33371=ORIENTED_EDGE('',*,*,#23197,.T.);
#33372=ORIENTED_EDGE('',*,*,#23200,.F.);
#33373=ORIENTED_EDGE('',*,*,#23201,.T.);
#33374=ORIENTED_EDGE('',*,*,#23202,.T.);
#33375=ORIENTED_EDGE('',*,*,#23203,.T.);
#33376=ORIENTED_EDGE('',*,*,#23204,.F.);
#33377=ORIENTED_EDGE('',*,*,#23205,.T.);
#33378=ORIENTED_EDGE('',*,*,#23206,.T.);
#33379=ORIENTED_EDGE('',*,*,#23207,.T.);
#33380=ORIENTED_EDGE('',*,*,#23208,.F.);
#33381=ORIENTED_EDGE('',*,*,#23209,.T.);
#33382=ORIENTED_EDGE('',*,*,#23210,.T.);
#33383=ORIENTED_EDGE('',*,*,#23211,.T.);
#33384=ORIENTED_EDGE('',*,*,#23212,.F.);
#33385=ORIENTED_EDGE('',*,*,#23213,.T.);
#33386=ORIENTED_EDGE('',*,*,#23214,.T.);
#33387=ORIENTED_EDGE('',*,*,#23215,.T.);
#33388=ORIENTED_EDGE('',*,*,#23216,.F.);
#33389=ORIENTED_EDGE('',*,*,#23217,.T.);
#33390=ORIENTED_EDGE('',*,*,#23218,.T.);
#33391=ORIENTED_EDGE('',*,*,#23219,.T.);
#33392=ORIENTED_EDGE('',*,*,#23220,.F.);
#33393=ORIENTED_EDGE('',*,*,#23221,.T.);
#33394=ORIENTED_EDGE('',*,*,#23222,.T.);
#33395=ORIENTED_EDGE('',*,*,#23223,.T.);
#33396=ORIENTED_EDGE('',*,*,#23224,.F.);
#33397=ORIENTED_EDGE('',*,*,#23225,.T.);
#33398=ORIENTED_EDGE('',*,*,#23226,.T.);
#33399=ORIENTED_EDGE('',*,*,#23227,.T.);
#33400=ORIENTED_EDGE('',*,*,#23228,.F.);
#33401=ORIENTED_EDGE('',*,*,#23229,.T.);
#33402=ORIENTED_EDGE('',*,*,#23230,.T.);
#33403=ORIENTED_EDGE('',*,*,#23231,.T.);
#33404=ORIENTED_EDGE('',*,*,#23232,.F.);
#33405=ORIENTED_EDGE('',*,*,#23233,.T.);
#33406=ORIENTED_EDGE('',*,*,#23234,.T.);
#33407=ORIENTED_EDGE('',*,*,#23235,.T.);
#33408=ORIENTED_EDGE('',*,*,#23236,.F.);
#33409=ORIENTED_EDGE('',*,*,#23237,.T.);
#33410=ORIENTED_EDGE('',*,*,#23238,.T.);
#33411=ORIENTED_EDGE('',*,*,#23239,.T.);
#33412=ORIENTED_EDGE('',*,*,#23240,.F.);
#33413=ORIENTED_EDGE('',*,*,#23241,.T.);
#33414=ORIENTED_EDGE('',*,*,#23242,.T.);
#33415=ORIENTED_EDGE('',*,*,#23243,.T.);
#33416=ORIENTED_EDGE('',*,*,#23244,.T.);
#33417=ORIENTED_EDGE('',*,*,#23245,.T.);
#33418=ORIENTED_EDGE('',*,*,#23246,.T.);
#33419=ORIENTED_EDGE('',*,*,#23247,.T.);
#33420=ORIENTED_EDGE('',*,*,#23248,.T.);
#33421=ORIENTED_EDGE('',*,*,#23249,.T.);
#33422=ORIENTED_EDGE('',*,*,#23250,.T.);
#33423=ORIENTED_EDGE('',*,*,#23251,.T.);
#33424=ORIENTED_EDGE('',*,*,#23252,.T.);
#33425=ORIENTED_EDGE('',*,*,#23253,.T.);
#33426=ORIENTED_EDGE('',*,*,#23254,.T.);
#33427=ORIENTED_EDGE('',*,*,#23255,.T.);
#33428=ORIENTED_EDGE('',*,*,#23256,.T.);
#33429=ORIENTED_EDGE('',*,*,#23257,.T.);
#33430=ORIENTED_EDGE('',*,*,#23258,.T.);
#33431=ORIENTED_EDGE('',*,*,#23259,.T.);
#33432=ORIENTED_EDGE('',*,*,#23260,.T.);
#33433=ORIENTED_EDGE('',*,*,#23261,.T.);
#33434=ORIENTED_EDGE('',*,*,#23262,.T.);
#33435=ORIENTED_EDGE('',*,*,#23263,.T.);
#33436=ORIENTED_EDGE('',*,*,#23264,.T.);
#33437=ORIENTED_EDGE('',*,*,#23265,.T.);
#33438=ORIENTED_EDGE('',*,*,#23266,.T.);
#33439=ORIENTED_EDGE('',*,*,#23267,.T.);
#33440=ORIENTED_EDGE('',*,*,#23268,.T.);
#33441=ORIENTED_EDGE('',*,*,#23269,.T.);
#33442=ORIENTED_EDGE('',*,*,#23270,.T.);
#33443=ORIENTED_EDGE('',*,*,#23271,.T.);
#33444=ORIENTED_EDGE('',*,*,#23272,.T.);
#33445=ORIENTED_EDGE('',*,*,#23273,.T.);
#33446=ORIENTED_EDGE('',*,*,#23274,.T.);
#33447=ORIENTED_EDGE('',*,*,#23275,.T.);
#33448=ORIENTED_EDGE('',*,*,#23276,.T.);
#33449=ORIENTED_EDGE('',*,*,#23277,.T.);
#33450=ORIENTED_EDGE('',*,*,#23278,.T.);
#33451=ORIENTED_EDGE('',*,*,#23279,.T.);
#33452=ORIENTED_EDGE('',*,*,#23280,.T.);
#33453=ORIENTED_EDGE('',*,*,#23281,.T.);
#33454=ORIENTED_EDGE('',*,*,#23282,.T.);
#33455=ORIENTED_EDGE('',*,*,#23283,.T.);
#33456=ORIENTED_EDGE('',*,*,#23284,.T.);
#33457=ORIENTED_EDGE('',*,*,#23285,.T.);
#33458=ORIENTED_EDGE('',*,*,#23286,.T.);
#33459=ORIENTED_EDGE('',*,*,#23287,.T.);
#33460=ORIENTED_EDGE('',*,*,#23288,.T.);
#33461=ORIENTED_EDGE('',*,*,#23289,.T.);
#33462=ORIENTED_EDGE('',*,*,#23290,.T.);
#33463=ORIENTED_EDGE('',*,*,#23291,.T.);
#33464=ORIENTED_EDGE('',*,*,#23292,.T.);
#33465=ORIENTED_EDGE('',*,*,#23293,.T.);
#33466=ORIENTED_EDGE('',*,*,#23294,.T.);
#33467=ORIENTED_EDGE('',*,*,#23295,.T.);
#33468=ORIENTED_EDGE('',*,*,#23296,.T.);
#33469=ORIENTED_EDGE('',*,*,#23297,.T.);
#33470=ORIENTED_EDGE('',*,*,#23298,.T.);
#33471=ORIENTED_EDGE('',*,*,#23299,.T.);
#33472=ORIENTED_EDGE('',*,*,#23300,.T.);
#33473=ORIENTED_EDGE('',*,*,#23301,.T.);
#33474=ORIENTED_EDGE('',*,*,#23302,.T.);
#33475=ORIENTED_EDGE('',*,*,#23303,.T.);
#33476=ORIENTED_EDGE('',*,*,#23304,.T.);
#33477=ORIENTED_EDGE('',*,*,#23305,.T.);
#33478=ORIENTED_EDGE('',*,*,#23306,.T.);
#33479=ORIENTED_EDGE('',*,*,#23307,.T.);
#33480=ORIENTED_EDGE('',*,*,#23308,.T.);
#33481=ORIENTED_EDGE('',*,*,#23309,.T.);
#33482=ORIENTED_EDGE('',*,*,#23310,.T.);
#33483=ORIENTED_EDGE('',*,*,#23311,.T.);
#33484=ORIENTED_EDGE('',*,*,#23312,.T.);
#33485=ORIENTED_EDGE('',*,*,#23313,.T.);
#33486=ORIENTED_EDGE('',*,*,#23314,.T.);
#33487=ORIENTED_EDGE('',*,*,#23315,.T.);
#33488=ORIENTED_EDGE('',*,*,#23316,.T.);
#33489=ORIENTED_EDGE('',*,*,#23317,.T.);
#33490=ORIENTED_EDGE('',*,*,#23318,.T.);
#33491=ORIENTED_EDGE('',*,*,#23319,.T.);
#33492=ORIENTED_EDGE('',*,*,#23320,.T.);
#33493=ORIENTED_EDGE('',*,*,#23321,.T.);
#33494=ORIENTED_EDGE('',*,*,#23322,.T.);
#33495=ORIENTED_EDGE('',*,*,#23323,.T.);
#33496=ORIENTED_EDGE('',*,*,#23324,.T.);
#33497=ORIENTED_EDGE('',*,*,#23325,.T.);
#33498=ORIENTED_EDGE('',*,*,#23326,.T.);
#33499=ORIENTED_EDGE('',*,*,#23327,.T.);
#33500=ORIENTED_EDGE('',*,*,#23328,.T.);
#33501=ORIENTED_EDGE('',*,*,#23329,.T.);
#33502=ORIENTED_EDGE('',*,*,#23330,.T.);
#33503=ORIENTED_EDGE('',*,*,#23331,.T.);
#33504=ORIENTED_EDGE('',*,*,#23332,.T.);
#33505=ORIENTED_EDGE('',*,*,#23333,.T.);
#33506=ORIENTED_EDGE('',*,*,#23334,.T.);
#33507=ORIENTED_EDGE('',*,*,#23335,.T.);
#33508=ORIENTED_EDGE('',*,*,#23336,.T.);
#33509=ORIENTED_EDGE('',*,*,#23337,.T.);
#33510=ORIENTED_EDGE('',*,*,#23338,.T.);
#33511=ORIENTED_EDGE('',*,*,#23339,.T.);
#33512=ORIENTED_EDGE('',*,*,#23340,.T.);
#33513=ORIENTED_EDGE('',*,*,#23243,.F.);
#33514=ORIENTED_EDGE('',*,*,#23341,.T.);
#33515=ORIENTED_EDGE('',*,*,#23342,.T.);
#33516=ORIENTED_EDGE('',*,*,#23343,.F.);
#33517=ORIENTED_EDGE('',*,*,#23344,.T.);
#33518=ORIENTED_EDGE('',*,*,#23345,.T.);
#33519=ORIENTED_EDGE('',*,*,#23346,.T.);
#33520=ORIENTED_EDGE('',*,*,#23347,.F.);
#33521=ORIENTED_EDGE('',*,*,#23348,.T.);
#33522=ORIENTED_EDGE('',*,*,#23349,.T.);
#33523=ORIENTED_EDGE('',*,*,#23350,.T.);
#33524=ORIENTED_EDGE('',*,*,#23351,.F.);
#33525=ORIENTED_EDGE('',*,*,#23352,.T.);
#33526=ORIENTED_EDGE('',*,*,#23353,.T.);
#33527=ORIENTED_EDGE('',*,*,#23354,.T.);
#33528=ORIENTED_EDGE('',*,*,#23355,.F.);
#33529=ORIENTED_EDGE('',*,*,#23356,.T.);
#33530=ORIENTED_EDGE('',*,*,#23357,.T.);
#33531=ORIENTED_EDGE('',*,*,#23358,.T.);
#33532=ORIENTED_EDGE('',*,*,#23359,.F.);
#33533=ORIENTED_EDGE('',*,*,#23360,.T.);
#33534=ORIENTED_EDGE('',*,*,#23361,.T.);
#33535=ORIENTED_EDGE('',*,*,#23362,.T.);
#33536=ORIENTED_EDGE('',*,*,#23363,.F.);
#33537=ORIENTED_EDGE('',*,*,#23364,.T.);
#33538=ORIENTED_EDGE('',*,*,#23365,.T.);
#33539=ORIENTED_EDGE('',*,*,#23366,.T.);
#33540=ORIENTED_EDGE('',*,*,#23367,.F.);
#33541=ORIENTED_EDGE('',*,*,#23368,.T.);
#33542=ORIENTED_EDGE('',*,*,#23369,.T.);
#33543=ORIENTED_EDGE('',*,*,#23370,.T.);
#33544=ORIENTED_EDGE('',*,*,#23371,.F.);
#33545=ORIENTED_EDGE('',*,*,#23372,.T.);
#33546=ORIENTED_EDGE('',*,*,#23373,.T.);
#33547=ORIENTED_EDGE('',*,*,#23374,.T.);
#33548=ORIENTED_EDGE('',*,*,#23375,.F.);
#33549=ORIENTED_EDGE('',*,*,#23376,.T.);
#33550=ORIENTED_EDGE('',*,*,#23377,.T.);
#33551=ORIENTED_EDGE('',*,*,#23378,.T.);
#33552=ORIENTED_EDGE('',*,*,#23379,.F.);
#33553=ORIENTED_EDGE('',*,*,#23380,.T.);
#33554=ORIENTED_EDGE('',*,*,#23381,.T.);
#33555=ORIENTED_EDGE('',*,*,#23382,.T.);
#33556=ORIENTED_EDGE('',*,*,#23383,.F.);
#33557=ORIENTED_EDGE('',*,*,#23384,.T.);
#33558=ORIENTED_EDGE('',*,*,#23385,.T.);
#33559=ORIENTED_EDGE('',*,*,#23386,.T.);
#33560=ORIENTED_EDGE('',*,*,#23387,.F.);
#33561=ORIENTED_EDGE('',*,*,#23388,.T.);
#33562=ORIENTED_EDGE('',*,*,#23389,.T.);
#33563=ORIENTED_EDGE('',*,*,#23390,.T.);
#33564=ORIENTED_EDGE('',*,*,#23391,.F.);
#33565=ORIENTED_EDGE('',*,*,#23196,.T.);
#33566=ORIENTED_EDGE('',*,*,#23392,.F.);
#33567=ORIENTED_EDGE('',*,*,#23393,.T.);
#33568=ORIENTED_EDGE('',*,*,#23200,.T.);
#33569=ORIENTED_EDGE('',*,*,#23191,.T.);
#33570=ORIENTED_EDGE('',*,*,#23391,.T.);
#33571=ORIENTED_EDGE('',*,*,#23394,.T.);
#33572=ORIENTED_EDGE('',*,*,#23395,.F.);
#33573=ORIENTED_EDGE('',*,*,#23396,.F.);
#33574=ORIENTED_EDGE('',*,*,#23397,.F.);
#33575=ORIENTED_EDGE('',*,*,#23398,.F.);
#33576=ORIENTED_EDGE('',*,*,#23201,.F.);
#33577=ORIENTED_EDGE('',*,*,#23393,.F.);
#33578=ORIENTED_EDGE('',*,*,#23202,.F.);
#33579=ORIENTED_EDGE('',*,*,#23398,.T.);
#33580=ORIENTED_EDGE('',*,*,#23399,.T.);
#33581=ORIENTED_EDGE('',*,*,#23400,.T.);
#33582=ORIENTED_EDGE('',*,*,#23401,.F.);
#33583=ORIENTED_EDGE('',*,*,#23402,.F.);
#33584=ORIENTED_EDGE('',*,*,#23203,.F.);
#33585=ORIENTED_EDGE('',*,*,#23400,.F.);
#33586=ORIENTED_EDGE('',*,*,#23403,.T.);
#33587=ORIENTED_EDGE('',*,*,#23404,.F.);
#33588=ORIENTED_EDGE('',*,*,#23403,.F.);
#33589=ORIENTED_EDGE('',*,*,#23399,.F.);
#33590=ORIENTED_EDGE('',*,*,#23397,.T.);
#33591=ORIENTED_EDGE('',*,*,#23402,.T.);
#33592=ORIENTED_EDGE('',*,*,#23405,.F.);
#33593=ORIENTED_EDGE('',*,*,#23406,.T.);
#33594=ORIENTED_EDGE('',*,*,#23204,.T.);
#33595=ORIENTED_EDGE('',*,*,#23407,.F.);
#33596=ORIENTED_EDGE('',*,*,#23408,.F.);
#33597=ORIENTED_EDGE('',*,*,#23409,.F.);
#33598=ORIENTED_EDGE('',*,*,#23205,.F.);
#33599=ORIENTED_EDGE('',*,*,#23406,.F.);
#33600=ORIENTED_EDGE('',*,*,#23206,.F.);
#33601=ORIENTED_EDGE('',*,*,#23409,.T.);
#33602=ORIENTED_EDGE('',*,*,#23410,.T.);
#33603=ORIENTED_EDGE('',*,*,#23411,.T.);
#33604=ORIENTED_EDGE('',*,*,#23412,.F.);
#33605=ORIENTED_EDGE('',*,*,#23413,.F.);
#33606=ORIENTED_EDGE('',*,*,#23207,.F.);
#33607=ORIENTED_EDGE('',*,*,#23411,.F.);
#33608=ORIENTED_EDGE('',*,*,#23414,.T.);
#33609=ORIENTED_EDGE('',*,*,#23415,.F.);
#33610=ORIENTED_EDGE('',*,*,#23414,.F.);
#33611=ORIENTED_EDGE('',*,*,#23410,.F.);
#33612=ORIENTED_EDGE('',*,*,#23408,.T.);
#33613=ORIENTED_EDGE('',*,*,#23413,.T.);
#33614=ORIENTED_EDGE('',*,*,#23416,.F.);
#33615=ORIENTED_EDGE('',*,*,#23417,.T.);
#33616=ORIENTED_EDGE('',*,*,#23208,.T.);
#33617=ORIENTED_EDGE('',*,*,#23418,.F.);
#33618=ORIENTED_EDGE('',*,*,#23419,.F.);
#33619=ORIENTED_EDGE('',*,*,#23420,.F.);
#33620=ORIENTED_EDGE('',*,*,#23209,.F.);
#33621=ORIENTED_EDGE('',*,*,#23417,.F.);
#33622=ORIENTED_EDGE('',*,*,#23210,.F.);
#33623=ORIENTED_EDGE('',*,*,#23420,.T.);
#33624=ORIENTED_EDGE('',*,*,#23421,.T.);
#33625=ORIENTED_EDGE('',*,*,#23422,.T.);
#33626=ORIENTED_EDGE('',*,*,#23423,.F.);
#33627=ORIENTED_EDGE('',*,*,#23424,.F.);
#33628=ORIENTED_EDGE('',*,*,#23211,.F.);
#33629=ORIENTED_EDGE('',*,*,#23422,.F.);
#33630=ORIENTED_EDGE('',*,*,#23425,.T.);
#33631=ORIENTED_EDGE('',*,*,#23426,.F.);
#33632=ORIENTED_EDGE('',*,*,#23425,.F.);
#33633=ORIENTED_EDGE('',*,*,#23421,.F.);
#33634=ORIENTED_EDGE('',*,*,#23419,.T.);
#33635=ORIENTED_EDGE('',*,*,#23424,.T.);
#33636=ORIENTED_EDGE('',*,*,#23427,.F.);
#33637=ORIENTED_EDGE('',*,*,#23428,.T.);
#33638=ORIENTED_EDGE('',*,*,#23212,.T.);
#33639=ORIENTED_EDGE('',*,*,#23429,.F.);
#33640=ORIENTED_EDGE('',*,*,#23430,.F.);
#33641=ORIENTED_EDGE('',*,*,#23431,.F.);
#33642=ORIENTED_EDGE('',*,*,#23213,.F.);
#33643=ORIENTED_EDGE('',*,*,#23428,.F.);
#33644=ORIENTED_EDGE('',*,*,#23214,.F.);
#33645=ORIENTED_EDGE('',*,*,#23431,.T.);
#33646=ORIENTED_EDGE('',*,*,#23432,.T.);
#33647=ORIENTED_EDGE('',*,*,#23433,.T.);
#33648=ORIENTED_EDGE('',*,*,#23434,.F.);
#33649=ORIENTED_EDGE('',*,*,#23435,.F.);
#33650=ORIENTED_EDGE('',*,*,#23215,.F.);
#33651=ORIENTED_EDGE('',*,*,#23433,.F.);
#33652=ORIENTED_EDGE('',*,*,#23436,.T.);
#33653=ORIENTED_EDGE('',*,*,#23437,.F.);
#33654=ORIENTED_EDGE('',*,*,#23436,.F.);
#33655=ORIENTED_EDGE('',*,*,#23432,.F.);
#33656=ORIENTED_EDGE('',*,*,#23430,.T.);
#33657=ORIENTED_EDGE('',*,*,#23435,.T.);
#33658=ORIENTED_EDGE('',*,*,#23438,.F.);
#33659=ORIENTED_EDGE('',*,*,#23439,.T.);
#33660=ORIENTED_EDGE('',*,*,#23216,.T.);
#33661=ORIENTED_EDGE('',*,*,#23440,.F.);
#33662=ORIENTED_EDGE('',*,*,#23441,.F.);
#33663=ORIENTED_EDGE('',*,*,#23442,.F.);
#33664=ORIENTED_EDGE('',*,*,#23217,.F.);
#33665=ORIENTED_EDGE('',*,*,#23439,.F.);
#33666=ORIENTED_EDGE('',*,*,#23218,.F.);
#33667=ORIENTED_EDGE('',*,*,#23442,.T.);
#33668=ORIENTED_EDGE('',*,*,#23443,.T.);
#33669=ORIENTED_EDGE('',*,*,#23444,.T.);
#33670=ORIENTED_EDGE('',*,*,#23445,.F.);
#33671=ORIENTED_EDGE('',*,*,#23446,.F.);
#33672=ORIENTED_EDGE('',*,*,#23219,.F.);
#33673=ORIENTED_EDGE('',*,*,#23444,.F.);
#33674=ORIENTED_EDGE('',*,*,#23447,.T.);
#33675=ORIENTED_EDGE('',*,*,#23448,.F.);
#33676=ORIENTED_EDGE('',*,*,#23447,.F.);
#33677=ORIENTED_EDGE('',*,*,#23443,.F.);
#33678=ORIENTED_EDGE('',*,*,#23441,.T.);
#33679=ORIENTED_EDGE('',*,*,#23446,.T.);
#33680=ORIENTED_EDGE('',*,*,#23449,.F.);
#33681=ORIENTED_EDGE('',*,*,#23450,.T.);
#33682=ORIENTED_EDGE('',*,*,#23220,.T.);
#33683=ORIENTED_EDGE('',*,*,#23451,.F.);
#33684=ORIENTED_EDGE('',*,*,#23452,.F.);
#33685=ORIENTED_EDGE('',*,*,#23453,.F.);
#33686=ORIENTED_EDGE('',*,*,#23221,.F.);
#33687=ORIENTED_EDGE('',*,*,#23450,.F.);
#33688=ORIENTED_EDGE('',*,*,#23222,.F.);
#33689=ORIENTED_EDGE('',*,*,#23453,.T.);
#33690=ORIENTED_EDGE('',*,*,#23454,.T.);
#33691=ORIENTED_EDGE('',*,*,#23455,.T.);
#33692=ORIENTED_EDGE('',*,*,#23456,.F.);
#33693=ORIENTED_EDGE('',*,*,#23457,.F.);
#33694=ORIENTED_EDGE('',*,*,#23223,.F.);
#33695=ORIENTED_EDGE('',*,*,#23455,.F.);
#33696=ORIENTED_EDGE('',*,*,#23458,.T.);
#33697=ORIENTED_EDGE('',*,*,#23459,.F.);
#33698=ORIENTED_EDGE('',*,*,#23458,.F.);
#33699=ORIENTED_EDGE('',*,*,#23454,.F.);
#33700=ORIENTED_EDGE('',*,*,#23452,.T.);
#33701=ORIENTED_EDGE('',*,*,#23457,.T.);
#33702=ORIENTED_EDGE('',*,*,#23460,.F.);
#33703=ORIENTED_EDGE('',*,*,#23461,.T.);
#33704=ORIENTED_EDGE('',*,*,#23224,.T.);
#33705=ORIENTED_EDGE('',*,*,#23462,.F.);
#33706=ORIENTED_EDGE('',*,*,#23463,.F.);
#33707=ORIENTED_EDGE('',*,*,#23464,.F.);
#33708=ORIENTED_EDGE('',*,*,#23225,.F.);
#33709=ORIENTED_EDGE('',*,*,#23461,.F.);
#33710=ORIENTED_EDGE('',*,*,#23226,.F.);
#33711=ORIENTED_EDGE('',*,*,#23464,.T.);
#33712=ORIENTED_EDGE('',*,*,#23465,.T.);
#33713=ORIENTED_EDGE('',*,*,#23466,.T.);
#33714=ORIENTED_EDGE('',*,*,#23467,.F.);
#33715=ORIENTED_EDGE('',*,*,#23468,.F.);
#33716=ORIENTED_EDGE('',*,*,#23227,.F.);
#33717=ORIENTED_EDGE('',*,*,#23466,.F.);
#33718=ORIENTED_EDGE('',*,*,#23469,.T.);
#33719=ORIENTED_EDGE('',*,*,#23470,.F.);
#33720=ORIENTED_EDGE('',*,*,#23469,.F.);
#33721=ORIENTED_EDGE('',*,*,#23465,.F.);
#33722=ORIENTED_EDGE('',*,*,#23463,.T.);
#33723=ORIENTED_EDGE('',*,*,#23468,.T.);
#33724=ORIENTED_EDGE('',*,*,#23471,.F.);
#33725=ORIENTED_EDGE('',*,*,#23472,.T.);
#33726=ORIENTED_EDGE('',*,*,#23228,.T.);
#33727=ORIENTED_EDGE('',*,*,#23473,.F.);
#33728=ORIENTED_EDGE('',*,*,#23474,.F.);
#33729=ORIENTED_EDGE('',*,*,#23475,.F.);
#33730=ORIENTED_EDGE('',*,*,#23229,.F.);
#33731=ORIENTED_EDGE('',*,*,#23472,.F.);
#33732=ORIENTED_EDGE('',*,*,#23230,.F.);
#33733=ORIENTED_EDGE('',*,*,#23475,.T.);
#33734=ORIENTED_EDGE('',*,*,#23476,.T.);
#33735=ORIENTED_EDGE('',*,*,#23477,.T.);
#33736=ORIENTED_EDGE('',*,*,#23478,.F.);
#33737=ORIENTED_EDGE('',*,*,#23479,.F.);
#33738=ORIENTED_EDGE('',*,*,#23231,.F.);
#33739=ORIENTED_EDGE('',*,*,#23477,.F.);
#33740=ORIENTED_EDGE('',*,*,#23480,.T.);
#33741=ORIENTED_EDGE('',*,*,#23481,.F.);
#33742=ORIENTED_EDGE('',*,*,#23480,.F.);
#33743=ORIENTED_EDGE('',*,*,#23476,.F.);
#33744=ORIENTED_EDGE('',*,*,#23474,.T.);
#33745=ORIENTED_EDGE('',*,*,#23479,.T.);
#33746=ORIENTED_EDGE('',*,*,#23482,.F.);
#33747=ORIENTED_EDGE('',*,*,#23483,.T.);
#33748=ORIENTED_EDGE('',*,*,#23232,.T.);
#33749=ORIENTED_EDGE('',*,*,#23484,.F.);
#33750=ORIENTED_EDGE('',*,*,#23485,.F.);
#33751=ORIENTED_EDGE('',*,*,#23486,.F.);
#33752=ORIENTED_EDGE('',*,*,#23233,.F.);
#33753=ORIENTED_EDGE('',*,*,#23483,.F.);
#33754=ORIENTED_EDGE('',*,*,#23234,.F.);
#33755=ORIENTED_EDGE('',*,*,#23486,.T.);
#33756=ORIENTED_EDGE('',*,*,#23487,.T.);
#33757=ORIENTED_EDGE('',*,*,#23488,.T.);
#33758=ORIENTED_EDGE('',*,*,#23489,.F.);
#33759=ORIENTED_EDGE('',*,*,#23490,.F.);
#33760=ORIENTED_EDGE('',*,*,#23235,.F.);
#33761=ORIENTED_EDGE('',*,*,#23488,.F.);
#33762=ORIENTED_EDGE('',*,*,#23491,.T.);
#33763=ORIENTED_EDGE('',*,*,#23492,.F.);
#33764=ORIENTED_EDGE('',*,*,#23491,.F.);
#33765=ORIENTED_EDGE('',*,*,#23487,.F.);
#33766=ORIENTED_EDGE('',*,*,#23485,.T.);
#33767=ORIENTED_EDGE('',*,*,#23490,.T.);
#33768=ORIENTED_EDGE('',*,*,#23493,.F.);
#33769=ORIENTED_EDGE('',*,*,#23494,.T.);
#33770=ORIENTED_EDGE('',*,*,#23236,.T.);
#33771=ORIENTED_EDGE('',*,*,#23495,.F.);
#33772=ORIENTED_EDGE('',*,*,#23496,.F.);
#33773=ORIENTED_EDGE('',*,*,#23497,.F.);
#33774=ORIENTED_EDGE('',*,*,#23237,.F.);
#33775=ORIENTED_EDGE('',*,*,#23494,.F.);
#33776=ORIENTED_EDGE('',*,*,#23238,.F.);
#33777=ORIENTED_EDGE('',*,*,#23497,.T.);
#33778=ORIENTED_EDGE('',*,*,#23498,.T.);
#33779=ORIENTED_EDGE('',*,*,#23499,.T.);
#33780=ORIENTED_EDGE('',*,*,#23500,.F.);
#33781=ORIENTED_EDGE('',*,*,#23501,.F.);
#33782=ORIENTED_EDGE('',*,*,#23239,.F.);
#33783=ORIENTED_EDGE('',*,*,#23499,.F.);
#33784=ORIENTED_EDGE('',*,*,#23502,.T.);
#33785=ORIENTED_EDGE('',*,*,#23503,.F.);
#33786=ORIENTED_EDGE('',*,*,#23502,.F.);
#33787=ORIENTED_EDGE('',*,*,#23498,.F.);
#33788=ORIENTED_EDGE('',*,*,#23496,.T.);
#33789=ORIENTED_EDGE('',*,*,#23501,.T.);
#33790=ORIENTED_EDGE('',*,*,#23504,.F.);
#33791=ORIENTED_EDGE('',*,*,#23505,.T.);
#33792=ORIENTED_EDGE('',*,*,#23240,.T.);
#33793=ORIENTED_EDGE('',*,*,#23506,.F.);
#33794=ORIENTED_EDGE('',*,*,#23507,.F.);
#33795=ORIENTED_EDGE('',*,*,#23508,.F.);
#33796=ORIENTED_EDGE('',*,*,#23241,.F.);
#33797=ORIENTED_EDGE('',*,*,#23505,.F.);
#33798=ORIENTED_EDGE('',*,*,#23242,.F.);
#33799=ORIENTED_EDGE('',*,*,#23508,.T.);
#33800=ORIENTED_EDGE('',*,*,#23509,.T.);
#33801=ORIENTED_EDGE('',*,*,#23510,.T.);
#33802=ORIENTED_EDGE('',*,*,#23341,.F.);
#33803=ORIENTED_EDGE('',*,*,#23511,.F.);
#33804=ORIENTED_EDGE('',*,*,#23512,.F.);
#33805=ORIENTED_EDGE('',*,*,#23342,.F.);
#33806=ORIENTED_EDGE('',*,*,#23510,.F.);
#33807=ORIENTED_EDGE('',*,*,#23513,.T.);
#33808=ORIENTED_EDGE('',*,*,#23514,.F.);
#33809=ORIENTED_EDGE('',*,*,#23513,.F.);
#33810=ORIENTED_EDGE('',*,*,#23509,.F.);
#33811=ORIENTED_EDGE('',*,*,#23507,.T.);
#33812=ORIENTED_EDGE('',*,*,#23512,.T.);
#33813=ORIENTED_EDGE('',*,*,#23515,.F.);
#33814=ORIENTED_EDGE('',*,*,#23516,.T.);
#33815=ORIENTED_EDGE('',*,*,#23343,.T.);
#33816=ORIENTED_EDGE('',*,*,#23517,.F.);
#33817=ORIENTED_EDGE('',*,*,#23518,.F.);
#33818=ORIENTED_EDGE('',*,*,#23519,.F.);
#33819=ORIENTED_EDGE('',*,*,#23344,.F.);
#33820=ORIENTED_EDGE('',*,*,#23516,.F.);
#33821=ORIENTED_EDGE('',*,*,#23345,.F.);
#33822=ORIENTED_EDGE('',*,*,#23519,.T.);
#33823=ORIENTED_EDGE('',*,*,#23520,.T.);
#33824=ORIENTED_EDGE('',*,*,#23521,.T.);
#33825=ORIENTED_EDGE('',*,*,#23522,.F.);
#33826=ORIENTED_EDGE('',*,*,#23523,.F.);
#33827=ORIENTED_EDGE('',*,*,#23346,.F.);
#33828=ORIENTED_EDGE('',*,*,#23521,.F.);
#33829=ORIENTED_EDGE('',*,*,#23524,.T.);
#33830=ORIENTED_EDGE('',*,*,#23525,.F.);
#33831=ORIENTED_EDGE('',*,*,#23524,.F.);
#33832=ORIENTED_EDGE('',*,*,#23520,.F.);
#33833=ORIENTED_EDGE('',*,*,#23518,.T.);
#33834=ORIENTED_EDGE('',*,*,#23523,.T.);
#33835=ORIENTED_EDGE('',*,*,#23526,.F.);
#33836=ORIENTED_EDGE('',*,*,#23527,.T.);
#33837=ORIENTED_EDGE('',*,*,#23347,.T.);
#33838=ORIENTED_EDGE('',*,*,#23528,.F.);
#33839=ORIENTED_EDGE('',*,*,#23529,.F.);
#33840=ORIENTED_EDGE('',*,*,#23530,.F.);
#33841=ORIENTED_EDGE('',*,*,#23348,.F.);
#33842=ORIENTED_EDGE('',*,*,#23527,.F.);
#33843=ORIENTED_EDGE('',*,*,#23349,.F.);
#33844=ORIENTED_EDGE('',*,*,#23530,.T.);
#33845=ORIENTED_EDGE('',*,*,#23531,.T.);
#33846=ORIENTED_EDGE('',*,*,#23532,.T.);
#33847=ORIENTED_EDGE('',*,*,#23533,.F.);
#33848=ORIENTED_EDGE('',*,*,#23534,.F.);
#33849=ORIENTED_EDGE('',*,*,#23350,.F.);
#33850=ORIENTED_EDGE('',*,*,#23532,.F.);
#33851=ORIENTED_EDGE('',*,*,#23535,.T.);
#33852=ORIENTED_EDGE('',*,*,#23536,.F.);
#33853=ORIENTED_EDGE('',*,*,#23535,.F.);
#33854=ORIENTED_EDGE('',*,*,#23531,.F.);
#33855=ORIENTED_EDGE('',*,*,#23529,.T.);
#33856=ORIENTED_EDGE('',*,*,#23534,.T.);
#33857=ORIENTED_EDGE('',*,*,#23537,.F.);
#33858=ORIENTED_EDGE('',*,*,#23538,.T.);
#33859=ORIENTED_EDGE('',*,*,#23351,.T.);
#33860=ORIENTED_EDGE('',*,*,#23539,.F.);
#33861=ORIENTED_EDGE('',*,*,#23540,.F.);
#33862=ORIENTED_EDGE('',*,*,#23541,.F.);
#33863=ORIENTED_EDGE('',*,*,#23352,.F.);
#33864=ORIENTED_EDGE('',*,*,#23538,.F.);
#33865=ORIENTED_EDGE('',*,*,#23353,.F.);
#33866=ORIENTED_EDGE('',*,*,#23541,.T.);
#33867=ORIENTED_EDGE('',*,*,#23542,.T.);
#33868=ORIENTED_EDGE('',*,*,#23543,.T.);
#33869=ORIENTED_EDGE('',*,*,#23544,.F.);
#33870=ORIENTED_EDGE('',*,*,#23545,.F.);
#33871=ORIENTED_EDGE('',*,*,#23354,.F.);
#33872=ORIENTED_EDGE('',*,*,#23543,.F.);
#33873=ORIENTED_EDGE('',*,*,#23546,.T.);
#33874=ORIENTED_EDGE('',*,*,#23547,.F.);
#33875=ORIENTED_EDGE('',*,*,#23546,.F.);
#33876=ORIENTED_EDGE('',*,*,#23542,.F.);
#33877=ORIENTED_EDGE('',*,*,#23540,.T.);
#33878=ORIENTED_EDGE('',*,*,#23545,.T.);
#33879=ORIENTED_EDGE('',*,*,#23548,.F.);
#33880=ORIENTED_EDGE('',*,*,#23549,.T.);
#33881=ORIENTED_EDGE('',*,*,#23355,.T.);
#33882=ORIENTED_EDGE('',*,*,#23550,.F.);
#33883=ORIENTED_EDGE('',*,*,#23551,.F.);
#33884=ORIENTED_EDGE('',*,*,#23552,.F.);
#33885=ORIENTED_EDGE('',*,*,#23356,.F.);
#33886=ORIENTED_EDGE('',*,*,#23549,.F.);
#33887=ORIENTED_EDGE('',*,*,#23357,.F.);
#33888=ORIENTED_EDGE('',*,*,#23552,.T.);
#33889=ORIENTED_EDGE('',*,*,#23553,.T.);
#33890=ORIENTED_EDGE('',*,*,#23554,.T.);
#33891=ORIENTED_EDGE('',*,*,#23555,.F.);
#33892=ORIENTED_EDGE('',*,*,#23556,.F.);
#33893=ORIENTED_EDGE('',*,*,#23358,.F.);
#33894=ORIENTED_EDGE('',*,*,#23554,.F.);
#33895=ORIENTED_EDGE('',*,*,#23557,.T.);
#33896=ORIENTED_EDGE('',*,*,#23558,.F.);
#33897=ORIENTED_EDGE('',*,*,#23557,.F.);
#33898=ORIENTED_EDGE('',*,*,#23553,.F.);
#33899=ORIENTED_EDGE('',*,*,#23551,.T.);
#33900=ORIENTED_EDGE('',*,*,#23556,.T.);
#33901=ORIENTED_EDGE('',*,*,#23559,.F.);
#33902=ORIENTED_EDGE('',*,*,#23560,.T.);
#33903=ORIENTED_EDGE('',*,*,#23359,.T.);
#33904=ORIENTED_EDGE('',*,*,#23561,.F.);
#33905=ORIENTED_EDGE('',*,*,#23562,.F.);
#33906=ORIENTED_EDGE('',*,*,#23563,.F.);
#33907=ORIENTED_EDGE('',*,*,#23360,.F.);
#33908=ORIENTED_EDGE('',*,*,#23560,.F.);
#33909=ORIENTED_EDGE('',*,*,#23361,.F.);
#33910=ORIENTED_EDGE('',*,*,#23563,.T.);
#33911=ORIENTED_EDGE('',*,*,#23564,.T.);
#33912=ORIENTED_EDGE('',*,*,#23565,.T.);
#33913=ORIENTED_EDGE('',*,*,#23566,.F.);
#33914=ORIENTED_EDGE('',*,*,#23567,.F.);
#33915=ORIENTED_EDGE('',*,*,#23362,.F.);
#33916=ORIENTED_EDGE('',*,*,#23565,.F.);
#33917=ORIENTED_EDGE('',*,*,#23568,.T.);
#33918=ORIENTED_EDGE('',*,*,#23569,.F.);
#33919=ORIENTED_EDGE('',*,*,#23568,.F.);
#33920=ORIENTED_EDGE('',*,*,#23564,.F.);
#33921=ORIENTED_EDGE('',*,*,#23562,.T.);
#33922=ORIENTED_EDGE('',*,*,#23567,.T.);
#33923=ORIENTED_EDGE('',*,*,#23570,.F.);
#33924=ORIENTED_EDGE('',*,*,#23571,.T.);
#33925=ORIENTED_EDGE('',*,*,#23363,.T.);
#33926=ORIENTED_EDGE('',*,*,#23572,.F.);
#33927=ORIENTED_EDGE('',*,*,#23573,.F.);
#33928=ORIENTED_EDGE('',*,*,#23574,.F.);
#33929=ORIENTED_EDGE('',*,*,#23364,.F.);
#33930=ORIENTED_EDGE('',*,*,#23571,.F.);
#33931=ORIENTED_EDGE('',*,*,#23365,.F.);
#33932=ORIENTED_EDGE('',*,*,#23574,.T.);
#33933=ORIENTED_EDGE('',*,*,#23575,.T.);
#33934=ORIENTED_EDGE('',*,*,#23576,.T.);
#33935=ORIENTED_EDGE('',*,*,#23577,.F.);
#33936=ORIENTED_EDGE('',*,*,#23578,.F.);
#33937=ORIENTED_EDGE('',*,*,#23366,.F.);
#33938=ORIENTED_EDGE('',*,*,#23576,.F.);
#33939=ORIENTED_EDGE('',*,*,#23579,.T.);
#33940=ORIENTED_EDGE('',*,*,#23580,.F.);
#33941=ORIENTED_EDGE('',*,*,#23579,.F.);
#33942=ORIENTED_EDGE('',*,*,#23575,.F.);
#33943=ORIENTED_EDGE('',*,*,#23573,.T.);
#33944=ORIENTED_EDGE('',*,*,#23578,.T.);
#33945=ORIENTED_EDGE('',*,*,#23581,.F.);
#33946=ORIENTED_EDGE('',*,*,#23582,.T.);
#33947=ORIENTED_EDGE('',*,*,#23367,.T.);
#33948=ORIENTED_EDGE('',*,*,#23583,.F.);
#33949=ORIENTED_EDGE('',*,*,#23584,.F.);
#33950=ORIENTED_EDGE('',*,*,#23585,.F.);
#33951=ORIENTED_EDGE('',*,*,#23368,.F.);
#33952=ORIENTED_EDGE('',*,*,#23582,.F.);
#33953=ORIENTED_EDGE('',*,*,#23369,.F.);
#33954=ORIENTED_EDGE('',*,*,#23585,.T.);
#33955=ORIENTED_EDGE('',*,*,#23586,.T.);
#33956=ORIENTED_EDGE('',*,*,#23587,.T.);
#33957=ORIENTED_EDGE('',*,*,#23588,.F.);
#33958=ORIENTED_EDGE('',*,*,#23589,.F.);
#33959=ORIENTED_EDGE('',*,*,#23370,.F.);
#33960=ORIENTED_EDGE('',*,*,#23587,.F.);
#33961=ORIENTED_EDGE('',*,*,#23590,.T.);
#33962=ORIENTED_EDGE('',*,*,#23591,.F.);
#33963=ORIENTED_EDGE('',*,*,#23590,.F.);
#33964=ORIENTED_EDGE('',*,*,#23586,.F.);
#33965=ORIENTED_EDGE('',*,*,#23584,.T.);
#33966=ORIENTED_EDGE('',*,*,#23589,.T.);
#33967=ORIENTED_EDGE('',*,*,#23592,.F.);
#33968=ORIENTED_EDGE('',*,*,#23593,.T.);
#33969=ORIENTED_EDGE('',*,*,#23371,.T.);
#33970=ORIENTED_EDGE('',*,*,#23594,.F.);
#33971=ORIENTED_EDGE('',*,*,#23595,.F.);
#33972=ORIENTED_EDGE('',*,*,#23596,.F.);
#33973=ORIENTED_EDGE('',*,*,#23372,.F.);
#33974=ORIENTED_EDGE('',*,*,#23593,.F.);
#33975=ORIENTED_EDGE('',*,*,#23373,.F.);
#33976=ORIENTED_EDGE('',*,*,#23596,.T.);
#33977=ORIENTED_EDGE('',*,*,#23597,.T.);
#33978=ORIENTED_EDGE('',*,*,#23598,.T.);
#33979=ORIENTED_EDGE('',*,*,#23599,.F.);
#33980=ORIENTED_EDGE('',*,*,#23600,.F.);
#33981=ORIENTED_EDGE('',*,*,#23374,.F.);
#33982=ORIENTED_EDGE('',*,*,#23598,.F.);
#33983=ORIENTED_EDGE('',*,*,#23601,.T.);
#33984=ORIENTED_EDGE('',*,*,#23602,.F.);
#33985=ORIENTED_EDGE('',*,*,#23601,.F.);
#33986=ORIENTED_EDGE('',*,*,#23597,.F.);
#33987=ORIENTED_EDGE('',*,*,#23595,.T.);
#33988=ORIENTED_EDGE('',*,*,#23600,.T.);
#33989=ORIENTED_EDGE('',*,*,#23603,.F.);
#33990=ORIENTED_EDGE('',*,*,#23604,.T.);
#33991=ORIENTED_EDGE('',*,*,#23375,.T.);
#33992=ORIENTED_EDGE('',*,*,#23605,.F.);
#33993=ORIENTED_EDGE('',*,*,#23606,.F.);
#33994=ORIENTED_EDGE('',*,*,#23607,.F.);
#33995=ORIENTED_EDGE('',*,*,#23376,.F.);
#33996=ORIENTED_EDGE('',*,*,#23604,.F.);
#33997=ORIENTED_EDGE('',*,*,#23377,.F.);
#33998=ORIENTED_EDGE('',*,*,#23607,.T.);
#33999=ORIENTED_EDGE('',*,*,#23608,.T.);
#34000=ORIENTED_EDGE('',*,*,#23609,.T.);
#34001=ORIENTED_EDGE('',*,*,#23610,.F.);
#34002=ORIENTED_EDGE('',*,*,#23611,.F.);
#34003=ORIENTED_EDGE('',*,*,#23378,.F.);
#34004=ORIENTED_EDGE('',*,*,#23609,.F.);
#34005=ORIENTED_EDGE('',*,*,#23612,.T.);
#34006=ORIENTED_EDGE('',*,*,#23613,.F.);
#34007=ORIENTED_EDGE('',*,*,#23612,.F.);
#34008=ORIENTED_EDGE('',*,*,#23608,.F.);
#34009=ORIENTED_EDGE('',*,*,#23606,.T.);
#34010=ORIENTED_EDGE('',*,*,#23611,.T.);
#34011=ORIENTED_EDGE('',*,*,#23614,.F.);
#34012=ORIENTED_EDGE('',*,*,#23615,.T.);
#34013=ORIENTED_EDGE('',*,*,#23379,.T.);
#34014=ORIENTED_EDGE('',*,*,#23616,.F.);
#34015=ORIENTED_EDGE('',*,*,#23617,.F.);
#34016=ORIENTED_EDGE('',*,*,#23618,.F.);
#34017=ORIENTED_EDGE('',*,*,#23380,.F.);
#34018=ORIENTED_EDGE('',*,*,#23615,.F.);
#34019=ORIENTED_EDGE('',*,*,#23381,.F.);
#34020=ORIENTED_EDGE('',*,*,#23618,.T.);
#34021=ORIENTED_EDGE('',*,*,#23619,.T.);
#34022=ORIENTED_EDGE('',*,*,#23620,.T.);
#34023=ORIENTED_EDGE('',*,*,#23621,.F.);
#34024=ORIENTED_EDGE('',*,*,#23622,.F.);
#34025=ORIENTED_EDGE('',*,*,#23382,.F.);
#34026=ORIENTED_EDGE('',*,*,#23620,.F.);
#34027=ORIENTED_EDGE('',*,*,#23623,.T.);
#34028=ORIENTED_EDGE('',*,*,#23624,.F.);
#34029=ORIENTED_EDGE('',*,*,#23623,.F.);
#34030=ORIENTED_EDGE('',*,*,#23619,.F.);
#34031=ORIENTED_EDGE('',*,*,#23617,.T.);
#34032=ORIENTED_EDGE('',*,*,#23622,.T.);
#34033=ORIENTED_EDGE('',*,*,#23625,.F.);
#34034=ORIENTED_EDGE('',*,*,#23626,.T.);
#34035=ORIENTED_EDGE('',*,*,#23383,.T.);
#34036=ORIENTED_EDGE('',*,*,#23627,.F.);
#34037=ORIENTED_EDGE('',*,*,#23628,.F.);
#34038=ORIENTED_EDGE('',*,*,#23629,.F.);
#34039=ORIENTED_EDGE('',*,*,#23384,.F.);
#34040=ORIENTED_EDGE('',*,*,#23626,.F.);
#34041=ORIENTED_EDGE('',*,*,#23385,.F.);
#34042=ORIENTED_EDGE('',*,*,#23629,.T.);
#34043=ORIENTED_EDGE('',*,*,#23630,.T.);
#34044=ORIENTED_EDGE('',*,*,#23631,.T.);
#34045=ORIENTED_EDGE('',*,*,#23632,.F.);
#34046=ORIENTED_EDGE('',*,*,#23633,.F.);
#34047=ORIENTED_EDGE('',*,*,#23386,.F.);
#34048=ORIENTED_EDGE('',*,*,#23631,.F.);
#34049=ORIENTED_EDGE('',*,*,#23634,.T.);
#34050=ORIENTED_EDGE('',*,*,#23635,.F.);
#34051=ORIENTED_EDGE('',*,*,#23634,.F.);
#34052=ORIENTED_EDGE('',*,*,#23630,.F.);
#34053=ORIENTED_EDGE('',*,*,#23628,.T.);
#34054=ORIENTED_EDGE('',*,*,#23633,.T.);
#34055=ORIENTED_EDGE('',*,*,#23636,.F.);
#34056=ORIENTED_EDGE('',*,*,#23637,.T.);
#34057=ORIENTED_EDGE('',*,*,#23387,.T.);
#34058=ORIENTED_EDGE('',*,*,#23638,.F.);
#34059=ORIENTED_EDGE('',*,*,#23639,.F.);
#34060=ORIENTED_EDGE('',*,*,#23640,.F.);
#34061=ORIENTED_EDGE('',*,*,#23388,.F.);
#34062=ORIENTED_EDGE('',*,*,#23637,.F.);
#34063=ORIENTED_EDGE('',*,*,#23389,.F.);
#34064=ORIENTED_EDGE('',*,*,#23640,.T.);
#34065=ORIENTED_EDGE('',*,*,#23641,.T.);
#34066=ORIENTED_EDGE('',*,*,#23642,.T.);
#34067=ORIENTED_EDGE('',*,*,#23643,.F.);
#34068=ORIENTED_EDGE('',*,*,#23394,.F.);
#34069=ORIENTED_EDGE('',*,*,#23390,.F.);
#34070=ORIENTED_EDGE('',*,*,#23642,.F.);
#34071=ORIENTED_EDGE('',*,*,#23644,.T.);
#34072=ORIENTED_EDGE('',*,*,#23645,.F.);
#34073=ORIENTED_EDGE('',*,*,#23644,.F.);
#34074=ORIENTED_EDGE('',*,*,#23641,.F.);
#34075=ORIENTED_EDGE('',*,*,#23639,.T.);
#34076=ORIENTED_EDGE('',*,*,#23289,.F.);
#34077=ORIENTED_EDGE('',*,*,#23646,.T.);
#34078=ORIENTED_EDGE('',*,*,#23647,.F.);
#34079=ORIENTED_EDGE('',*,*,#23648,.F.);
#34080=ORIENTED_EDGE('',*,*,#23649,.F.);
#34081=ORIENTED_EDGE('',*,*,#23650,.F.);
#34082=ORIENTED_EDGE('',*,*,#23647,.T.);
#34083=ORIENTED_EDGE('',*,*,#23651,.T.);
#34084=ORIENTED_EDGE('',*,*,#23652,.F.);
#34085=ORIENTED_EDGE('',*,*,#23287,.F.);
#34086=ORIENTED_EDGE('',*,*,#23653,.F.);
#34087=ORIENTED_EDGE('',*,*,#23654,.F.);
#34088=ORIENTED_EDGE('',*,*,#23652,.T.);
#34089=ORIENTED_EDGE('',*,*,#23655,.T.);
#34090=ORIENTED_EDGE('',*,*,#23288,.F.);
#34091=ORIENTED_EDGE('',*,*,#23655,.F.);
#34092=ORIENTED_EDGE('',*,*,#23651,.F.);
#34093=ORIENTED_EDGE('',*,*,#23646,.F.);
#34094=ORIENTED_EDGE('',*,*,#23648,.T.);
#34095=ORIENTED_EDGE('',*,*,#23650,.T.);
#34096=ORIENTED_EDGE('',*,*,#23654,.T.);
#34097=ORIENTED_EDGE('',*,*,#23656,.F.);
#34098=ORIENTED_EDGE('',*,*,#23657,.T.);
#34099=ORIENTED_EDGE('',*,*,#23658,.T.);
#34100=ORIENTED_EDGE('',*,*,#23659,.T.);
#34101=ORIENTED_EDGE('',*,*,#23660,.F.);
#34102=ORIENTED_EDGE('',*,*,#23661,.T.);
#34103=ORIENTED_EDGE('',*,*,#23662,.T.);
#34104=ORIENTED_EDGE('',*,*,#23663,.T.);
#34105=ORIENTED_EDGE('',*,*,#23664,.F.);
#34106=ORIENTED_EDGE('',*,*,#23665,.T.);
#34107=ORIENTED_EDGE('',*,*,#23666,.T.);
#34108=ORIENTED_EDGE('',*,*,#23667,.T.);
#34109=ORIENTED_EDGE('',*,*,#23668,.F.);
#34110=ORIENTED_EDGE('',*,*,#23669,.T.);
#34111=ORIENTED_EDGE('',*,*,#23670,.T.);
#34112=ORIENTED_EDGE('',*,*,#23671,.T.);
#34113=ORIENTED_EDGE('',*,*,#23672,.F.);
#34114=ORIENTED_EDGE('',*,*,#23673,.T.);
#34115=ORIENTED_EDGE('',*,*,#23674,.T.);
#34116=ORIENTED_EDGE('',*,*,#23675,.T.);
#34117=ORIENTED_EDGE('',*,*,#23676,.F.);
#34118=ORIENTED_EDGE('',*,*,#23677,.T.);
#34119=ORIENTED_EDGE('',*,*,#23678,.T.);
#34120=ORIENTED_EDGE('',*,*,#23679,.T.);
#34121=ORIENTED_EDGE('',*,*,#23680,.F.);
#34122=ORIENTED_EDGE('',*,*,#23681,.T.);
#34123=ORIENTED_EDGE('',*,*,#23682,.T.);
#34124=ORIENTED_EDGE('',*,*,#23683,.T.);
#34125=ORIENTED_EDGE('',*,*,#23684,.F.);
#34126=ORIENTED_EDGE('',*,*,#23685,.T.);
#34127=ORIENTED_EDGE('',*,*,#23686,.T.);
#34128=ORIENTED_EDGE('',*,*,#23687,.T.);
#34129=ORIENTED_EDGE('',*,*,#23688,.F.);
#34130=ORIENTED_EDGE('',*,*,#23689,.T.);
#34131=ORIENTED_EDGE('',*,*,#23690,.T.);
#34132=ORIENTED_EDGE('',*,*,#23691,.T.);
#34133=ORIENTED_EDGE('',*,*,#23692,.F.);
#34134=ORIENTED_EDGE('',*,*,#23693,.T.);
#34135=ORIENTED_EDGE('',*,*,#23694,.T.);
#34136=ORIENTED_EDGE('',*,*,#23695,.T.);
#34137=ORIENTED_EDGE('',*,*,#23696,.F.);
#34138=ORIENTED_EDGE('',*,*,#23697,.T.);
#34139=ORIENTED_EDGE('',*,*,#23698,.T.);
#34140=ORIENTED_EDGE('',*,*,#23699,.T.);
#34141=ORIENTED_EDGE('',*,*,#23700,.F.);
#34142=ORIENTED_EDGE('',*,*,#23701,.T.);
#34143=ORIENTED_EDGE('',*,*,#23702,.T.);
#34144=ORIENTED_EDGE('',*,*,#23703,.T.);
#34145=ORIENTED_EDGE('',*,*,#23704,.F.);
#34146=ORIENTED_EDGE('',*,*,#23705,.T.);
#34147=ORIENTED_EDGE('',*,*,#23706,.T.);
#34148=ORIENTED_EDGE('',*,*,#23707,.T.);
#34149=ORIENTED_EDGE('',*,*,#23708,.F.);
#34150=ORIENTED_EDGE('',*,*,#23709,.T.);
#34151=ORIENTED_EDGE('',*,*,#23710,.T.);
#34152=ORIENTED_EDGE('',*,*,#23711,.T.);
#34153=ORIENTED_EDGE('',*,*,#23712,.F.);
#34154=ORIENTED_EDGE('',*,*,#23713,.T.);
#34155=ORIENTED_EDGE('',*,*,#23714,.T.);
#34156=ORIENTED_EDGE('',*,*,#23715,.T.);
#34157=ORIENTED_EDGE('',*,*,#23716,.F.);
#34158=ORIENTED_EDGE('',*,*,#23717,.T.);
#34159=ORIENTED_EDGE('',*,*,#23718,.T.);
#34160=ORIENTED_EDGE('',*,*,#23719,.T.);
#34161=ORIENTED_EDGE('',*,*,#23720,.F.);
#34162=ORIENTED_EDGE('',*,*,#23721,.T.);
#34163=ORIENTED_EDGE('',*,*,#23722,.T.);
#34164=ORIENTED_EDGE('',*,*,#23723,.T.);
#34165=ORIENTED_EDGE('',*,*,#23724,.F.);
#34166=ORIENTED_EDGE('',*,*,#23725,.T.);
#34167=ORIENTED_EDGE('',*,*,#23726,.T.);
#34168=ORIENTED_EDGE('',*,*,#23727,.T.);
#34169=ORIENTED_EDGE('',*,*,#23728,.F.);
#34170=ORIENTED_EDGE('',*,*,#23729,.T.);
#34171=ORIENTED_EDGE('',*,*,#23730,.T.);
#34172=ORIENTED_EDGE('',*,*,#23731,.T.);
#34173=ORIENTED_EDGE('',*,*,#23732,.F.);
#34174=ORIENTED_EDGE('',*,*,#23733,.T.);
#34175=ORIENTED_EDGE('',*,*,#23734,.T.);
#34176=ORIENTED_EDGE('',*,*,#23735,.T.);
#34177=ORIENTED_EDGE('',*,*,#23736,.F.);
#34178=ORIENTED_EDGE('',*,*,#23737,.T.);
#34179=ORIENTED_EDGE('',*,*,#23738,.T.);
#34180=ORIENTED_EDGE('',*,*,#23739,.T.);
#34181=ORIENTED_EDGE('',*,*,#23740,.F.);
#34182=ORIENTED_EDGE('',*,*,#23741,.T.);
#34183=ORIENTED_EDGE('',*,*,#23742,.T.);
#34184=ORIENTED_EDGE('',*,*,#23743,.T.);
#34185=ORIENTED_EDGE('',*,*,#23744,.F.);
#34186=ORIENTED_EDGE('',*,*,#23745,.T.);
#34187=ORIENTED_EDGE('',*,*,#23746,.T.);
#34188=ORIENTED_EDGE('',*,*,#23747,.T.);
#34189=ORIENTED_EDGE('',*,*,#23748,.F.);
#34190=ORIENTED_EDGE('',*,*,#23653,.T.);
#34191=ORIENTED_EDGE('',*,*,#23286,.F.);
#34192=ORIENTED_EDGE('',*,*,#23749,.T.);
#34193=ORIENTED_EDGE('',*,*,#23656,.T.);
#34194=ORIENTED_EDGE('',*,*,#23649,.T.);
#34195=ORIENTED_EDGE('',*,*,#23748,.T.);
#34196=ORIENTED_EDGE('',*,*,#23750,.T.);
#34197=ORIENTED_EDGE('',*,*,#23290,.F.);
#34198=ORIENTED_EDGE('',*,*,#23285,.F.);
#34199=ORIENTED_EDGE('',*,*,#23751,.T.);
#34200=ORIENTED_EDGE('',*,*,#23752,.F.);
#34201=ORIENTED_EDGE('',*,*,#23657,.F.);
#34202=ORIENTED_EDGE('',*,*,#23749,.F.);
#34203=ORIENTED_EDGE('',*,*,#23658,.F.);
#34204=ORIENTED_EDGE('',*,*,#23752,.T.);
#34205=ORIENTED_EDGE('',*,*,#23753,.T.);
#34206=ORIENTED_EDGE('',*,*,#23754,.F.);
#34207=ORIENTED_EDGE('',*,*,#23283,.F.);
#34208=ORIENTED_EDGE('',*,*,#23755,.F.);
#34209=ORIENTED_EDGE('',*,*,#23659,.F.);
#34210=ORIENTED_EDGE('',*,*,#23754,.T.);
#34211=ORIENTED_EDGE('',*,*,#23756,.T.);
#34212=ORIENTED_EDGE('',*,*,#23284,.F.);
#34213=ORIENTED_EDGE('',*,*,#23756,.F.);
#34214=ORIENTED_EDGE('',*,*,#23753,.F.);
#34215=ORIENTED_EDGE('',*,*,#23751,.F.);
#34216=ORIENTED_EDGE('',*,*,#23755,.T.);
#34217=ORIENTED_EDGE('',*,*,#23282,.F.);
#34218=ORIENTED_EDGE('',*,*,#23757,.T.);
#34219=ORIENTED_EDGE('',*,*,#23660,.T.);
#34220=ORIENTED_EDGE('',*,*,#23281,.F.);
#34221=ORIENTED_EDGE('',*,*,#23758,.T.);
#34222=ORIENTED_EDGE('',*,*,#23759,.F.);
#34223=ORIENTED_EDGE('',*,*,#23661,.F.);
#34224=ORIENTED_EDGE('',*,*,#23757,.F.);
#34225=ORIENTED_EDGE('',*,*,#23662,.F.);
#34226=ORIENTED_EDGE('',*,*,#23759,.T.);
#34227=ORIENTED_EDGE('',*,*,#23760,.T.);
#34228=ORIENTED_EDGE('',*,*,#23761,.F.);
#34229=ORIENTED_EDGE('',*,*,#23279,.F.);
#34230=ORIENTED_EDGE('',*,*,#23762,.F.);
#34231=ORIENTED_EDGE('',*,*,#23663,.F.);
#34232=ORIENTED_EDGE('',*,*,#23761,.T.);
#34233=ORIENTED_EDGE('',*,*,#23763,.T.);
#34234=ORIENTED_EDGE('',*,*,#23280,.F.);
#34235=ORIENTED_EDGE('',*,*,#23763,.F.);
#34236=ORIENTED_EDGE('',*,*,#23760,.F.);
#34237=ORIENTED_EDGE('',*,*,#23758,.F.);
#34238=ORIENTED_EDGE('',*,*,#23762,.T.);
#34239=ORIENTED_EDGE('',*,*,#23278,.F.);
#34240=ORIENTED_EDGE('',*,*,#23764,.T.);
#34241=ORIENTED_EDGE('',*,*,#23664,.T.);
#34242=ORIENTED_EDGE('',*,*,#23277,.F.);
#34243=ORIENTED_EDGE('',*,*,#23765,.T.);
#34244=ORIENTED_EDGE('',*,*,#23766,.F.);
#34245=ORIENTED_EDGE('',*,*,#23665,.F.);
#34246=ORIENTED_EDGE('',*,*,#23764,.F.);
#34247=ORIENTED_EDGE('',*,*,#23666,.F.);
#34248=ORIENTED_EDGE('',*,*,#23766,.T.);
#34249=ORIENTED_EDGE('',*,*,#23767,.T.);
#34250=ORIENTED_EDGE('',*,*,#23768,.F.);
#34251=ORIENTED_EDGE('',*,*,#23275,.F.);
#34252=ORIENTED_EDGE('',*,*,#23769,.F.);
#34253=ORIENTED_EDGE('',*,*,#23667,.F.);
#34254=ORIENTED_EDGE('',*,*,#23768,.T.);
#34255=ORIENTED_EDGE('',*,*,#23770,.T.);
#34256=ORIENTED_EDGE('',*,*,#23276,.F.);
#34257=ORIENTED_EDGE('',*,*,#23770,.F.);
#34258=ORIENTED_EDGE('',*,*,#23767,.F.);
#34259=ORIENTED_EDGE('',*,*,#23765,.F.);
#34260=ORIENTED_EDGE('',*,*,#23769,.T.);
#34261=ORIENTED_EDGE('',*,*,#23274,.F.);
#34262=ORIENTED_EDGE('',*,*,#23771,.T.);
#34263=ORIENTED_EDGE('',*,*,#23668,.T.);
#34264=ORIENTED_EDGE('',*,*,#23273,.F.);
#34265=ORIENTED_EDGE('',*,*,#23772,.T.);
#34266=ORIENTED_EDGE('',*,*,#23773,.F.);
#34267=ORIENTED_EDGE('',*,*,#23669,.F.);
#34268=ORIENTED_EDGE('',*,*,#23771,.F.);
#34269=ORIENTED_EDGE('',*,*,#23670,.F.);
#34270=ORIENTED_EDGE('',*,*,#23773,.T.);
#34271=ORIENTED_EDGE('',*,*,#23774,.T.);
#34272=ORIENTED_EDGE('',*,*,#23775,.F.);
#34273=ORIENTED_EDGE('',*,*,#23271,.F.);
#34274=ORIENTED_EDGE('',*,*,#23776,.F.);
#34275=ORIENTED_EDGE('',*,*,#23671,.F.);
#34276=ORIENTED_EDGE('',*,*,#23775,.T.);
#34277=ORIENTED_EDGE('',*,*,#23777,.T.);
#34278=ORIENTED_EDGE('',*,*,#23272,.F.);
#34279=ORIENTED_EDGE('',*,*,#23777,.F.);
#34280=ORIENTED_EDGE('',*,*,#23774,.F.);
#34281=ORIENTED_EDGE('',*,*,#23772,.F.);
#34282=ORIENTED_EDGE('',*,*,#23776,.T.);
#34283=ORIENTED_EDGE('',*,*,#23270,.F.);
#34284=ORIENTED_EDGE('',*,*,#23778,.T.);
#34285=ORIENTED_EDGE('',*,*,#23672,.T.);
#34286=ORIENTED_EDGE('',*,*,#23269,.F.);
#34287=ORIENTED_EDGE('',*,*,#23779,.T.);
#34288=ORIENTED_EDGE('',*,*,#23780,.F.);
#34289=ORIENTED_EDGE('',*,*,#23673,.F.);
#34290=ORIENTED_EDGE('',*,*,#23778,.F.);
#34291=ORIENTED_EDGE('',*,*,#23674,.F.);
#34292=ORIENTED_EDGE('',*,*,#23780,.T.);
#34293=ORIENTED_EDGE('',*,*,#23781,.T.);
#34294=ORIENTED_EDGE('',*,*,#23782,.F.);
#34295=ORIENTED_EDGE('',*,*,#23267,.F.);
#34296=ORIENTED_EDGE('',*,*,#23783,.F.);
#34297=ORIENTED_EDGE('',*,*,#23675,.F.);
#34298=ORIENTED_EDGE('',*,*,#23782,.T.);
#34299=ORIENTED_EDGE('',*,*,#23784,.T.);
#34300=ORIENTED_EDGE('',*,*,#23268,.F.);
#34301=ORIENTED_EDGE('',*,*,#23784,.F.);
#34302=ORIENTED_EDGE('',*,*,#23781,.F.);
#34303=ORIENTED_EDGE('',*,*,#23779,.F.);
#34304=ORIENTED_EDGE('',*,*,#23783,.T.);
#34305=ORIENTED_EDGE('',*,*,#23266,.F.);
#34306=ORIENTED_EDGE('',*,*,#23785,.T.);
#34307=ORIENTED_EDGE('',*,*,#23676,.T.);
#34308=ORIENTED_EDGE('',*,*,#23265,.F.);
#34309=ORIENTED_EDGE('',*,*,#23786,.T.);
#34310=ORIENTED_EDGE('',*,*,#23787,.F.);
#34311=ORIENTED_EDGE('',*,*,#23677,.F.);
#34312=ORIENTED_EDGE('',*,*,#23785,.F.);
#34313=ORIENTED_EDGE('',*,*,#23678,.F.);
#34314=ORIENTED_EDGE('',*,*,#23787,.T.);
#34315=ORIENTED_EDGE('',*,*,#23788,.T.);
#34316=ORIENTED_EDGE('',*,*,#23789,.F.);
#34317=ORIENTED_EDGE('',*,*,#23263,.F.);
#34318=ORIENTED_EDGE('',*,*,#23790,.F.);
#34319=ORIENTED_EDGE('',*,*,#23679,.F.);
#34320=ORIENTED_EDGE('',*,*,#23789,.T.);
#34321=ORIENTED_EDGE('',*,*,#23791,.T.);
#34322=ORIENTED_EDGE('',*,*,#23264,.F.);
#34323=ORIENTED_EDGE('',*,*,#23791,.F.);
#34324=ORIENTED_EDGE('',*,*,#23788,.F.);
#34325=ORIENTED_EDGE('',*,*,#23786,.F.);
#34326=ORIENTED_EDGE('',*,*,#23790,.T.);
#34327=ORIENTED_EDGE('',*,*,#23262,.F.);
#34328=ORIENTED_EDGE('',*,*,#23792,.T.);
#34329=ORIENTED_EDGE('',*,*,#23680,.T.);
#34330=ORIENTED_EDGE('',*,*,#23261,.F.);
#34331=ORIENTED_EDGE('',*,*,#23793,.T.);
#34332=ORIENTED_EDGE('',*,*,#23794,.F.);
#34333=ORIENTED_EDGE('',*,*,#23681,.F.);
#34334=ORIENTED_EDGE('',*,*,#23792,.F.);
#34335=ORIENTED_EDGE('',*,*,#23682,.F.);
#34336=ORIENTED_EDGE('',*,*,#23794,.T.);
#34337=ORIENTED_EDGE('',*,*,#23795,.T.);
#34338=ORIENTED_EDGE('',*,*,#23796,.F.);
#34339=ORIENTED_EDGE('',*,*,#23259,.F.);
#34340=ORIENTED_EDGE('',*,*,#23797,.F.);
#34341=ORIENTED_EDGE('',*,*,#23683,.F.);
#34342=ORIENTED_EDGE('',*,*,#23796,.T.);
#34343=ORIENTED_EDGE('',*,*,#23798,.T.);
#34344=ORIENTED_EDGE('',*,*,#23260,.F.);
#34345=ORIENTED_EDGE('',*,*,#23798,.F.);
#34346=ORIENTED_EDGE('',*,*,#23795,.F.);
#34347=ORIENTED_EDGE('',*,*,#23793,.F.);
#34348=ORIENTED_EDGE('',*,*,#23797,.T.);
#34349=ORIENTED_EDGE('',*,*,#23258,.F.);
#34350=ORIENTED_EDGE('',*,*,#23799,.T.);
#34351=ORIENTED_EDGE('',*,*,#23684,.T.);
#34352=ORIENTED_EDGE('',*,*,#23257,.F.);
#34353=ORIENTED_EDGE('',*,*,#23800,.T.);
#34354=ORIENTED_EDGE('',*,*,#23801,.F.);
#34355=ORIENTED_EDGE('',*,*,#23685,.F.);
#34356=ORIENTED_EDGE('',*,*,#23799,.F.);
#34357=ORIENTED_EDGE('',*,*,#23686,.F.);
#34358=ORIENTED_EDGE('',*,*,#23801,.T.);
#34359=ORIENTED_EDGE('',*,*,#23802,.T.);
#34360=ORIENTED_EDGE('',*,*,#23803,.F.);
#34361=ORIENTED_EDGE('',*,*,#23255,.F.);
#34362=ORIENTED_EDGE('',*,*,#23804,.F.);
#34363=ORIENTED_EDGE('',*,*,#23687,.F.);
#34364=ORIENTED_EDGE('',*,*,#23803,.T.);
#34365=ORIENTED_EDGE('',*,*,#23805,.T.);
#34366=ORIENTED_EDGE('',*,*,#23256,.F.);
#34367=ORIENTED_EDGE('',*,*,#23805,.F.);
#34368=ORIENTED_EDGE('',*,*,#23802,.F.);
#34369=ORIENTED_EDGE('',*,*,#23800,.F.);
#34370=ORIENTED_EDGE('',*,*,#23804,.T.);
#34371=ORIENTED_EDGE('',*,*,#23254,.F.);
#34372=ORIENTED_EDGE('',*,*,#23806,.T.);
#34373=ORIENTED_EDGE('',*,*,#23688,.T.);
#34374=ORIENTED_EDGE('',*,*,#23253,.F.);
#34375=ORIENTED_EDGE('',*,*,#23807,.T.);
#34376=ORIENTED_EDGE('',*,*,#23808,.F.);
#34377=ORIENTED_EDGE('',*,*,#23689,.F.);
#34378=ORIENTED_EDGE('',*,*,#23806,.F.);
#34379=ORIENTED_EDGE('',*,*,#23690,.F.);
#34380=ORIENTED_EDGE('',*,*,#23808,.T.);
#34381=ORIENTED_EDGE('',*,*,#23809,.T.);
#34382=ORIENTED_EDGE('',*,*,#23810,.F.);
#34383=ORIENTED_EDGE('',*,*,#23251,.F.);
#34384=ORIENTED_EDGE('',*,*,#23811,.F.);
#34385=ORIENTED_EDGE('',*,*,#23691,.F.);
#34386=ORIENTED_EDGE('',*,*,#23810,.T.);
#34387=ORIENTED_EDGE('',*,*,#23812,.T.);
#34388=ORIENTED_EDGE('',*,*,#23252,.F.);
#34389=ORIENTED_EDGE('',*,*,#23812,.F.);
#34390=ORIENTED_EDGE('',*,*,#23809,.F.);
#34391=ORIENTED_EDGE('',*,*,#23807,.F.);
#34392=ORIENTED_EDGE('',*,*,#23811,.T.);
#34393=ORIENTED_EDGE('',*,*,#23250,.F.);
#34394=ORIENTED_EDGE('',*,*,#23813,.T.);
#34395=ORIENTED_EDGE('',*,*,#23692,.T.);
#34396=ORIENTED_EDGE('',*,*,#23249,.F.);
#34397=ORIENTED_EDGE('',*,*,#23814,.T.);
#34398=ORIENTED_EDGE('',*,*,#23815,.F.);
#34399=ORIENTED_EDGE('',*,*,#23693,.F.);
#34400=ORIENTED_EDGE('',*,*,#23813,.F.);
#34401=ORIENTED_EDGE('',*,*,#23694,.F.);
#34402=ORIENTED_EDGE('',*,*,#23815,.T.);
#34403=ORIENTED_EDGE('',*,*,#23816,.T.);
#34404=ORIENTED_EDGE('',*,*,#23817,.F.);
#34405=ORIENTED_EDGE('',*,*,#23247,.F.);
#34406=ORIENTED_EDGE('',*,*,#23818,.F.);
#34407=ORIENTED_EDGE('',*,*,#23695,.F.);
#34408=ORIENTED_EDGE('',*,*,#23817,.T.);
#34409=ORIENTED_EDGE('',*,*,#23819,.T.);
#34410=ORIENTED_EDGE('',*,*,#23248,.F.);
#34411=ORIENTED_EDGE('',*,*,#23819,.F.);
#34412=ORIENTED_EDGE('',*,*,#23816,.F.);
#34413=ORIENTED_EDGE('',*,*,#23814,.F.);
#34414=ORIENTED_EDGE('',*,*,#23818,.T.);
#34415=ORIENTED_EDGE('',*,*,#23246,.F.);
#34416=ORIENTED_EDGE('',*,*,#23820,.T.);
#34417=ORIENTED_EDGE('',*,*,#23696,.T.);
#34418=ORIENTED_EDGE('',*,*,#23245,.F.);
#34419=ORIENTED_EDGE('',*,*,#23821,.T.);
#34420=ORIENTED_EDGE('',*,*,#23822,.F.);
#34421=ORIENTED_EDGE('',*,*,#23697,.F.);
#34422=ORIENTED_EDGE('',*,*,#23820,.F.);
#34423=ORIENTED_EDGE('',*,*,#23698,.F.);
#34424=ORIENTED_EDGE('',*,*,#23822,.T.);
#34425=ORIENTED_EDGE('',*,*,#23823,.T.);
#34426=ORIENTED_EDGE('',*,*,#23824,.F.);
#34427=ORIENTED_EDGE('',*,*,#23339,.F.);
#34428=ORIENTED_EDGE('',*,*,#23825,.F.);
#34429=ORIENTED_EDGE('',*,*,#23699,.F.);
#34430=ORIENTED_EDGE('',*,*,#23824,.T.);
#34431=ORIENTED_EDGE('',*,*,#23826,.T.);
#34432=ORIENTED_EDGE('',*,*,#23340,.F.);
#34433=ORIENTED_EDGE('',*,*,#23826,.F.);
#34434=ORIENTED_EDGE('',*,*,#23823,.F.);
#34435=ORIENTED_EDGE('',*,*,#23821,.F.);
#34436=ORIENTED_EDGE('',*,*,#23244,.F.);
#34437=ORIENTED_EDGE('',*,*,#23825,.T.);
#34438=ORIENTED_EDGE('',*,*,#23338,.F.);
#34439=ORIENTED_EDGE('',*,*,#23827,.T.);
#34440=ORIENTED_EDGE('',*,*,#23700,.T.);
#34441=ORIENTED_EDGE('',*,*,#23337,.F.);
#34442=ORIENTED_EDGE('',*,*,#23828,.T.);
#34443=ORIENTED_EDGE('',*,*,#23829,.F.);
#34444=ORIENTED_EDGE('',*,*,#23701,.F.);
#34445=ORIENTED_EDGE('',*,*,#23827,.F.);
#34446=ORIENTED_EDGE('',*,*,#23702,.F.);
#34447=ORIENTED_EDGE('',*,*,#23829,.T.);
#34448=ORIENTED_EDGE('',*,*,#23830,.T.);
#34449=ORIENTED_EDGE('',*,*,#23831,.F.);
#34450=ORIENTED_EDGE('',*,*,#23335,.F.);
#34451=ORIENTED_EDGE('',*,*,#23832,.F.);
#34452=ORIENTED_EDGE('',*,*,#23703,.F.);
#34453=ORIENTED_EDGE('',*,*,#23831,.T.);
#34454=ORIENTED_EDGE('',*,*,#23833,.T.);
#34455=ORIENTED_EDGE('',*,*,#23336,.F.);
#34456=ORIENTED_EDGE('',*,*,#23833,.F.);
#34457=ORIENTED_EDGE('',*,*,#23830,.F.);
#34458=ORIENTED_EDGE('',*,*,#23828,.F.);
#34459=ORIENTED_EDGE('',*,*,#23832,.T.);
#34460=ORIENTED_EDGE('',*,*,#23334,.F.);
#34461=ORIENTED_EDGE('',*,*,#23834,.T.);
#34462=ORIENTED_EDGE('',*,*,#23704,.T.);
#34463=ORIENTED_EDGE('',*,*,#23333,.F.);
#34464=ORIENTED_EDGE('',*,*,#23835,.T.);
#34465=ORIENTED_EDGE('',*,*,#23836,.F.);
#34466=ORIENTED_EDGE('',*,*,#23705,.F.);
#34467=ORIENTED_EDGE('',*,*,#23834,.F.);
#34468=ORIENTED_EDGE('',*,*,#23706,.F.);
#34469=ORIENTED_EDGE('',*,*,#23836,.T.);
#34470=ORIENTED_EDGE('',*,*,#23837,.T.);
#34471=ORIENTED_EDGE('',*,*,#23838,.F.);
#34472=ORIENTED_EDGE('',*,*,#23331,.F.);
#34473=ORIENTED_EDGE('',*,*,#23839,.F.);
#34474=ORIENTED_EDGE('',*,*,#23707,.F.);
#34475=ORIENTED_EDGE('',*,*,#23838,.T.);
#34476=ORIENTED_EDGE('',*,*,#23840,.T.);
#34477=ORIENTED_EDGE('',*,*,#23332,.F.);
#34478=ORIENTED_EDGE('',*,*,#23840,.F.);
#34479=ORIENTED_EDGE('',*,*,#23837,.F.);
#34480=ORIENTED_EDGE('',*,*,#23835,.F.);
#34481=ORIENTED_EDGE('',*,*,#23839,.T.);
#34482=ORIENTED_EDGE('',*,*,#23330,.F.);
#34483=ORIENTED_EDGE('',*,*,#23841,.T.);
#34484=ORIENTED_EDGE('',*,*,#23708,.T.);
#34485=ORIENTED_EDGE('',*,*,#23329,.F.);
#34486=ORIENTED_EDGE('',*,*,#23842,.T.);
#34487=ORIENTED_EDGE('',*,*,#23843,.F.);
#34488=ORIENTED_EDGE('',*,*,#23709,.F.);
#34489=ORIENTED_EDGE('',*,*,#23841,.F.);
#34490=ORIENTED_EDGE('',*,*,#23710,.F.);
#34491=ORIENTED_EDGE('',*,*,#23843,.T.);
#34492=ORIENTED_EDGE('',*,*,#23844,.T.);
#34493=ORIENTED_EDGE('',*,*,#23845,.F.);
#34494=ORIENTED_EDGE('',*,*,#23327,.F.);
#34495=ORIENTED_EDGE('',*,*,#23846,.F.);
#34496=ORIENTED_EDGE('',*,*,#23711,.F.);
#34497=ORIENTED_EDGE('',*,*,#23845,.T.);
#34498=ORIENTED_EDGE('',*,*,#23847,.T.);
#34499=ORIENTED_EDGE('',*,*,#23328,.F.);
#34500=ORIENTED_EDGE('',*,*,#23847,.F.);
#34501=ORIENTED_EDGE('',*,*,#23844,.F.);
#34502=ORIENTED_EDGE('',*,*,#23842,.F.);
#34503=ORIENTED_EDGE('',*,*,#23846,.T.);
#34504=ORIENTED_EDGE('',*,*,#23326,.F.);
#34505=ORIENTED_EDGE('',*,*,#23848,.T.);
#34506=ORIENTED_EDGE('',*,*,#23712,.T.);
#34507=ORIENTED_EDGE('',*,*,#23325,.F.);
#34508=ORIENTED_EDGE('',*,*,#23849,.T.);
#34509=ORIENTED_EDGE('',*,*,#23850,.F.);
#34510=ORIENTED_EDGE('',*,*,#23713,.F.);
#34511=ORIENTED_EDGE('',*,*,#23848,.F.);
#34512=ORIENTED_EDGE('',*,*,#23714,.F.);
#34513=ORIENTED_EDGE('',*,*,#23850,.T.);
#34514=ORIENTED_EDGE('',*,*,#23851,.T.);
#34515=ORIENTED_EDGE('',*,*,#23852,.F.);
#34516=ORIENTED_EDGE('',*,*,#23323,.F.);
#34517=ORIENTED_EDGE('',*,*,#23853,.F.);
#34518=ORIENTED_EDGE('',*,*,#23715,.F.);
#34519=ORIENTED_EDGE('',*,*,#23852,.T.);
#34520=ORIENTED_EDGE('',*,*,#23854,.T.);
#34521=ORIENTED_EDGE('',*,*,#23324,.F.);
#34522=ORIENTED_EDGE('',*,*,#23854,.F.);
#34523=ORIENTED_EDGE('',*,*,#23851,.F.);
#34524=ORIENTED_EDGE('',*,*,#23849,.F.);
#34525=ORIENTED_EDGE('',*,*,#23853,.T.);
#34526=ORIENTED_EDGE('',*,*,#23322,.F.);
#34527=ORIENTED_EDGE('',*,*,#23855,.T.);
#34528=ORIENTED_EDGE('',*,*,#23716,.T.);
#34529=ORIENTED_EDGE('',*,*,#23321,.F.);
#34530=ORIENTED_EDGE('',*,*,#23856,.T.);
#34531=ORIENTED_EDGE('',*,*,#23857,.F.);
#34532=ORIENTED_EDGE('',*,*,#23717,.F.);
#34533=ORIENTED_EDGE('',*,*,#23855,.F.);
#34534=ORIENTED_EDGE('',*,*,#23718,.F.);
#34535=ORIENTED_EDGE('',*,*,#23857,.T.);
#34536=ORIENTED_EDGE('',*,*,#23858,.T.);
#34537=ORIENTED_EDGE('',*,*,#23859,.F.);
#34538=ORIENTED_EDGE('',*,*,#23319,.F.);
#34539=ORIENTED_EDGE('',*,*,#23860,.F.);
#34540=ORIENTED_EDGE('',*,*,#23719,.F.);
#34541=ORIENTED_EDGE('',*,*,#23859,.T.);
#34542=ORIENTED_EDGE('',*,*,#23861,.T.);
#34543=ORIENTED_EDGE('',*,*,#23320,.F.);
#34544=ORIENTED_EDGE('',*,*,#23861,.F.);
#34545=ORIENTED_EDGE('',*,*,#23858,.F.);
#34546=ORIENTED_EDGE('',*,*,#23856,.F.);
#34547=ORIENTED_EDGE('',*,*,#23860,.T.);
#34548=ORIENTED_EDGE('',*,*,#23318,.F.);
#34549=ORIENTED_EDGE('',*,*,#23862,.T.);
#34550=ORIENTED_EDGE('',*,*,#23720,.T.);
#34551=ORIENTED_EDGE('',*,*,#23317,.F.);
#34552=ORIENTED_EDGE('',*,*,#23863,.T.);
#34553=ORIENTED_EDGE('',*,*,#23864,.F.);
#34554=ORIENTED_EDGE('',*,*,#23721,.F.);
#34555=ORIENTED_EDGE('',*,*,#23862,.F.);
#34556=ORIENTED_EDGE('',*,*,#23722,.F.);
#34557=ORIENTED_EDGE('',*,*,#23864,.T.);
#34558=ORIENTED_EDGE('',*,*,#23865,.T.);
#34559=ORIENTED_EDGE('',*,*,#23866,.F.);
#34560=ORIENTED_EDGE('',*,*,#23315,.F.);
#34561=ORIENTED_EDGE('',*,*,#23867,.F.);
#34562=ORIENTED_EDGE('',*,*,#23723,.F.);
#34563=ORIENTED_EDGE('',*,*,#23866,.T.);
#34564=ORIENTED_EDGE('',*,*,#23868,.T.);
#34565=ORIENTED_EDGE('',*,*,#23316,.F.);
#34566=ORIENTED_EDGE('',*,*,#23868,.F.);
#34567=ORIENTED_EDGE('',*,*,#23865,.F.);
#34568=ORIENTED_EDGE('',*,*,#23863,.F.);
#34569=ORIENTED_EDGE('',*,*,#23867,.T.);
#34570=ORIENTED_EDGE('',*,*,#23314,.F.);
#34571=ORIENTED_EDGE('',*,*,#23869,.T.);
#34572=ORIENTED_EDGE('',*,*,#23724,.T.);
#34573=ORIENTED_EDGE('',*,*,#23313,.F.);
#34574=ORIENTED_EDGE('',*,*,#23870,.T.);
#34575=ORIENTED_EDGE('',*,*,#23871,.F.);
#34576=ORIENTED_EDGE('',*,*,#23725,.F.);
#34577=ORIENTED_EDGE('',*,*,#23869,.F.);
#34578=ORIENTED_EDGE('',*,*,#23726,.F.);
#34579=ORIENTED_EDGE('',*,*,#23871,.T.);
#34580=ORIENTED_EDGE('',*,*,#23872,.T.);
#34581=ORIENTED_EDGE('',*,*,#23873,.F.);
#34582=ORIENTED_EDGE('',*,*,#23311,.F.);
#34583=ORIENTED_EDGE('',*,*,#23874,.F.);
#34584=ORIENTED_EDGE('',*,*,#23727,.F.);
#34585=ORIENTED_EDGE('',*,*,#23873,.T.);
#34586=ORIENTED_EDGE('',*,*,#23875,.T.);
#34587=ORIENTED_EDGE('',*,*,#23312,.F.);
#34588=ORIENTED_EDGE('',*,*,#23875,.F.);
#34589=ORIENTED_EDGE('',*,*,#23872,.F.);
#34590=ORIENTED_EDGE('',*,*,#23870,.F.);
#34591=ORIENTED_EDGE('',*,*,#23874,.T.);
#34592=ORIENTED_EDGE('',*,*,#23310,.F.);
#34593=ORIENTED_EDGE('',*,*,#23876,.T.);
#34594=ORIENTED_EDGE('',*,*,#23728,.T.);
#34595=ORIENTED_EDGE('',*,*,#23309,.F.);
#34596=ORIENTED_EDGE('',*,*,#23877,.T.);
#34597=ORIENTED_EDGE('',*,*,#23878,.F.);
#34598=ORIENTED_EDGE('',*,*,#23729,.F.);
#34599=ORIENTED_EDGE('',*,*,#23876,.F.);
#34600=ORIENTED_EDGE('',*,*,#23730,.F.);
#34601=ORIENTED_EDGE('',*,*,#23878,.T.);
#34602=ORIENTED_EDGE('',*,*,#23879,.T.);
#34603=ORIENTED_EDGE('',*,*,#23880,.F.);
#34604=ORIENTED_EDGE('',*,*,#23307,.F.);
#34605=ORIENTED_EDGE('',*,*,#23881,.F.);
#34606=ORIENTED_EDGE('',*,*,#23731,.F.);
#34607=ORIENTED_EDGE('',*,*,#23880,.T.);
#34608=ORIENTED_EDGE('',*,*,#23882,.T.);
#34609=ORIENTED_EDGE('',*,*,#23308,.F.);
#34610=ORIENTED_EDGE('',*,*,#23882,.F.);
#34611=ORIENTED_EDGE('',*,*,#23879,.F.);
#34612=ORIENTED_EDGE('',*,*,#23877,.F.);
#34613=ORIENTED_EDGE('',*,*,#23881,.T.);
#34614=ORIENTED_EDGE('',*,*,#23306,.F.);
#34615=ORIENTED_EDGE('',*,*,#23883,.T.);
#34616=ORIENTED_EDGE('',*,*,#23732,.T.);
#34617=ORIENTED_EDGE('',*,*,#23305,.F.);
#34618=ORIENTED_EDGE('',*,*,#23884,.T.);
#34619=ORIENTED_EDGE('',*,*,#23885,.F.);
#34620=ORIENTED_EDGE('',*,*,#23733,.F.);
#34621=ORIENTED_EDGE('',*,*,#23883,.F.);
#34622=ORIENTED_EDGE('',*,*,#23734,.F.);
#34623=ORIENTED_EDGE('',*,*,#23885,.T.);
#34624=ORIENTED_EDGE('',*,*,#23886,.T.);
#34625=ORIENTED_EDGE('',*,*,#23887,.F.);
#34626=ORIENTED_EDGE('',*,*,#23303,.F.);
#34627=ORIENTED_EDGE('',*,*,#23888,.F.);
#34628=ORIENTED_EDGE('',*,*,#23735,.F.);
#34629=ORIENTED_EDGE('',*,*,#23887,.T.);
#34630=ORIENTED_EDGE('',*,*,#23889,.T.);
#34631=ORIENTED_EDGE('',*,*,#23304,.F.);
#34632=ORIENTED_EDGE('',*,*,#23889,.F.);
#34633=ORIENTED_EDGE('',*,*,#23886,.F.);
#34634=ORIENTED_EDGE('',*,*,#23884,.F.);
#34635=ORIENTED_EDGE('',*,*,#23888,.T.);
#34636=ORIENTED_EDGE('',*,*,#23302,.F.);
#34637=ORIENTED_EDGE('',*,*,#23890,.T.);
#34638=ORIENTED_EDGE('',*,*,#23736,.T.);
#34639=ORIENTED_EDGE('',*,*,#23301,.F.);
#34640=ORIENTED_EDGE('',*,*,#23891,.T.);
#34641=ORIENTED_EDGE('',*,*,#23892,.F.);
#34642=ORIENTED_EDGE('',*,*,#23737,.F.);
#34643=ORIENTED_EDGE('',*,*,#23890,.F.);
#34644=ORIENTED_EDGE('',*,*,#23738,.F.);
#34645=ORIENTED_EDGE('',*,*,#23892,.T.);
#34646=ORIENTED_EDGE('',*,*,#23893,.T.);
#34647=ORIENTED_EDGE('',*,*,#23894,.F.);
#34648=ORIENTED_EDGE('',*,*,#23299,.F.);
#34649=ORIENTED_EDGE('',*,*,#23895,.F.);
#34650=ORIENTED_EDGE('',*,*,#23739,.F.);
#34651=ORIENTED_EDGE('',*,*,#23894,.T.);
#34652=ORIENTED_EDGE('',*,*,#23896,.T.);
#34653=ORIENTED_EDGE('',*,*,#23300,.F.);
#34654=ORIENTED_EDGE('',*,*,#23896,.F.);
#34655=ORIENTED_EDGE('',*,*,#23893,.F.);
#34656=ORIENTED_EDGE('',*,*,#23891,.F.);
#34657=ORIENTED_EDGE('',*,*,#23895,.T.);
#34658=ORIENTED_EDGE('',*,*,#23298,.F.);
#34659=ORIENTED_EDGE('',*,*,#23897,.T.);
#34660=ORIENTED_EDGE('',*,*,#23740,.T.);
#34661=ORIENTED_EDGE('',*,*,#23297,.F.);
#34662=ORIENTED_EDGE('',*,*,#23898,.T.);
#34663=ORIENTED_EDGE('',*,*,#23899,.F.);
#34664=ORIENTED_EDGE('',*,*,#23741,.F.);
#34665=ORIENTED_EDGE('',*,*,#23897,.F.);
#34666=ORIENTED_EDGE('',*,*,#23742,.F.);
#34667=ORIENTED_EDGE('',*,*,#23899,.T.);
#34668=ORIENTED_EDGE('',*,*,#23900,.T.);
#34669=ORIENTED_EDGE('',*,*,#23901,.F.);
#34670=ORIENTED_EDGE('',*,*,#23295,.F.);
#34671=ORIENTED_EDGE('',*,*,#23902,.F.);
#34672=ORIENTED_EDGE('',*,*,#23743,.F.);
#34673=ORIENTED_EDGE('',*,*,#23901,.T.);
#34674=ORIENTED_EDGE('',*,*,#23903,.T.);
#34675=ORIENTED_EDGE('',*,*,#23296,.F.);
#34676=ORIENTED_EDGE('',*,*,#23903,.F.);
#34677=ORIENTED_EDGE('',*,*,#23900,.F.);
#34678=ORIENTED_EDGE('',*,*,#23898,.F.);
#34679=ORIENTED_EDGE('',*,*,#23902,.T.);
#34680=ORIENTED_EDGE('',*,*,#23294,.F.);
#34681=ORIENTED_EDGE('',*,*,#23904,.T.);
#34682=ORIENTED_EDGE('',*,*,#23744,.T.);
#34683=ORIENTED_EDGE('',*,*,#23293,.F.);
#34684=ORIENTED_EDGE('',*,*,#23905,.T.);
#34685=ORIENTED_EDGE('',*,*,#23906,.F.);
#34686=ORIENTED_EDGE('',*,*,#23745,.F.);
#34687=ORIENTED_EDGE('',*,*,#23904,.F.);
#34688=ORIENTED_EDGE('',*,*,#23746,.F.);
#34689=ORIENTED_EDGE('',*,*,#23906,.T.);
#34690=ORIENTED_EDGE('',*,*,#23907,.T.);
#34691=ORIENTED_EDGE('',*,*,#23908,.F.);
#34692=ORIENTED_EDGE('',*,*,#23291,.F.);
#34693=ORIENTED_EDGE('',*,*,#23750,.F.);
#34694=ORIENTED_EDGE('',*,*,#23747,.F.);
#34695=ORIENTED_EDGE('',*,*,#23908,.T.);
#34696=ORIENTED_EDGE('',*,*,#23909,.T.);
#34697=ORIENTED_EDGE('',*,*,#23292,.F.);
#34698=ORIENTED_EDGE('',*,*,#23909,.F.);
#34699=ORIENTED_EDGE('',*,*,#23907,.F.);
#34700=ORIENTED_EDGE('',*,*,#23905,.F.);
#34701=ORIENTED_EDGE('',*,*,#23187,.T.);
#34702=ORIENTED_EDGE('',*,*,#23395,.T.);
#34703=ORIENTED_EDGE('',*,*,#23643,.T.);
#34704=ORIENTED_EDGE('',*,*,#23645,.T.);
#34705=ORIENTED_EDGE('',*,*,#23638,.T.);
#34706=ORIENTED_EDGE('',*,*,#23636,.T.);
#34707=ORIENTED_EDGE('',*,*,#23632,.T.);
#34708=ORIENTED_EDGE('',*,*,#23635,.T.);
#34709=ORIENTED_EDGE('',*,*,#23627,.T.);
#34710=ORIENTED_EDGE('',*,*,#23625,.T.);
#34711=ORIENTED_EDGE('',*,*,#23621,.T.);
#34712=ORIENTED_EDGE('',*,*,#23624,.T.);
#34713=ORIENTED_EDGE('',*,*,#23616,.T.);
#34714=ORIENTED_EDGE('',*,*,#23614,.T.);
#34715=ORIENTED_EDGE('',*,*,#23610,.T.);
#34716=ORIENTED_EDGE('',*,*,#23613,.T.);
#34717=ORIENTED_EDGE('',*,*,#23605,.T.);
#34718=ORIENTED_EDGE('',*,*,#23603,.T.);
#34719=ORIENTED_EDGE('',*,*,#23599,.T.);
#34720=ORIENTED_EDGE('',*,*,#23602,.T.);
#34721=ORIENTED_EDGE('',*,*,#23594,.T.);
#34722=ORIENTED_EDGE('',*,*,#23592,.T.);
#34723=ORIENTED_EDGE('',*,*,#23588,.T.);
#34724=ORIENTED_EDGE('',*,*,#23591,.T.);
#34725=ORIENTED_EDGE('',*,*,#23583,.T.);
#34726=ORIENTED_EDGE('',*,*,#23581,.T.);
#34727=ORIENTED_EDGE('',*,*,#23577,.T.);
#34728=ORIENTED_EDGE('',*,*,#23580,.T.);
#34729=ORIENTED_EDGE('',*,*,#23572,.T.);
#34730=ORIENTED_EDGE('',*,*,#23570,.T.);
#34731=ORIENTED_EDGE('',*,*,#23566,.T.);
#34732=ORIENTED_EDGE('',*,*,#23569,.T.);
#34733=ORIENTED_EDGE('',*,*,#23561,.T.);
#34734=ORIENTED_EDGE('',*,*,#23559,.T.);
#34735=ORIENTED_EDGE('',*,*,#23555,.T.);
#34736=ORIENTED_EDGE('',*,*,#23558,.T.);
#34737=ORIENTED_EDGE('',*,*,#23550,.T.);
#34738=ORIENTED_EDGE('',*,*,#23548,.T.);
#34739=ORIENTED_EDGE('',*,*,#23544,.T.);
#34740=ORIENTED_EDGE('',*,*,#23547,.T.);
#34741=ORIENTED_EDGE('',*,*,#23539,.T.);
#34742=ORIENTED_EDGE('',*,*,#23537,.T.);
#34743=ORIENTED_EDGE('',*,*,#23533,.T.);
#34744=ORIENTED_EDGE('',*,*,#23536,.T.);
#34745=ORIENTED_EDGE('',*,*,#23528,.T.);
#34746=ORIENTED_EDGE('',*,*,#23526,.T.);
#34747=ORIENTED_EDGE('',*,*,#23522,.T.);
#34748=ORIENTED_EDGE('',*,*,#23525,.T.);
#34749=ORIENTED_EDGE('',*,*,#23517,.T.);
#34750=ORIENTED_EDGE('',*,*,#23515,.T.);
#34751=ORIENTED_EDGE('',*,*,#23511,.T.);
#34752=ORIENTED_EDGE('',*,*,#23514,.T.);
#34753=ORIENTED_EDGE('',*,*,#23506,.T.);
#34754=ORIENTED_EDGE('',*,*,#23504,.T.);
#34755=ORIENTED_EDGE('',*,*,#23500,.T.);
#34756=ORIENTED_EDGE('',*,*,#23503,.T.);
#34757=ORIENTED_EDGE('',*,*,#23495,.T.);
#34758=ORIENTED_EDGE('',*,*,#23493,.T.);
#34759=ORIENTED_EDGE('',*,*,#23489,.T.);
#34760=ORIENTED_EDGE('',*,*,#23492,.T.);
#34761=ORIENTED_EDGE('',*,*,#23484,.T.);
#34762=ORIENTED_EDGE('',*,*,#23482,.T.);
#34763=ORIENTED_EDGE('',*,*,#23478,.T.);
#34764=ORIENTED_EDGE('',*,*,#23481,.T.);
#34765=ORIENTED_EDGE('',*,*,#23473,.T.);
#34766=ORIENTED_EDGE('',*,*,#23471,.T.);
#34767=ORIENTED_EDGE('',*,*,#23467,.T.);
#34768=ORIENTED_EDGE('',*,*,#23470,.T.);
#34769=ORIENTED_EDGE('',*,*,#23462,.T.);
#34770=ORIENTED_EDGE('',*,*,#23460,.T.);
#34771=ORIENTED_EDGE('',*,*,#23456,.T.);
#34772=ORIENTED_EDGE('',*,*,#23459,.T.);
#34773=ORIENTED_EDGE('',*,*,#23451,.T.);
#34774=ORIENTED_EDGE('',*,*,#23449,.T.);
#34775=ORIENTED_EDGE('',*,*,#23445,.T.);
#34776=ORIENTED_EDGE('',*,*,#23448,.T.);
#34777=ORIENTED_EDGE('',*,*,#23440,.T.);
#34778=ORIENTED_EDGE('',*,*,#23438,.T.);
#34779=ORIENTED_EDGE('',*,*,#23434,.T.);
#34780=ORIENTED_EDGE('',*,*,#23437,.T.);
#34781=ORIENTED_EDGE('',*,*,#23429,.T.);
#34782=ORIENTED_EDGE('',*,*,#23427,.T.);
#34783=ORIENTED_EDGE('',*,*,#23423,.T.);
#34784=ORIENTED_EDGE('',*,*,#23426,.T.);
#34785=ORIENTED_EDGE('',*,*,#23418,.T.);
#34786=ORIENTED_EDGE('',*,*,#23416,.T.);
#34787=ORIENTED_EDGE('',*,*,#23412,.T.);
#34788=ORIENTED_EDGE('',*,*,#23415,.T.);
#34789=ORIENTED_EDGE('',*,*,#23407,.T.);
#34790=ORIENTED_EDGE('',*,*,#23405,.T.);
#34791=ORIENTED_EDGE('',*,*,#23401,.T.);
#34792=ORIENTED_EDGE('',*,*,#23404,.T.);
#34793=ORIENTED_EDGE('',*,*,#23396,.T.);
#34794=ORIENTED_EDGE('',*,*,#23392,.T.);
#34795=ORIENTED_EDGE('',*,*,#23195,.T.);
#34796=ORIENTED_EDGE('',*,*,#23199,.T.);
#37778=CYLINDRICAL_SURFACE('',#43851,12.);
#39632=ADVANCED_FACE('',(#3829),#1443,.F.);
#39633=ADVANCED_FACE('',(#3830),#1444,.T.);
#39634=ADVANCED_FACE('',(#3831),#1445,.F.);
#39635=ADVANCED_FACE('',(#3832),#1446,.F.);
#39636=ADVANCED_FACE('',(#3833),#37778,.T.);
#39637=ADVANCED_FACE('',(#3834),#693,.T.);
#39638=ADVANCED_FACE('',(#3835),#694,.T.);
#39639=ADVANCED_FACE('',(#3836),#1447,.F.);
#39640=ADVANCED_FACE('',(#3837),#1448,.T.);
#39641=ADVANCED_FACE('',(#3838),#1449,.F.);
#39642=ADVANCED_FACE('',(#3839),#1450,.F.);
#39643=ADVANCED_FACE('',(#3840),#695,.T.);
#39644=ADVANCED_FACE('',(#3841),#1451,.F.);
#39645=ADVANCED_FACE('',(#3842),#1452,.T.);
#39646=ADVANCED_FACE('',(#3843),#1453,.F.);
#39647=ADVANCED_FACE('',(#3844),#1454,.F.);
#39648=ADVANCED_FACE('',(#3845),#696,.T.);
#39649=ADVANCED_FACE('',(#3846),#1455,.F.);
#39650=ADVANCED_FACE('',(#3847),#1456,.T.);
#39651=ADVANCED_FACE('',(#3848),#1457,.F.);
#39652=ADVANCED_FACE('',(#3849),#1458,.F.);
#39653=ADVANCED_FACE('',(#3850),#697,.T.);
#39654=ADVANCED_FACE('',(#3851),#1459,.F.);
#39655=ADVANCED_FACE('',(#3852),#1460,.T.);
#39656=ADVANCED_FACE('',(#3853),#1461,.F.);
#39657=ADVANCED_FACE('',(#3854),#1462,.F.);
#39658=ADVANCED_FACE('',(#3855),#698,.T.);
#39659=ADVANCED_FACE('',(#3856),#1463,.F.);
#39660=ADVANCED_FACE('',(#3857),#1464,.T.);
#39661=ADVANCED_FACE('',(#3858),#1465,.F.);
#39662=ADVANCED_FACE('',(#3859),#1466,.F.);
#39663=ADVANCED_FACE('',(#3860),#699,.T.);
#39664=ADVANCED_FACE('',(#3861),#1467,.F.);
#39665=ADVANCED_FACE('',(#3862),#1468,.T.);
#39666=ADVANCED_FACE('',(#3863),#1469,.F.);
#39667=ADVANCED_FACE('',(#3864),#1470,.F.);
#39668=ADVANCED_FACE('',(#3865),#700,.T.);
#39669=ADVANCED_FACE('',(#3866),#1471,.F.);
#39670=ADVANCED_FACE('',(#3867),#1472,.T.);
#39671=ADVANCED_FACE('',(#3868),#1473,.F.);
#39672=ADVANCED_FACE('',(#3869),#1474,.F.);
#39673=ADVANCED_FACE('',(#3870),#701,.T.);
#39674=ADVANCED_FACE('',(#3871),#1475,.F.);
#39675=ADVANCED_FACE('',(#3872),#1476,.T.);
#39676=ADVANCED_FACE('',(#3873),#1477,.F.);
#39677=ADVANCED_FACE('',(#3874),#1478,.F.);
#39678=ADVANCED_FACE('',(#3875),#702,.T.);
#39679=ADVANCED_FACE('',(#3876),#1479,.F.);
#39680=ADVANCED_FACE('',(#3877),#1480,.T.);
#39681=ADVANCED_FACE('',(#3878),#1481,.F.);
#39682=ADVANCED_FACE('',(#3879),#1482,.F.);
#39683=ADVANCED_FACE('',(#3880),#703,.T.);
#39684=ADVANCED_FACE('',(#3881),#1483,.F.);
#39685=ADVANCED_FACE('',(#3882),#1484,.T.);
#39686=ADVANCED_FACE('',(#3883),#1485,.F.);
#39687=ADVANCED_FACE('',(#3884),#1486,.F.);
#39688=ADVANCED_FACE('',(#3885),#704,.T.);
#39689=ADVANCED_FACE('',(#3886),#1487,.F.);
#39690=ADVANCED_FACE('',(#3887),#1488,.T.);
#39691=ADVANCED_FACE('',(#3888),#1489,.F.);
#39692=ADVANCED_FACE('',(#3889),#1490,.F.);
#39693=ADVANCED_FACE('',(#3890),#705,.T.);
#39694=ADVANCED_FACE('',(#3891),#1491,.F.);
#39695=ADVANCED_FACE('',(#3892),#1492,.T.);
#39696=ADVANCED_FACE('',(#3893),#1493,.F.);
#39697=ADVANCED_FACE('',(#3894),#1494,.F.);
#39698=ADVANCED_FACE('',(#3895),#706,.T.);
#39699=ADVANCED_FACE('',(#3896),#1495,.F.);
#39700=ADVANCED_FACE('',(#3897),#1496,.T.);
#39701=ADVANCED_FACE('',(#3898),#1497,.F.);
#39702=ADVANCED_FACE('',(#3899),#1498,.F.);
#39703=ADVANCED_FACE('',(#3900),#707,.T.);
#39704=ADVANCED_FACE('',(#3901),#1499,.F.);
#39705=ADVANCED_FACE('',(#3902),#1500,.T.);
#39706=ADVANCED_FACE('',(#3903),#1501,.F.);
#39707=ADVANCED_FACE('',(#3904),#1502,.F.);
#39708=ADVANCED_FACE('',(#3905),#708,.T.);
#39709=ADVANCED_FACE('',(#3906),#1503,.F.);
#39710=ADVANCED_FACE('',(#3907),#1504,.T.);
#39711=ADVANCED_FACE('',(#3908),#1505,.F.);
#39712=ADVANCED_FACE('',(#3909),#1506,.F.);
#39713=ADVANCED_FACE('',(#3910),#709,.T.);
#39714=ADVANCED_FACE('',(#3911),#1507,.F.);
#39715=ADVANCED_FACE('',(#3912),#1508,.T.);
#39716=ADVANCED_FACE('',(#3913),#1509,.F.);
#39717=ADVANCED_FACE('',(#3914),#1510,.F.);
#39718=ADVANCED_FACE('',(#3915),#710,.T.);
#39719=ADVANCED_FACE('',(#3916),#1511,.F.);
#39720=ADVANCED_FACE('',(#3917),#1512,.T.);
#39721=ADVANCED_FACE('',(#3918),#1513,.F.);
#39722=ADVANCED_FACE('',(#3919),#1514,.F.);
#39723=ADVANCED_FACE('',(#3920),#711,.T.);
#39724=ADVANCED_FACE('',(#3921),#1515,.F.);
#39725=ADVANCED_FACE('',(#3922),#1516,.T.);
#39726=ADVANCED_FACE('',(#3923),#1517,.F.);
#39727=ADVANCED_FACE('',(#3924),#1518,.F.);
#39728=ADVANCED_FACE('',(#3925),#712,.T.);
#39729=ADVANCED_FACE('',(#3926),#1519,.F.);
#39730=ADVANCED_FACE('',(#3927),#1520,.T.);
#39731=ADVANCED_FACE('',(#3928),#1521,.F.);
#39732=ADVANCED_FACE('',(#3929),#1522,.F.);
#39733=ADVANCED_FACE('',(#3930),#713,.T.);
#39734=ADVANCED_FACE('',(#3931),#1523,.F.);
#39735=ADVANCED_FACE('',(#3932),#1524,.T.);
#39736=ADVANCED_FACE('',(#3933),#1525,.F.);
#39737=ADVANCED_FACE('',(#3934),#1526,.F.);
#39738=ADVANCED_FACE('',(#3935),#714,.T.);
#39739=ADVANCED_FACE('',(#3936),#1527,.F.);
#39740=ADVANCED_FACE('',(#3937),#1528,.T.);
#39741=ADVANCED_FACE('',(#3938),#1529,.F.);
#39742=ADVANCED_FACE('',(#3939),#1530,.F.);
#39743=ADVANCED_FACE('',(#3940),#715,.T.);
#39744=ADVANCED_FACE('',(#3941),#1531,.F.);
#39745=ADVANCED_FACE('',(#3942),#1532,.T.);
#39746=ADVANCED_FACE('',(#3943),#1533,.F.);
#39747=ADVANCED_FACE('',(#3944),#1534,.F.);
#39748=ADVANCED_FACE('',(#3945),#716,.T.);
#39749=ADVANCED_FACE('',(#3946),#1535,.F.);
#39750=ADVANCED_FACE('',(#3947),#1536,.T.);
#39751=ADVANCED_FACE('',(#3948),#1537,.F.);
#39752=ADVANCED_FACE('',(#3949),#1538,.F.);
#39753=ADVANCED_FACE('',(#3950),#1539,.F.);
#39754=ADVANCED_FACE('',(#3951),#1540,.F.);
#39755=ADVANCED_FACE('',(#3952),#1541,.F.);
#39756=ADVANCED_FACE('',(#3953),#1542,.F.);
#39757=ADVANCED_FACE('',(#3954),#1543,.T.);
#39758=ADVANCED_FACE('',(#3955),#717,.T.);
#39759=ADVANCED_FACE('',(#3956),#718,.T.);
#39760=ADVANCED_FACE('',(#3957),#1544,.F.);
#39761=ADVANCED_FACE('',(#3958),#1545,.F.);
#39762=ADVANCED_FACE('',(#3959),#1546,.F.);
#39763=ADVANCED_FACE('',(#3960),#1547,.F.);
#39764=ADVANCED_FACE('',(#3961),#719,.T.);
#39765=ADVANCED_FACE('',(#3962),#1548,.F.);
#39766=ADVANCED_FACE('',(#3963),#1549,.F.);
#39767=ADVANCED_FACE('',(#3964),#1550,.F.);
#39768=ADVANCED_FACE('',(#3965),#1551,.F.);
#39769=ADVANCED_FACE('',(#3966),#720,.T.);
#39770=ADVANCED_FACE('',(#3967),#1552,.F.);
#39771=ADVANCED_FACE('',(#3968),#1553,.F.);
#39772=ADVANCED_FACE('',(#3969),#1554,.F.);
#39773=ADVANCED_FACE('',(#3970),#1555,.F.);
#39774=ADVANCED_FACE('',(#3971),#721,.T.);
#39775=ADVANCED_FACE('',(#3972),#1556,.F.);
#39776=ADVANCED_FACE('',(#3973),#1557,.F.);
#39777=ADVANCED_FACE('',(#3974),#1558,.F.);
#39778=ADVANCED_FACE('',(#3975),#1559,.F.);
#39779=ADVANCED_FACE('',(#3976),#722,.T.);
#39780=ADVANCED_FACE('',(#3977),#1560,.F.);
#39781=ADVANCED_FACE('',(#3978),#1561,.F.);
#39782=ADVANCED_FACE('',(#3979),#1562,.F.);
#39783=ADVANCED_FACE('',(#3980),#1563,.F.);
#39784=ADVANCED_FACE('',(#3981),#723,.T.);
#39785=ADVANCED_FACE('',(#3982),#1564,.F.);
#39786=ADVANCED_FACE('',(#3983),#1565,.F.);
#39787=ADVANCED_FACE('',(#3984),#1566,.F.);
#39788=ADVANCED_FACE('',(#3985),#1567,.F.);
#39789=ADVANCED_FACE('',(#3986),#724,.T.);
#39790=ADVANCED_FACE('',(#3987),#1568,.F.);
#39791=ADVANCED_FACE('',(#3988),#1569,.F.);
#39792=ADVANCED_FACE('',(#3989),#1570,.F.);
#39793=ADVANCED_FACE('',(#3990),#1571,.F.);
#39794=ADVANCED_FACE('',(#3991),#725,.T.);
#39795=ADVANCED_FACE('',(#3992),#1572,.F.);
#39796=ADVANCED_FACE('',(#3993),#1573,.F.);
#39797=ADVANCED_FACE('',(#3994),#1574,.F.);
#39798=ADVANCED_FACE('',(#3995),#1575,.F.);
#39799=ADVANCED_FACE('',(#3996),#726,.T.);
#39800=ADVANCED_FACE('',(#3997),#1576,.F.);
#39801=ADVANCED_FACE('',(#3998),#1577,.F.);
#39802=ADVANCED_FACE('',(#3999),#1578,.F.);
#39803=ADVANCED_FACE('',(#4000),#1579,.F.);
#39804=ADVANCED_FACE('',(#4001),#727,.T.);
#39805=ADVANCED_FACE('',(#4002),#1580,.F.);
#39806=ADVANCED_FACE('',(#4003),#1581,.F.);
#39807=ADVANCED_FACE('',(#4004),#1582,.F.);
#39808=ADVANCED_FACE('',(#4005),#1583,.F.);
#39809=ADVANCED_FACE('',(#4006),#728,.T.);
#39810=ADVANCED_FACE('',(#4007),#1584,.F.);
#39811=ADVANCED_FACE('',(#4008),#1585,.F.);
#39812=ADVANCED_FACE('',(#4009),#1586,.F.);
#39813=ADVANCED_FACE('',(#4010),#1587,.F.);
#39814=ADVANCED_FACE('',(#4011),#729,.T.);
#39815=ADVANCED_FACE('',(#4012),#1588,.F.);
#39816=ADVANCED_FACE('',(#4013),#1589,.F.);
#39817=ADVANCED_FACE('',(#4014),#1590,.F.);
#39818=ADVANCED_FACE('',(#4015),#1591,.F.);
#39819=ADVANCED_FACE('',(#4016),#730,.T.);
#39820=ADVANCED_FACE('',(#4017),#1592,.F.);
#39821=ADVANCED_FACE('',(#4018),#1593,.F.);
#39822=ADVANCED_FACE('',(#4019),#1594,.F.);
#39823=ADVANCED_FACE('',(#4020),#1595,.F.);
#39824=ADVANCED_FACE('',(#4021),#731,.T.);
#39825=ADVANCED_FACE('',(#4022),#1596,.F.);
#39826=ADVANCED_FACE('',(#4023),#1597,.F.);
#39827=ADVANCED_FACE('',(#4024),#1598,.F.);
#39828=ADVANCED_FACE('',(#4025),#1599,.F.);
#39829=ADVANCED_FACE('',(#4026),#732,.T.);
#39830=ADVANCED_FACE('',(#4027),#1600,.F.);
#39831=ADVANCED_FACE('',(#4028),#1601,.F.);
#39832=ADVANCED_FACE('',(#4029),#1602,.F.);
#39833=ADVANCED_FACE('',(#4030),#1603,.F.);
#39834=ADVANCED_FACE('',(#4031),#733,.T.);
#39835=ADVANCED_FACE('',(#4032),#1604,.F.);
#39836=ADVANCED_FACE('',(#4033),#1605,.F.);
#39837=ADVANCED_FACE('',(#4034),#1606,.F.);
#39838=ADVANCED_FACE('',(#4035),#1607,.F.);
#39839=ADVANCED_FACE('',(#4036),#734,.T.);
#39840=ADVANCED_FACE('',(#4037),#1608,.F.);
#39841=ADVANCED_FACE('',(#4038),#1609,.F.);
#39842=ADVANCED_FACE('',(#4039),#1610,.F.);
#39843=ADVANCED_FACE('',(#4040),#1611,.F.);
#39844=ADVANCED_FACE('',(#4041),#735,.T.);
#39845=ADVANCED_FACE('',(#4042),#1612,.F.);
#39846=ADVANCED_FACE('',(#4043),#1613,.F.);
#39847=ADVANCED_FACE('',(#4044),#1614,.F.);
#39848=ADVANCED_FACE('',(#4045),#1615,.F.);
#39849=ADVANCED_FACE('',(#4046),#736,.T.);
#39850=ADVANCED_FACE('',(#4047),#1616,.F.);
#39851=ADVANCED_FACE('',(#4048),#1617,.F.);
#39852=ADVANCED_FACE('',(#4049),#1618,.F.);
#39853=ADVANCED_FACE('',(#4050),#1619,.F.);
#39854=ADVANCED_FACE('',(#4051),#737,.T.);
#39855=ADVANCED_FACE('',(#4052),#1620,.F.);
#39856=ADVANCED_FACE('',(#4053),#1621,.F.);
#39857=ADVANCED_FACE('',(#4054),#1622,.F.);
#39858=ADVANCED_FACE('',(#4055),#1623,.F.);
#39859=ADVANCED_FACE('',(#4056),#738,.T.);
#39860=ADVANCED_FACE('',(#4057),#1624,.F.);
#39861=ADVANCED_FACE('',(#4058),#1625,.F.);
#39862=ADVANCED_FACE('',(#4059),#1626,.F.);
#39863=ADVANCED_FACE('',(#4060),#1627,.F.);
#39864=ADVANCED_FACE('',(#4061),#739,.T.);
#39865=ADVANCED_FACE('',(#4062),#1628,.F.);
#39866=ADVANCED_FACE('',(#4063),#1629,.F.);
#39867=ADVANCED_FACE('',(#4064),#1630,.F.);
#39868=ADVANCED_FACE('',(#4065),#1631,.F.);
#39869=ADVANCED_FACE('',(#4066),#740,.T.);
#39870=ADVANCED_FACE('',(#4067),#1632,.F.);
#39871=ADVANCED_FACE('',(#4068),#1633,.F.);
#39872=ADVANCED_FACE('',(#4069),#1634,.F.);
#39873=ADVANCED_FACE('',(#4070),#1635,.F.);
#39874=ADVANCED_FACE('',(#4071),#1636,.T.);
#40354=CLOSED_SHELL('',(#39632,#39633,#39634,#39635,#39636,#39637,#39638,
#39639,#39640,#39641,#39642,#39643,#39644,#39645,#39646,#39647,#39648,#39649,
#39650,#39651,#39652,#39653,#39654,#39655,#39656,#39657,#39658,#39659,#39660,
#39661,#39662,#39663,#39664,#39665,#39666,#39667,#39668,#39669,#39670,#39671,
#39672,#39673,#39674,#39675,#39676,#39677,#39678,#39679,#39680,#39681,#39682,
#39683,#39684,#39685,#39686,#39687,#39688,#39689,#39690,#39691,#39692,#39693,
#39694,#39695,#39696,#39697,#39698,#39699,#39700,#39701,#39702,#39703,#39704,
#39705,#39706,#39707,#39708,#39709,#39710,#39711,#39712,#39713,#39714,#39715,
#39716,#39717,#39718,#39719,#39720,#39721,#39722,#39723,#39724,#39725,#39726,
#39727,#39728,#39729,#39730,#39731,#39732,#39733,#39734,#39735,#39736,#39737,
#39738,#39739,#39740,#39741,#39742,#39743,#39744,#39745,#39746,#39747,#39748,
#39749,#39750,#39751,#39752,#39753,#39754,#39755,#39756,#39757,#39758,#39759,
#39760,#39761,#39762,#39763,#39764,#39765,#39766,#39767,#39768,#39769,#39770,
#39771,#39772,#39773,#39774,#39775,#39776,#39777,#39778,#39779,#39780,#39781,
#39782,#39783,#39784,#39785,#39786,#39787,#39788,#39789,#39790,#39791,#39792,
#39793,#39794,#39795,#39796,#39797,#39798,#39799,#39800,#39801,#39802,#39803,
#39804,#39805,#39806,#39807,#39808,#39809,#39810,#39811,#39812,#39813,#39814,
#39815,#39816,#39817,#39818,#39819,#39820,#39821,#39822,#39823,#39824,#39825,
#39826,#39827,#39828,#39829,#39830,#39831,#39832,#39833,#39834,#39835,#39836,
#39837,#39838,#39839,#39840,#39841,#39842,#39843,#39844,#39845,#39846,#39847,
#39848,#39849,#39850,#39851,#39852,#39853,#39854,#39855,#39856,#39857,#39858,
#39859,#39860,#39861,#39862,#39863,#39864,#39865,#39866,#39867,#39868,#39869,
#39870,#39871,#39872,#39873,#39874));
#43845=AXIS2_PLACEMENT_3D('',#83021,#53383,#53384);
#43846=AXIS2_PLACEMENT_3D('',#83022,#53385,#53386);
#43847=AXIS2_PLACEMENT_3D('',#83035,#53391,#53392);
#43848=AXIS2_PLACEMENT_3D('',#83037,#53393,#53394);
#43849=AXIS2_PLACEMENT_3D('',#83041,#53397,#53398);
#43850=AXIS2_PLACEMENT_3D('',#83051,#53402,#53403);
#43851=AXIS2_PLACEMENT_3D('',#83053,#53405,#53406);
#43852=AXIS2_PLACEMENT_3D('',#83055,#53407,#53408);
#43853=AXIS2_PLACEMENT_3D('',#83059,#53410,#53411);
#43854=AXIS2_PLACEMENT_3D('',#83063,#53413,#53414);
#43855=AXIS2_PLACEMENT_3D('',#83067,#53416,#53417);
#43856=AXIS2_PLACEMENT_3D('',#83071,#53419,#53420);
#43857=AXIS2_PLACEMENT_3D('',#83075,#53422,#53423);
#43858=AXIS2_PLACEMENT_3D('',#83079,#53425,#53426);
#43859=AXIS2_PLACEMENT_3D('',#83083,#53428,#53429);
#43860=AXIS2_PLACEMENT_3D('',#83087,#53431,#53432);
#43861=AXIS2_PLACEMENT_3D('',#83091,#53434,#53435);
#43862=AXIS2_PLACEMENT_3D('',#83095,#53437,#53438);
#43863=AXIS2_PLACEMENT_3D('',#83099,#53440,#53441);
#43864=AXIS2_PLACEMENT_3D('',#83103,#53443,#53444);
#43865=AXIS2_PLACEMENT_3D('',#83107,#53446,#53447);
#43866=AXIS2_PLACEMENT_3D('',#83111,#53449,#53450);
#43867=AXIS2_PLACEMENT_3D('',#83115,#53452,#53453);
#43868=AXIS2_PLACEMENT_3D('',#83119,#53455,#53456);
#43869=AXIS2_PLACEMENT_3D('',#83123,#53458,#53459);
#43870=AXIS2_PLACEMENT_3D('',#83127,#53461,#53462);
#43871=AXIS2_PLACEMENT_3D('',#83131,#53464,#53465);
#43872=AXIS2_PLACEMENT_3D('',#83135,#53467,#53468);
#43873=AXIS2_PLACEMENT_3D('',#83139,#53470,#53471);
#43874=AXIS2_PLACEMENT_3D('',#83143,#53473,#53474);
#43875=AXIS2_PLACEMENT_3D('',#83147,#53476,#53477);
#43876=AXIS2_PLACEMENT_3D('',#83151,#53479,#53480);
#43877=AXIS2_PLACEMENT_3D('',#83155,#53482,#53483);
#43878=AXIS2_PLACEMENT_3D('',#83159,#53485,#53486);
#43879=AXIS2_PLACEMENT_3D('',#83163,#53488,#53489);
#43880=AXIS2_PLACEMENT_3D('',#83167,#53491,#53492);
#43881=AXIS2_PLACEMENT_3D('',#83171,#53494,#53495);
#43882=AXIS2_PLACEMENT_3D('',#83175,#53497,#53498);
#43883=AXIS2_PLACEMENT_3D('',#83179,#53500,#53501);
#43884=AXIS2_PLACEMENT_3D('',#83183,#53503,#53504);
#43885=AXIS2_PLACEMENT_3D('',#83187,#53506,#53507);
#43886=AXIS2_PLACEMENT_3D('',#83191,#53509,#53510);
#43887=AXIS2_PLACEMENT_3D('',#83195,#53512,#53513);
#43888=AXIS2_PLACEMENT_3D('',#83199,#53515,#53516);
#43889=AXIS2_PLACEMENT_3D('',#83203,#53518,#53519);
#43890=AXIS2_PLACEMENT_3D('',#83207,#53521,#53522);
#43891=AXIS2_PLACEMENT_3D('',#83211,#53524,#53525);
#43892=AXIS2_PLACEMENT_3D('',#83215,#53527,#53528);
#43893=AXIS2_PLACEMENT_3D('',#83219,#53530,#53531);
#43894=AXIS2_PLACEMENT_3D('',#83223,#53533,#53534);
#43895=AXIS2_PLACEMENT_3D('',#83227,#53536,#53537);
#43896=AXIS2_PLACEMENT_3D('',#83231,#53539,#53540);
#43897=AXIS2_PLACEMENT_3D('',#83235,#53542,#53543);
#43898=AXIS2_PLACEMENT_3D('',#83239,#53545,#53546);
#43899=AXIS2_PLACEMENT_3D('',#83243,#53548,#53549);
#43900=AXIS2_PLACEMENT_3D('',#83247,#53551,#53552);
#43901=AXIS2_PLACEMENT_3D('',#83251,#53554,#53555);
#43902=AXIS2_PLACEMENT_3D('',#83255,#53557,#53558);
#43903=AXIS2_PLACEMENT_3D('',#83259,#53560,#53561);
#43904=AXIS2_PLACEMENT_3D('',#83263,#53563,#53564);
#43905=AXIS2_PLACEMENT_3D('',#83267,#53566,#53567);
#43906=AXIS2_PLACEMENT_3D('',#83271,#53569,#53570);
#43907=AXIS2_PLACEMENT_3D('',#83275,#53572,#53573);
#43908=AXIS2_PLACEMENT_3D('',#83279,#53575,#53576);
#43909=AXIS2_PLACEMENT_3D('',#83283,#53578,#53579);
#43910=AXIS2_PLACEMENT_3D('',#83287,#53581,#53582);
#43911=AXIS2_PLACEMENT_3D('',#83291,#53584,#53585);
#43912=AXIS2_PLACEMENT_3D('',#83295,#53587,#53588);
#43913=AXIS2_PLACEMENT_3D('',#83299,#53590,#53591);
#43914=AXIS2_PLACEMENT_3D('',#83303,#53593,#53594);
#43915=AXIS2_PLACEMENT_3D('',#83307,#53596,#53597);
#43916=AXIS2_PLACEMENT_3D('',#83311,#53599,#53600);
#43917=AXIS2_PLACEMENT_3D('',#83315,#53602,#53603);
#43918=AXIS2_PLACEMENT_3D('',#83319,#53605,#53606);
#43919=AXIS2_PLACEMENT_3D('',#83323,#53608,#53609);
#43920=AXIS2_PLACEMENT_3D('',#83327,#53611,#53612);
#43921=AXIS2_PLACEMENT_3D('',#83331,#53614,#53615);
#43922=AXIS2_PLACEMENT_3D('',#83334,#53617,#53618);
#43923=AXIS2_PLACEMENT_3D('',#83336,#53619,#53620);
#43924=AXIS2_PLACEMENT_3D('',#83340,#53622,#53623);
#43925=AXIS2_PLACEMENT_3D('',#83344,#53625,#53626);
#43926=AXIS2_PLACEMENT_3D('',#83348,#53628,#53629);
#43927=AXIS2_PLACEMENT_3D('',#83352,#53631,#53632);
#43928=AXIS2_PLACEMENT_3D('',#83356,#53634,#53635);
#43929=AXIS2_PLACEMENT_3D('',#83360,#53637,#53638);
#43930=AXIS2_PLACEMENT_3D('',#83364,#53640,#53641);
#43931=AXIS2_PLACEMENT_3D('',#83368,#53643,#53644);
#43932=AXIS2_PLACEMENT_3D('',#83372,#53646,#53647);
#43933=AXIS2_PLACEMENT_3D('',#83376,#53649,#53650);
#43934=AXIS2_PLACEMENT_3D('',#83380,#53652,#53653);
#43935=AXIS2_PLACEMENT_3D('',#83384,#53655,#53656);
#43936=AXIS2_PLACEMENT_3D('',#83388,#53658,#53659);
#43937=AXIS2_PLACEMENT_3D('',#83392,#53661,#53662);
#43938=AXIS2_PLACEMENT_3D('',#83396,#53664,#53665);
#43939=AXIS2_PLACEMENT_3D('',#83400,#53667,#53668);
#43940=AXIS2_PLACEMENT_3D('',#83404,#53670,#53671);
#43941=AXIS2_PLACEMENT_3D('',#83408,#53673,#53674);
#43942=AXIS2_PLACEMENT_3D('',#83412,#53676,#53677);
#43943=AXIS2_PLACEMENT_3D('',#83416,#53679,#53680);
#43944=AXIS2_PLACEMENT_3D('',#83420,#53682,#53683);
#43945=AXIS2_PLACEMENT_3D('',#83424,#53685,#53686);
#43946=AXIS2_PLACEMENT_3D('',#83428,#53688,#53689);
#43947=AXIS2_PLACEMENT_3D('',#83432,#53691,#53692);
#43948=AXIS2_PLACEMENT_3D('',#83435,#53694,#53695);
#43949=AXIS2_PLACEMENT_3D('',#83436,#53696,#53697);
#43950=AXIS2_PLACEMENT_3D('',#83438,#53698,#53699);
#43951=AXIS2_PLACEMENT_3D('',#83442,#53700,#53701);
#43952=AXIS2_PLACEMENT_3D('',#83447,#53702,#53703);
#43953=AXIS2_PLACEMENT_3D('',#83448,#53704,#53705);
#43954=AXIS2_PLACEMENT_3D('',#83454,#53709,#53710);
#43955=AXIS2_PLACEMENT_3D('',#83458,#53713,#53714);
#43956=AXIS2_PLACEMENT_3D('',#83466,#53717,#53718);
#43957=AXIS2_PLACEMENT_3D('',#83468,#53720,#53721);
#43958=AXIS2_PLACEMENT_3D('',#83470,#53722,#53723);
#43959=AXIS2_PLACEMENT_3D('',#83474,#53724,#53725);
#43960=AXIS2_PLACEMENT_3D('',#83480,#53729,#53730);
#43961=AXIS2_PLACEMENT_3D('',#83484,#53733,#53734);
#43962=AXIS2_PLACEMENT_3D('',#83492,#53737,#53738);
#43963=AXIS2_PLACEMENT_3D('',#83494,#53740,#53741);
#43964=AXIS2_PLACEMENT_3D('',#83496,#53742,#53743);
#43965=AXIS2_PLACEMENT_3D('',#83500,#53744,#53745);
#43966=AXIS2_PLACEMENT_3D('',#83506,#53749,#53750);
#43967=AXIS2_PLACEMENT_3D('',#83510,#53753,#53754);
#43968=AXIS2_PLACEMENT_3D('',#83518,#53757,#53758);
#43969=AXIS2_PLACEMENT_3D('',#83520,#53760,#53761);
#43970=AXIS2_PLACEMENT_3D('',#83522,#53762,#53763);
#43971=AXIS2_PLACEMENT_3D('',#83526,#53764,#53765);
#43972=AXIS2_PLACEMENT_3D('',#83532,#53769,#53770);
#43973=AXIS2_PLACEMENT_3D('',#83536,#53773,#53774);
#43974=AXIS2_PLACEMENT_3D('',#83544,#53777,#53778);
#43975=AXIS2_PLACEMENT_3D('',#83546,#53780,#53781);
#43976=AXIS2_PLACEMENT_3D('',#83548,#53782,#53783);
#43977=AXIS2_PLACEMENT_3D('',#83552,#53784,#53785);
#43978=AXIS2_PLACEMENT_3D('',#83558,#53789,#53790);
#43979=AXIS2_PLACEMENT_3D('',#83562,#53793,#53794);
#43980=AXIS2_PLACEMENT_3D('',#83570,#53797,#53798);
#43981=AXIS2_PLACEMENT_3D('',#83572,#53800,#53801);
#43982=AXIS2_PLACEMENT_3D('',#83574,#53802,#53803);
#43983=AXIS2_PLACEMENT_3D('',#83578,#53804,#53805);
#43984=AXIS2_PLACEMENT_3D('',#83584,#53809,#53810);
#43985=AXIS2_PLACEMENT_3D('',#83588,#53813,#53814);
#43986=AXIS2_PLACEMENT_3D('',#83596,#53817,#53818);
#43987=AXIS2_PLACEMENT_3D('',#83598,#53820,#53821);
#43988=AXIS2_PLACEMENT_3D('',#83600,#53822,#53823);
#43989=AXIS2_PLACEMENT_3D('',#83604,#53824,#53825);
#43990=AXIS2_PLACEMENT_3D('',#83610,#53829,#53830);
#43991=AXIS2_PLACEMENT_3D('',#83614,#53833,#53834);
#43992=AXIS2_PLACEMENT_3D('',#83622,#53837,#53838);
#43993=AXIS2_PLACEMENT_3D('',#83624,#53840,#53841);
#43994=AXIS2_PLACEMENT_3D('',#83626,#53842,#53843);
#43995=AXIS2_PLACEMENT_3D('',#83630,#53844,#53845);
#43996=AXIS2_PLACEMENT_3D('',#83636,#53849,#53850);
#43997=AXIS2_PLACEMENT_3D('',#83640,#53853,#53854);
#43998=AXIS2_PLACEMENT_3D('',#83648,#53857,#53858);
#43999=AXIS2_PLACEMENT_3D('',#83650,#53860,#53861);
#44000=AXIS2_PLACEMENT_3D('',#83652,#53862,#53863);
#44001=AXIS2_PLACEMENT_3D('',#83656,#53864,#53865);
#44002=AXIS2_PLACEMENT_3D('',#83662,#53869,#53870);
#44003=AXIS2_PLACEMENT_3D('',#83666,#53873,#53874);
#44004=AXIS2_PLACEMENT_3D('',#83674,#53877,#53878);
#44005=AXIS2_PLACEMENT_3D('',#83676,#53880,#53881);
#44006=AXIS2_PLACEMENT_3D('',#83678,#53882,#53883);
#44007=AXIS2_PLACEMENT_3D('',#83682,#53884,#53885);
#44008=AXIS2_PLACEMENT_3D('',#83688,#53889,#53890);
#44009=AXIS2_PLACEMENT_3D('',#83692,#53893,#53894);
#44010=AXIS2_PLACEMENT_3D('',#83700,#53897,#53898);
#44011=AXIS2_PLACEMENT_3D('',#83702,#53900,#53901);
#44012=AXIS2_PLACEMENT_3D('',#83704,#53902,#53903);
#44013=AXIS2_PLACEMENT_3D('',#83708,#53904,#53905);
#44014=AXIS2_PLACEMENT_3D('',#83714,#53909,#53910);
#44015=AXIS2_PLACEMENT_3D('',#83718,#53913,#53914);
#44016=AXIS2_PLACEMENT_3D('',#83726,#53917,#53918);
#44017=AXIS2_PLACEMENT_3D('',#83728,#53920,#53921);
#44018=AXIS2_PLACEMENT_3D('',#83730,#53922,#53923);
#44019=AXIS2_PLACEMENT_3D('',#83734,#53924,#53925);
#44020=AXIS2_PLACEMENT_3D('',#83740,#53929,#53930);
#44021=AXIS2_PLACEMENT_3D('',#83744,#53933,#53934);
#44022=AXIS2_PLACEMENT_3D('',#83752,#53937,#53938);
#44023=AXIS2_PLACEMENT_3D('',#83754,#53940,#53941);
#44024=AXIS2_PLACEMENT_3D('',#83756,#53942,#53943);
#44025=AXIS2_PLACEMENT_3D('',#83760,#53944,#53945);
#44026=AXIS2_PLACEMENT_3D('',#83766,#53949,#53950);
#44027=AXIS2_PLACEMENT_3D('',#83770,#53953,#53954);
#44028=AXIS2_PLACEMENT_3D('',#83778,#53957,#53958);
#44029=AXIS2_PLACEMENT_3D('',#83780,#53960,#53961);
#44030=AXIS2_PLACEMENT_3D('',#83782,#53962,#53963);
#44031=AXIS2_PLACEMENT_3D('',#83786,#53964,#53965);
#44032=AXIS2_PLACEMENT_3D('',#83792,#53969,#53970);
#44033=AXIS2_PLACEMENT_3D('',#83796,#53973,#53974);
#44034=AXIS2_PLACEMENT_3D('',#83804,#53977,#53978);
#44035=AXIS2_PLACEMENT_3D('',#83806,#53980,#53981);
#44036=AXIS2_PLACEMENT_3D('',#83808,#53982,#53983);
#44037=AXIS2_PLACEMENT_3D('',#83812,#53984,#53985);
#44038=AXIS2_PLACEMENT_3D('',#83818,#53989,#53990);
#44039=AXIS2_PLACEMENT_3D('',#83822,#53993,#53994);
#44040=AXIS2_PLACEMENT_3D('',#83830,#53997,#53998);
#44041=AXIS2_PLACEMENT_3D('',#83832,#54000,#54001);
#44042=AXIS2_PLACEMENT_3D('',#83834,#54002,#54003);
#44043=AXIS2_PLACEMENT_3D('',#83838,#54004,#54005);
#44044=AXIS2_PLACEMENT_3D('',#83844,#54009,#54010);
#44045=AXIS2_PLACEMENT_3D('',#83848,#54013,#54014);
#44046=AXIS2_PLACEMENT_3D('',#83856,#54017,#54018);
#44047=AXIS2_PLACEMENT_3D('',#83858,#54020,#54021);
#44048=AXIS2_PLACEMENT_3D('',#83860,#54022,#54023);
#44049=AXIS2_PLACEMENT_3D('',#83864,#54024,#54025);
#44050=AXIS2_PLACEMENT_3D('',#83870,#54029,#54030);
#44051=AXIS2_PLACEMENT_3D('',#83874,#54033,#54034);
#44052=AXIS2_PLACEMENT_3D('',#83882,#54037,#54038);
#44053=AXIS2_PLACEMENT_3D('',#83884,#54040,#54041);
#44054=AXIS2_PLACEMENT_3D('',#83886,#54042,#54043);
#44055=AXIS2_PLACEMENT_3D('',#83890,#54044,#54045);
#44056=AXIS2_PLACEMENT_3D('',#83896,#54049,#54050);
#44057=AXIS2_PLACEMENT_3D('',#83900,#54053,#54054);
#44058=AXIS2_PLACEMENT_3D('',#83908,#54057,#54058);
#44059=AXIS2_PLACEMENT_3D('',#83910,#54060,#54061);
#44060=AXIS2_PLACEMENT_3D('',#83912,#54062,#54063);
#44061=AXIS2_PLACEMENT_3D('',#83916,#54064,#54065);
#44062=AXIS2_PLACEMENT_3D('',#83922,#54069,#54070);
#44063=AXIS2_PLACEMENT_3D('',#83926,#54073,#54074);
#44064=AXIS2_PLACEMENT_3D('',#83934,#54077,#54078);
#44065=AXIS2_PLACEMENT_3D('',#83936,#54080,#54081);
#44066=AXIS2_PLACEMENT_3D('',#83938,#54082,#54083);
#44067=AXIS2_PLACEMENT_3D('',#83942,#54084,#54085);
#44068=AXIS2_PLACEMENT_3D('',#83948,#54089,#54090);
#44069=AXIS2_PLACEMENT_3D('',#83952,#54093,#54094);
#44070=AXIS2_PLACEMENT_3D('',#83960,#54097,#54098);
#44071=AXIS2_PLACEMENT_3D('',#83962,#54100,#54101);
#44072=AXIS2_PLACEMENT_3D('',#83964,#54102,#54103);
#44073=AXIS2_PLACEMENT_3D('',#83968,#54104,#54105);
#44074=AXIS2_PLACEMENT_3D('',#83974,#54109,#54110);
#44075=AXIS2_PLACEMENT_3D('',#83978,#54113,#54114);
#44076=AXIS2_PLACEMENT_3D('',#83986,#54117,#54118);
#44077=AXIS2_PLACEMENT_3D('',#83988,#54120,#54121);
#44078=AXIS2_PLACEMENT_3D('',#83990,#54122,#54123);
#44079=AXIS2_PLACEMENT_3D('',#83994,#54124,#54125);
#44080=AXIS2_PLACEMENT_3D('',#84000,#54129,#54130);
#44081=AXIS2_PLACEMENT_3D('',#84004,#54133,#54134);
#44082=AXIS2_PLACEMENT_3D('',#84012,#54137,#54138);
#44083=AXIS2_PLACEMENT_3D('',#84014,#54140,#54141);
#44084=AXIS2_PLACEMENT_3D('',#84016,#54142,#54143);
#44085=AXIS2_PLACEMENT_3D('',#84020,#54144,#54145);
#44086=AXIS2_PLACEMENT_3D('',#84026,#54149,#54150);
#44087=AXIS2_PLACEMENT_3D('',#84030,#54153,#54154);
#44088=AXIS2_PLACEMENT_3D('',#84034,#54157,#54158);
#44089=AXIS2_PLACEMENT_3D('',#84036,#54160,#54161);
#44090=AXIS2_PLACEMENT_3D('',#84046,#54165,#54166);
#44091=AXIS2_PLACEMENT_3D('',#84052,#54170,#54171);
#44092=AXIS2_PLACEMENT_3D('',#84059,#54174,#54175);
#44093=AXIS2_PLACEMENT_3D('',#84060,#54176,#54177);
#44094=AXIS2_PLACEMENT_3D('',#84062,#54178,#54179);
#44095=AXIS2_PLACEMENT_3D('',#84070,#54183,#54184);
#44096=AXIS2_PLACEMENT_3D('',#84078,#54188,#54189);
#44097=AXIS2_PLACEMENT_3D('',#84086,#54193,#54194);
#44098=AXIS2_PLACEMENT_3D('',#84094,#54198,#54199);
#44099=AXIS2_PLACEMENT_3D('',#84102,#54203,#54204);
#44100=AXIS2_PLACEMENT_3D('',#84110,#54208,#54209);
#44101=AXIS2_PLACEMENT_3D('',#84118,#54213,#54214);
#44102=AXIS2_PLACEMENT_3D('',#84126,#54218,#54219);
#44103=AXIS2_PLACEMENT_3D('',#84134,#54223,#54224);
#44104=AXIS2_PLACEMENT_3D('',#84142,#54228,#54229);
#44105=AXIS2_PLACEMENT_3D('',#84150,#54233,#54234);
#44106=AXIS2_PLACEMENT_3D('',#84158,#54238,#54239);
#44107=AXIS2_PLACEMENT_3D('',#84166,#54243,#54244);
#44108=AXIS2_PLACEMENT_3D('',#84174,#54248,#54249);
#44109=AXIS2_PLACEMENT_3D('',#84182,#54253,#54254);
#44110=AXIS2_PLACEMENT_3D('',#84190,#54258,#54259);
#44111=AXIS2_PLACEMENT_3D('',#84198,#54263,#54264);
#44112=AXIS2_PLACEMENT_3D('',#84206,#54268,#54269);
#44113=AXIS2_PLACEMENT_3D('',#84214,#54273,#54274);
#44114=AXIS2_PLACEMENT_3D('',#84222,#54278,#54279);
#44115=AXIS2_PLACEMENT_3D('',#84230,#54283,#54284);
#44116=AXIS2_PLACEMENT_3D('',#84238,#54288,#54289);
#44117=AXIS2_PLACEMENT_3D('',#84245,#54293,#54294);
#44118=AXIS2_PLACEMENT_3D('',#84246,#54295,#54296);
#44119=AXIS2_PLACEMENT_3D('',#84250,#54297,#54298);
#44120=AXIS2_PLACEMENT_3D('',#84254,#54299,#54300);
#44121=AXIS2_PLACEMENT_3D('',#84258,#54303,#54304);
#44122=AXIS2_PLACEMENT_3D('',#84262,#54307,#54308);
#44123=AXIS2_PLACEMENT_3D('',#84267,#54310,#54311);
#44124=AXIS2_PLACEMENT_3D('',#84268,#54312,#54313);
#44125=AXIS2_PLACEMENT_3D('',#84272,#54314,#54315);
#44126=AXIS2_PLACEMENT_3D('',#84276,#54318,#54319);
#44127=AXIS2_PLACEMENT_3D('',#84280,#54322,#54323);
#44128=AXIS2_PLACEMENT_3D('',#84285,#54325,#54326);
#44129=AXIS2_PLACEMENT_3D('',#84286,#54327,#54328);
#44130=AXIS2_PLACEMENT_3D('',#84290,#54329,#54330);
#44131=AXIS2_PLACEMENT_3D('',#84294,#54333,#54334);
#44132=AXIS2_PLACEMENT_3D('',#84298,#54337,#54338);
#44133=AXIS2_PLACEMENT_3D('',#84303,#54340,#54341);
#44134=AXIS2_PLACEMENT_3D('',#84304,#54342,#54343);
#44135=AXIS2_PLACEMENT_3D('',#84308,#54344,#54345);
#44136=AXIS2_PLACEMENT_3D('',#84312,#54348,#54349);
#44137=AXIS2_PLACEMENT_3D('',#84316,#54352,#54353);
#44138=AXIS2_PLACEMENT_3D('',#84321,#54355,#54356);
#44139=AXIS2_PLACEMENT_3D('',#84322,#54357,#54358);
#44140=AXIS2_PLACEMENT_3D('',#84326,#54359,#54360);
#44141=AXIS2_PLACEMENT_3D('',#84330,#54363,#54364);
#44142=AXIS2_PLACEMENT_3D('',#84334,#54367,#54368);
#44143=AXIS2_PLACEMENT_3D('',#84339,#54370,#54371);
#44144=AXIS2_PLACEMENT_3D('',#84340,#54372,#54373);
#44145=AXIS2_PLACEMENT_3D('',#84344,#54374,#54375);
#44146=AXIS2_PLACEMENT_3D('',#84348,#54378,#54379);
#44147=AXIS2_PLACEMENT_3D('',#84352,#54382,#54383);
#44148=AXIS2_PLACEMENT_3D('',#84357,#54385,#54386);
#44149=AXIS2_PLACEMENT_3D('',#84358,#54387,#54388);
#44150=AXIS2_PLACEMENT_3D('',#84362,#54389,#54390);
#44151=AXIS2_PLACEMENT_3D('',#84366,#54393,#54394);
#44152=AXIS2_PLACEMENT_3D('',#84370,#54397,#54398);
#44153=AXIS2_PLACEMENT_3D('',#84375,#54400,#54401);
#44154=AXIS2_PLACEMENT_3D('',#84376,#54402,#54403);
#44155=AXIS2_PLACEMENT_3D('',#84380,#54404,#54405);
#44156=AXIS2_PLACEMENT_3D('',#84384,#54408,#54409);
#44157=AXIS2_PLACEMENT_3D('',#84388,#54412,#54413);
#44158=AXIS2_PLACEMENT_3D('',#84393,#54415,#54416);
#44159=AXIS2_PLACEMENT_3D('',#84394,#54417,#54418);
#44160=AXIS2_PLACEMENT_3D('',#84398,#54419,#54420);
#44161=AXIS2_PLACEMENT_3D('',#84402,#54423,#54424);
#44162=AXIS2_PLACEMENT_3D('',#84406,#54427,#54428);
#44163=AXIS2_PLACEMENT_3D('',#84411,#54430,#54431);
#44164=AXIS2_PLACEMENT_3D('',#84412,#54432,#54433);
#44165=AXIS2_PLACEMENT_3D('',#84416,#54434,#54435);
#44166=AXIS2_PLACEMENT_3D('',#84420,#54438,#54439);
#44167=AXIS2_PLACEMENT_3D('',#84424,#54442,#54443);
#44168=AXIS2_PLACEMENT_3D('',#84429,#54445,#54446);
#44169=AXIS2_PLACEMENT_3D('',#84430,#54447,#54448);
#44170=AXIS2_PLACEMENT_3D('',#84434,#54449,#54450);
#44171=AXIS2_PLACEMENT_3D('',#84438,#54453,#54454);
#44172=AXIS2_PLACEMENT_3D('',#84442,#54457,#54458);
#44173=AXIS2_PLACEMENT_3D('',#84447,#54460,#54461);
#44174=AXIS2_PLACEMENT_3D('',#84448,#54462,#54463);
#44175=AXIS2_PLACEMENT_3D('',#84452,#54464,#54465);
#44176=AXIS2_PLACEMENT_3D('',#84456,#54468,#54469);
#44177=AXIS2_PLACEMENT_3D('',#84460,#54472,#54473);
#44178=AXIS2_PLACEMENT_3D('',#84465,#54475,#54476);
#44179=AXIS2_PLACEMENT_3D('',#84466,#54477,#54478);
#44180=AXIS2_PLACEMENT_3D('',#84470,#54479,#54480);
#44181=AXIS2_PLACEMENT_3D('',#84474,#54483,#54484);
#44182=AXIS2_PLACEMENT_3D('',#84478,#54487,#54488);
#44183=AXIS2_PLACEMENT_3D('',#84483,#54490,#54491);
#44184=AXIS2_PLACEMENT_3D('',#84484,#54492,#54493);
#44185=AXIS2_PLACEMENT_3D('',#84488,#54494,#54495);
#44186=AXIS2_PLACEMENT_3D('',#84492,#54498,#54499);
#44187=AXIS2_PLACEMENT_3D('',#84496,#54502,#54503);
#44188=AXIS2_PLACEMENT_3D('',#84501,#54505,#54506);
#44189=AXIS2_PLACEMENT_3D('',#84502,#54507,#54508);
#44190=AXIS2_PLACEMENT_3D('',#84506,#54509,#54510);
#44191=AXIS2_PLACEMENT_3D('',#84510,#54513,#54514);
#44192=AXIS2_PLACEMENT_3D('',#84514,#54517,#54518);
#44193=AXIS2_PLACEMENT_3D('',#84519,#54520,#54521);
#44194=AXIS2_PLACEMENT_3D('',#84520,#54522,#54523);
#44195=AXIS2_PLACEMENT_3D('',#84524,#54524,#54525);
#44196=AXIS2_PLACEMENT_3D('',#84528,#54528,#54529);
#44197=AXIS2_PLACEMENT_3D('',#84532,#54532,#54533);
#44198=AXIS2_PLACEMENT_3D('',#84537,#54535,#54536);
#44199=AXIS2_PLACEMENT_3D('',#84538,#54537,#54538);
#44200=AXIS2_PLACEMENT_3D('',#84542,#54539,#54540);
#44201=AXIS2_PLACEMENT_3D('',#84546,#54543,#54544);
#44202=AXIS2_PLACEMENT_3D('',#84550,#54547,#54548);
#44203=AXIS2_PLACEMENT_3D('',#84555,#54550,#54551);
#44204=AXIS2_PLACEMENT_3D('',#84556,#54552,#54553);
#44205=AXIS2_PLACEMENT_3D('',#84560,#54554,#54555);
#44206=AXIS2_PLACEMENT_3D('',#84564,#54558,#54559);
#44207=AXIS2_PLACEMENT_3D('',#84568,#54562,#54563);
#44208=AXIS2_PLACEMENT_3D('',#84573,#54565,#54566);
#44209=AXIS2_PLACEMENT_3D('',#84574,#54567,#54568);
#44210=AXIS2_PLACEMENT_3D('',#84578,#54569,#54570);
#44211=AXIS2_PLACEMENT_3D('',#84582,#54573,#54574);
#44212=AXIS2_PLACEMENT_3D('',#84586,#54577,#54578);
#44213=AXIS2_PLACEMENT_3D('',#84591,#54580,#54581);
#44214=AXIS2_PLACEMENT_3D('',#84592,#54582,#54583);
#44215=AXIS2_PLACEMENT_3D('',#84596,#54584,#54585);
#44216=AXIS2_PLACEMENT_3D('',#84600,#54588,#54589);
#44217=AXIS2_PLACEMENT_3D('',#84604,#54592,#54593);
#44218=AXIS2_PLACEMENT_3D('',#84609,#54595,#54596);
#44219=AXIS2_PLACEMENT_3D('',#84610,#54597,#54598);
#44220=AXIS2_PLACEMENT_3D('',#84614,#54599,#54600);
#44221=AXIS2_PLACEMENT_3D('',#84618,#54603,#54604);
#44222=AXIS2_PLACEMENT_3D('',#84622,#54607,#54608);
#44223=AXIS2_PLACEMENT_3D('',#84627,#54610,#54611);
#44224=AXIS2_PLACEMENT_3D('',#84628,#54612,#54613);
#44225=AXIS2_PLACEMENT_3D('',#84632,#54614,#54615);
#44226=AXIS2_PLACEMENT_3D('',#84636,#54618,#54619);
#44227=AXIS2_PLACEMENT_3D('',#84640,#54622,#54623);
#44228=AXIS2_PLACEMENT_3D('',#84645,#54625,#54626);
#44229=AXIS2_PLACEMENT_3D('',#84646,#54627,#54628);
#44230=AXIS2_PLACEMENT_3D('',#84650,#54629,#54630);
#44231=AXIS2_PLACEMENT_3D('',#84654,#54633,#54634);
#44232=AXIS2_PLACEMENT_3D('',#84658,#54637,#54638);
#44233=AXIS2_PLACEMENT_3D('',#84660,#54640,#54641);
#44234=AXIS2_PLACEMENT_3D('',#84661,#54642,#54643);
#53383=DIRECTION('axis',(0.,0.,1.));
#53384=DIRECTION('refdir',(1.,0.,0.));
#53385=DIRECTION('center_axis',(0.,0.258819045102522,0.965925826289068));
#53386=DIRECTION('ref_axis',(0.,-0.965925826289068,0.258819045102522));
#53387=DIRECTION('',(0.,0.965925826289068,-0.258819045102522));
#53388=DIRECTION('',(1.,0.,0.));
#53389=DIRECTION('',(0.,-0.965925826289068,0.258819045102522));
#53390=DIRECTION('',(-1.,0.,0.));
#53391=DIRECTION('center_axis',(1.,0.,0.));
#53392=DIRECTION('ref_axis',(0.,-0.258819045102522,-0.965925826289068));
#53393=DIRECTION('center_axis',(-1.,0.,0.));
#53394=DIRECTION('ref_axis',(0.,1.,0.));
#53395=DIRECTION('',(0.,-0.258819045102522,-0.965925826289068));
#53396=DIRECTION('',(0.,0.965925826289068,-0.258819045102522));
#53397=DIRECTION('center_axis',(0.,-0.258819045102522,-0.965925826289068));
#53398=DIRECTION('ref_axis',(0.,0.965925826289068,-0.258819045102522));
#53399=DIRECTION('',(0.,-0.965925826289068,0.258819045102522));
#53400=DIRECTION('',(1.,0.,0.));
#53401=DIRECTION('',(1.,0.,0.));
#53402=DIRECTION('center_axis',(0.,-0.965925826289068,0.258819045102522));
#53403=DIRECTION('ref_axis',(0.,-0.258819045102522,-0.965925826289068));
#53404=DIRECTION('',(0.,0.258819045102522,0.965925826289068));
#53405=DIRECTION('center_axis',(1.,0.,0.));
#53406=DIRECTION('ref_axis',(0.,1.,0.));
#53407=DIRECTION('center_axis',(1.,0.,0.));
#53408=DIRECTION('ref_axis',(0.,0.,-1.));
#53409=DIRECTION('',(-1.,0.,0.));
#53410=DIRECTION('center_axis',(-1.,0.,0.));
#53411=DIRECTION('ref_axis',(0.,1.,0.));
#53412=DIRECTION('',(1.,0.,0.));
#53413=DIRECTION('center_axis',(1.,0.,0.));
#53414=DIRECTION('ref_axis',(0.,0.,-1.));
#53415=DIRECTION('',(-1.,0.,0.));
#53416=DIRECTION('center_axis',(-1.,0.,0.));
#53417=DIRECTION('ref_axis',(0.,1.,0.));
#53418=DIRECTION('',(1.,0.,0.));
#53419=DIRECTION('center_axis',(1.,0.,0.));
#53420=DIRECTION('ref_axis',(0.,0.,-1.));
#53421=DIRECTION('',(-1.,0.,0.));
#53422=DIRECTION('center_axis',(-1.,0.,0.));
#53423=DIRECTION('ref_axis',(0.,1.,0.));
#53424=DIRECTION('',(1.,0.,0.));
#53425=DIRECTION('center_axis',(1.,0.,0.));
#53426=DIRECTION('ref_axis',(0.,0.,-1.));
#53427=DIRECTION('',(-1.,0.,0.));
#53428=DIRECTION('center_axis',(-1.,0.,0.));
#53429=DIRECTION('ref_axis',(0.,1.,0.));
#53430=DIRECTION('',(1.,0.,0.));
#53431=DIRECTION('center_axis',(1.,0.,0.));
#53432=DIRECTION('ref_axis',(0.,0.,-1.));
#53433=DIRECTION('',(-1.,0.,0.));
#53434=DIRECTION('center_axis',(-1.,0.,0.));
#53435=DIRECTION('ref_axis',(0.,1.,0.));
#53436=DIRECTION('',(1.,0.,0.));
#53437=DIRECTION('center_axis',(1.,0.,0.));
#53438=DIRECTION('ref_axis',(0.,0.,-1.));
#53439=DIRECTION('',(-1.,0.,0.));
#53440=DIRECTION('center_axis',(-1.,0.,0.));
#53441=DIRECTION('ref_axis',(0.,1.,0.));
#53442=DIRECTION('',(1.,0.,0.));
#53443=DIRECTION('center_axis',(1.,0.,0.));
#53444=DIRECTION('ref_axis',(0.,0.,-1.));
#53445=DIRECTION('',(-1.,0.,0.));
#53446=DIRECTION('center_axis',(-1.,0.,0.));
#53447=DIRECTION('ref_axis',(0.,1.,0.));
#53448=DIRECTION('',(1.,0.,0.));
#53449=DIRECTION('center_axis',(1.,0.,0.));
#53450=DIRECTION('ref_axis',(0.,0.,-1.));
#53451=DIRECTION('',(-1.,0.,0.));
#53452=DIRECTION('center_axis',(-1.,0.,0.));
#53453=DIRECTION('ref_axis',(0.,1.,0.));
#53454=DIRECTION('',(1.,0.,0.));
#53455=DIRECTION('center_axis',(1.,0.,0.));
#53456=DIRECTION('ref_axis',(0.,0.,-1.));
#53457=DIRECTION('',(-1.,0.,0.));
#53458=DIRECTION('center_axis',(-1.,0.,0.));
#53459=DIRECTION('ref_axis',(0.,1.,0.));
#53460=DIRECTION('',(1.,0.,0.));
#53461=DIRECTION('center_axis',(1.,0.,0.));
#53462=DIRECTION('ref_axis',(0.,0.,-1.));
#53463=DIRECTION('',(-1.,0.,0.));
#53464=DIRECTION('center_axis',(-1.,0.,0.));
#53465=DIRECTION('ref_axis',(0.,1.,0.));
#53466=DIRECTION('',(1.,0.,0.));
#53467=DIRECTION('center_axis',(1.,0.,0.));
#53468=DIRECTION('ref_axis',(0.,0.,-1.));
#53469=DIRECTION('',(-1.,0.,0.));
#53470=DIRECTION('center_axis',(-1.,0.,0.));
#53471=DIRECTION('ref_axis',(0.,1.,0.));
#53472=DIRECTION('',(-1.,0.,0.));
#53473=DIRECTION('center_axis',(1.,0.,0.));
#53474=DIRECTION('ref_axis',(0.,1.,0.));
#53475=DIRECTION('',(-1.,0.,0.));
#53476=DIRECTION('center_axis',(1.,0.,0.));
#53477=DIRECTION('ref_axis',(0.,0.,-1.));
#53478=DIRECTION('',(1.,0.,0.));
#53479=DIRECTION('center_axis',(1.,0.,0.));
#53480=DIRECTION('ref_axis',(0.,1.,0.));
#53481=DIRECTION('',(-1.,0.,0.));
#53482=DIRECTION('center_axis',(1.,0.,0.));
#53483=DIRECTION('ref_axis',(0.,0.,-1.));
#53484=DIRECTION('',(1.,0.,0.));
#53485=DIRECTION('center_axis',(1.,0.,0.));
#53486=DIRECTION('ref_axis',(0.,1.,0.));
#53487=DIRECTION('',(-1.,0.,0.));
#53488=DIRECTION('center_axis',(1.,0.,0.));
#53489=DIRECTION('ref_axis',(0.,0.,-1.));
#53490=DIRECTION('',(1.,0.,0.));
#53491=DIRECTION('center_axis',(1.,0.,0.));
#53492=DIRECTION('ref_axis',(0.,1.,0.));
#53493=DIRECTION('',(-1.,0.,0.));
#53494=DIRECTION('center_axis',(1.,0.,0.));
#53495=DIRECTION('ref_axis',(0.,0.,-1.));
#53496=DIRECTION('',(1.,0.,0.));
#53497=DIRECTION('center_axis',(1.,0.,0.));
#53498=DIRECTION('ref_axis',(0.,1.,0.));
#53499=DIRECTION('',(-1.,0.,0.));
#53500=DIRECTION('center_axis',(1.,0.,0.));
#53501=DIRECTION('ref_axis',(0.,0.,-1.));
#53502=DIRECTION('',(1.,0.,0.));
#53503=DIRECTION('center_axis',(1.,0.,0.));
#53504=DIRECTION('ref_axis',(0.,1.,0.));
#53505=DIRECTION('',(-1.,0.,0.));
#53506=DIRECTION('center_axis',(1.,0.,0.));
#53507=DIRECTION('ref_axis',(0.,0.,-1.));
#53508=DIRECTION('',(1.,0.,0.));
#53509=DIRECTION('center_axis',(1.,0.,0.));
#53510=DIRECTION('ref_axis',(0.,1.,0.));
#53511=DIRECTION('',(-1.,0.,0.));
#53512=DIRECTION('center_axis',(1.,0.,0.));
#53513=DIRECTION('ref_axis',(0.,0.,-1.));
#53514=DIRECTION('',(1.,0.,0.));
#53515=DIRECTION('center_axis',(1.,0.,0.));
#53516=DIRECTION('ref_axis',(0.,1.,0.));
#53517=DIRECTION('',(-1.,0.,0.));
#53518=DIRECTION('center_axis',(1.,0.,0.));
#53519=DIRECTION('ref_axis',(0.,0.,-1.));
#53520=DIRECTION('',(1.,0.,0.));
#53521=DIRECTION('center_axis',(1.,0.,0.));
#53522=DIRECTION('ref_axis',(0.,1.,0.));
#53523=DIRECTION('',(-1.,0.,0.));
#53524=DIRECTION('center_axis',(1.,0.,0.));
#53525=DIRECTION('ref_axis',(0.,0.,-1.));
#53526=DIRECTION('',(1.,0.,0.));
#53527=DIRECTION('center_axis',(1.,0.,0.));
#53528=DIRECTION('ref_axis',(0.,1.,0.));
#53529=DIRECTION('',(-1.,0.,0.));
#53530=DIRECTION('center_axis',(1.,0.,0.));
#53531=DIRECTION('ref_axis',(0.,0.,-1.));
#53532=DIRECTION('',(1.,0.,0.));
#53533=DIRECTION('center_axis',(1.,0.,0.));
#53534=DIRECTION('ref_axis',(0.,1.,0.));
#53535=DIRECTION('',(-1.,0.,0.));
#53536=DIRECTION('center_axis',(1.,0.,0.));
#53537=DIRECTION('ref_axis',(0.,0.,-1.));
#53538=DIRECTION('',(1.,0.,0.));
#53539=DIRECTION('center_axis',(1.,0.,0.));
#53540=DIRECTION('ref_axis',(0.,1.,0.));
#53541=DIRECTION('',(-1.,0.,0.));
#53542=DIRECTION('center_axis',(1.,0.,0.));
#53543=DIRECTION('ref_axis',(0.,0.,-1.));
#53544=DIRECTION('',(1.,0.,0.));
#53545=DIRECTION('center_axis',(1.,0.,0.));
#53546=DIRECTION('ref_axis',(0.,1.,0.));
#53547=DIRECTION('',(-1.,0.,0.));
#53548=DIRECTION('center_axis',(1.,0.,0.));
#53549=DIRECTION('ref_axis',(0.,0.,-1.));
#53550=DIRECTION('',(1.,0.,0.));
#53551=DIRECTION('center_axis',(1.,0.,0.));
#53552=DIRECTION('ref_axis',(0.,1.,0.));
#53553=DIRECTION('',(-1.,0.,0.));
#53554=DIRECTION('center_axis',(1.,0.,0.));
#53555=DIRECTION('ref_axis',(0.,0.,-1.));
#53556=DIRECTION('',(1.,0.,0.));
#53557=DIRECTION('center_axis',(1.,0.,0.));
#53558=DIRECTION('ref_axis',(0.,1.,0.));
#53559=DIRECTION('',(-1.,0.,0.));
#53560=DIRECTION('center_axis',(1.,0.,0.));
#53561=DIRECTION('ref_axis',(0.,0.,-1.));
#53562=DIRECTION('',(1.,0.,0.));
#53563=DIRECTION('center_axis',(1.,0.,0.));
#53564=DIRECTION('ref_axis',(0.,1.,0.));
#53565=DIRECTION('',(-1.,0.,0.));
#53566=DIRECTION('center_axis',(1.,0.,0.));
#53567=DIRECTION('ref_axis',(0.,0.,-1.));
#53568=DIRECTION('',(1.,0.,0.));
#53569=DIRECTION('center_axis',(1.,0.,0.));
#53570=DIRECTION('ref_axis',(0.,1.,0.));
#53571=DIRECTION('',(-1.,0.,0.));
#53572=DIRECTION('center_axis',(1.,0.,0.));
#53573=DIRECTION('ref_axis',(0.,0.,-1.));
#53574=DIRECTION('',(1.,0.,0.));
#53575=DIRECTION('center_axis',(1.,0.,0.));
#53576=DIRECTION('ref_axis',(0.,1.,0.));
#53577=DIRECTION('',(-1.,0.,0.));
#53578=DIRECTION('center_axis',(1.,0.,0.));
#53579=DIRECTION('ref_axis',(0.,0.,-1.));
#53580=DIRECTION('',(1.,0.,0.));
#53581=DIRECTION('center_axis',(1.,0.,0.));
#53582=DIRECTION('ref_axis',(0.,1.,0.));
#53583=DIRECTION('',(-1.,0.,0.));
#53584=DIRECTION('center_axis',(1.,0.,0.));
#53585=DIRECTION('ref_axis',(0.,0.,-1.));
#53586=DIRECTION('',(1.,0.,0.));
#53587=DIRECTION('center_axis',(1.,0.,0.));
#53588=DIRECTION('ref_axis',(0.,1.,0.));
#53589=DIRECTION('',(-1.,0.,0.));
#53590=DIRECTION('center_axis',(1.,0.,0.));
#53591=DIRECTION('ref_axis',(0.,0.,-1.));
#53592=DIRECTION('',(1.,0.,0.));
#53593=DIRECTION('center_axis',(1.,0.,0.));
#53594=DIRECTION('ref_axis',(0.,1.,0.));
#53595=DIRECTION('',(-1.,0.,0.));
#53596=DIRECTION('center_axis',(1.,0.,0.));
#53597=DIRECTION('ref_axis',(0.,0.,-1.));
#53598=DIRECTION('',(1.,0.,0.));
#53599=DIRECTION('center_axis',(1.,0.,0.));
#53600=DIRECTION('ref_axis',(0.,1.,0.));
#53601=DIRECTION('',(-1.,0.,0.));
#53602=DIRECTION('center_axis',(1.,0.,0.));
#53603=DIRECTION('ref_axis',(0.,0.,-1.));
#53604=DIRECTION('',(1.,0.,0.));
#53605=DIRECTION('center_axis',(1.,0.,0.));
#53606=DIRECTION('ref_axis',(0.,1.,0.));
#53607=DIRECTION('',(-1.,0.,0.));
#53608=DIRECTION('center_axis',(1.,0.,0.));
#53609=DIRECTION('ref_axis',(0.,0.,-1.));
#53610=DIRECTION('',(1.,0.,0.));
#53611=DIRECTION('center_axis',(1.,0.,0.));
#53612=DIRECTION('ref_axis',(0.,1.,0.));
#53613=DIRECTION('',(-1.,0.,0.));
#53614=DIRECTION('center_axis',(1.,0.,0.));
#53615=DIRECTION('ref_axis',(0.,0.,-1.));
#53616=DIRECTION('',(1.,0.,0.));
#53617=DIRECTION('center_axis',(1.,0.,0.));
#53618=DIRECTION('ref_axis',(0.,1.,0.));
#53619=DIRECTION('center_axis',(-1.,0.,0.));
#53620=DIRECTION('ref_axis',(0.,1.,0.));
#53621=DIRECTION('',(1.,0.,0.));
#53622=DIRECTION('center_axis',(1.,0.,0.));
#53623=DIRECTION('ref_axis',(0.,0.,-1.));
#53624=DIRECTION('',(-1.,0.,0.));
#53625=DIRECTION('center_axis',(-1.,0.,0.));
#53626=DIRECTION('ref_axis',(0.,1.,0.));
#53627=DIRECTION('',(1.,0.,0.));
#53628=DIRECTION('center_axis',(1.,0.,0.));
#53629=DIRECTION('ref_axis',(0.,0.,-1.));
#53630=DIRECTION('',(-1.,0.,0.));
#53631=DIRECTION('center_axis',(-1.,0.,0.));
#53632=DIRECTION('ref_axis',(0.,1.,0.));
#53633=DIRECTION('',(1.,0.,0.));
#53634=DIRECTION('center_axis',(1.,0.,0.));
#53635=DIRECTION('ref_axis',(0.,0.,-1.));
#53636=DIRECTION('',(-1.,0.,0.));
#53637=DIRECTION('center_axis',(-1.,0.,0.));
#53638=DIRECTION('ref_axis',(0.,1.,0.));
#53639=DIRECTION('',(1.,0.,0.));
#53640=DIRECTION('center_axis',(1.,0.,0.));
#53641=DIRECTION('ref_axis',(0.,0.,-1.));
#53642=DIRECTION('',(-1.,0.,0.));
#53643=DIRECTION('center_axis',(-1.,0.,0.));
#53644=DIRECTION('ref_axis',(0.,1.,0.));
#53645=DIRECTION('',(1.,0.,0.));
#53646=DIRECTION('center_axis',(1.,0.,0.));
#53647=DIRECTION('ref_axis',(0.,0.,-1.));
#53648=DIRECTION('',(-1.,0.,0.));
#53649=DIRECTION('center_axis',(-1.,0.,0.));
#53650=DIRECTION('ref_axis',(0.,1.,0.));
#53651=DIRECTION('',(1.,0.,0.));
#53652=DIRECTION('center_axis',(1.,0.,0.));
#53653=DIRECTION('ref_axis',(0.,0.,-1.));
#53654=DIRECTION('',(-1.,0.,0.));
#53655=DIRECTION('center_axis',(-1.,0.,0.));
#53656=DIRECTION('ref_axis',(0.,1.,0.));
#53657=DIRECTION('',(1.,0.,0.));
#53658=DIRECTION('center_axis',(1.,0.,0.));
#53659=DIRECTION('ref_axis',(0.,0.,-1.));
#53660=DIRECTION('',(-1.,0.,0.));
#53661=DIRECTION('center_axis',(-1.,0.,0.));
#53662=DIRECTION('ref_axis',(0.,1.,0.));
#53663=DIRECTION('',(1.,0.,0.));
#53664=DIRECTION('center_axis',(1.,0.,0.));
#53665=DIRECTION('ref_axis',(0.,0.,-1.));
#53666=DIRECTION('',(-1.,0.,0.));
#53667=DIRECTION('center_axis',(-1.,0.,0.));
#53668=DIRECTION('ref_axis',(0.,1.,0.));
#53669=DIRECTION('',(1.,0.,0.));
#53670=DIRECTION('center_axis',(1.,0.,0.));
#53671=DIRECTION('ref_axis',(0.,0.,-1.));
#53672=DIRECTION('',(-1.,0.,0.));
#53673=DIRECTION('center_axis',(-1.,0.,0.));
#53674=DIRECTION('ref_axis',(0.,1.,0.));
#53675=DIRECTION('',(1.,0.,0.));
#53676=DIRECTION('center_axis',(1.,0.,0.));
#53677=DIRECTION('ref_axis',(0.,0.,-1.));
#53678=DIRECTION('',(-1.,0.,0.));
#53679=DIRECTION('center_axis',(-1.,0.,0.));
#53680=DIRECTION('ref_axis',(0.,1.,0.));
#53681=DIRECTION('',(1.,0.,0.));
#53682=DIRECTION('center_axis',(1.,0.,0.));
#53683=DIRECTION('ref_axis',(0.,0.,-1.));
#53684=DIRECTION('',(-1.,0.,0.));
#53685=DIRECTION('center_axis',(-1.,0.,0.));
#53686=DIRECTION('ref_axis',(0.,1.,0.));
#53687=DIRECTION('',(1.,0.,0.));
#53688=DIRECTION('center_axis',(1.,0.,0.));
#53689=DIRECTION('ref_axis',(0.,0.,-1.));
#53690=DIRECTION('',(-1.,0.,0.));
#53691=DIRECTION('center_axis',(-1.,0.,0.));
#53692=DIRECTION('ref_axis',(0.,1.,0.));
#53693=DIRECTION('',(1.,0.,0.));
#53694=DIRECTION('center_axis',(1.,0.,0.));
#53695=DIRECTION('ref_axis',(0.,0.,-1.));
#53696=DIRECTION('center_axis',(-1.,0.,0.));
#53697=DIRECTION('ref_axis',(0.,1.,0.));
#53698=DIRECTION('center_axis',(1.,0.,0.));
#53699=DIRECTION('ref_axis',(0.,0.,-1.));
#53700=DIRECTION('center_axis',(-1.,0.,0.));
#53701=DIRECTION('ref_axis',(0.,1.,0.));
#53702=DIRECTION('center_axis',(1.,0.,0.));
#53703=DIRECTION('ref_axis',(0.,0.,-1.));
#53704=DIRECTION('center_axis',(0.,0.5,0.866025403784438));
#53705=DIRECTION('ref_axis',(0.,-0.866025403784438,0.5));
#53706=DIRECTION('',(0.,0.866025403784438,-0.5));
#53707=DIRECTION('',(1.,0.,0.));
#53708=DIRECTION('',(0.,-0.866025403784438,0.5));
#53709=DIRECTION('center_axis',(1.,0.,0.));
#53710=DIRECTION('ref_axis',(0.,-0.5,-0.866025403784438));
#53711=DIRECTION('',(0.,-0.5,-0.866025403784438));
#53712=DIRECTION('',(0.,0.866025403784438,-0.5));
#53713=DIRECTION('center_axis',(0.,-0.5,-0.866025403784438));
#53714=DIRECTION('ref_axis',(0.,0.866025403784438,-0.5));
#53715=DIRECTION('',(0.,-0.866025403784438,0.5));
#53716=DIRECTION('',(1.,0.,0.));
#53717=DIRECTION('center_axis',(0.,-0.866025403784438,0.5));
#53718=DIRECTION('ref_axis',(0.,-0.5,-0.866025403784438));
#53719=DIRECTION('',(0.,0.5,0.866025403784438));
#53720=DIRECTION('center_axis',(-1.,0.,0.));
#53721=DIRECTION('ref_axis',(0.,1.,0.));
#53722=DIRECTION('center_axis',(1.,0.,0.));
#53723=DIRECTION('ref_axis',(0.,0.,-1.));
#53724=DIRECTION('center_axis',(0.,0.707106781186548,0.707106781186547));
#53725=DIRECTION('ref_axis',(0.,-0.707106781186547,0.707106781186548));
#53726=DIRECTION('',(0.,0.707106781186547,-0.707106781186548));
#53727=DIRECTION('',(1.,0.,0.));
#53728=DIRECTION('',(0.,-0.707106781186547,0.707106781186548));
#53729=DIRECTION('center_axis',(1.,0.,0.));
#53730=DIRECTION('ref_axis',(0.,-0.707106781186548,-0.707106781186547));
#53731=DIRECTION('',(0.,-0.707106781186548,-0.707106781186547));
#53732=DIRECTION('',(0.,0.707106781186547,-0.707106781186548));
#53733=DIRECTION('center_axis',(0.,-0.707106781186548,-0.707106781186547));
#53734=DIRECTION('ref_axis',(0.,0.707106781186547,-0.707106781186548));
#53735=DIRECTION('',(0.,-0.707106781186547,0.707106781186548));
#53736=DIRECTION('',(1.,0.,0.));
#53737=DIRECTION('center_axis',(0.,-0.707106781186547,0.707106781186548));
#53738=DIRECTION('ref_axis',(0.,-0.707106781186548,-0.707106781186547));
#53739=DIRECTION('',(0.,0.707106781186548,0.707106781186547));
#53740=DIRECTION('center_axis',(-1.,0.,0.));
#53741=DIRECTION('ref_axis',(0.,1.,0.));
#53742=DIRECTION('center_axis',(1.,0.,0.));
#53743=DIRECTION('ref_axis',(0.,0.,-1.));
#53744=DIRECTION('center_axis',(0.,0.866025403784439,0.499999999999999));
#53745=DIRECTION('ref_axis',(0.,-0.499999999999999,0.866025403784439));
#53746=DIRECTION('',(0.,0.499999999999999,-0.866025403784439));
#53747=DIRECTION('',(1.,0.,0.));
#53748=DIRECTION('',(0.,-0.499999999999999,0.866025403784439));
#53749=DIRECTION('center_axis',(1.,0.,0.));
#53750=DIRECTION('ref_axis',(0.,-0.866025403784439,-0.499999999999999));
#53751=DIRECTION('',(0.,-0.866025403784439,-0.499999999999999));
#53752=DIRECTION('',(0.,0.499999999999999,-0.866025403784439));
#53753=DIRECTION('center_axis',(0.,-0.866025403784439,-0.499999999999999));
#53754=DIRECTION('ref_axis',(0.,0.499999999999999,-0.866025403784439));
#53755=DIRECTION('',(0.,-0.499999999999999,0.866025403784439));
#53756=DIRECTION('',(1.,0.,0.));
#53757=DIRECTION('center_axis',(0.,-0.499999999999999,0.866025403784439));
#53758=DIRECTION('ref_axis',(0.,-0.866025403784439,-0.499999999999999));
#53759=DIRECTION('',(0.,0.866025403784439,0.499999999999999));
#53760=DIRECTION('center_axis',(-1.,0.,0.));
#53761=DIRECTION('ref_axis',(0.,1.,0.));
#53762=DIRECTION('center_axis',(1.,0.,0.));
#53763=DIRECTION('ref_axis',(0.,0.,-1.));
#53764=DIRECTION('center_axis',(0.,0.965925826289068,0.25881904510252));
#53765=DIRECTION('ref_axis',(0.,-0.25881904510252,0.965925826289068));
#53766=DIRECTION('',(0.,0.25881904510252,-0.965925826289068));
#53767=DIRECTION('',(1.,0.,0.));
#53768=DIRECTION('',(0.,-0.25881904510252,0.965925826289068));
#53769=DIRECTION('center_axis',(1.,0.,0.));
#53770=DIRECTION('ref_axis',(0.,-0.965925826289068,-0.25881904510252));
#53771=DIRECTION('',(0.,-0.965925826289068,-0.25881904510252));
#53772=DIRECTION('',(0.,0.25881904510252,-0.965925826289068));
#53773=DIRECTION('center_axis',(0.,-0.965925826289068,-0.25881904510252));
#53774=DIRECTION('ref_axis',(0.,0.25881904510252,-0.965925826289068));
#53775=DIRECTION('',(0.,-0.25881904510252,0.965925826289068));
#53776=DIRECTION('',(1.,0.,0.));
#53777=DIRECTION('center_axis',(0.,-0.25881904510252,0.965925826289068));
#53778=DIRECTION('ref_axis',(0.,-0.965925826289068,-0.25881904510252));
#53779=DIRECTION('',(0.,0.965925826289068,0.25881904510252));
#53780=DIRECTION('center_axis',(-1.,0.,0.));
#53781=DIRECTION('ref_axis',(0.,1.,0.));
#53782=DIRECTION('center_axis',(1.,0.,0.));
#53783=DIRECTION('ref_axis',(0.,0.,-1.));
#53784=DIRECTION('center_axis',(0.,1.,-1.83697019872103E-16));
#53785=DIRECTION('ref_axis',(0.,1.83697019872103E-16,1.));
#53786=DIRECTION('',(0.,-1.83697019872103E-16,-1.));
#53787=DIRECTION('',(1.,0.,0.));
#53788=DIRECTION('',(0.,1.83697019872103E-16,1.));
#53789=DIRECTION('center_axis',(1.,0.,0.));
#53790=DIRECTION('ref_axis',(0.,-1.,1.83697019872103E-16));
#53791=DIRECTION('',(0.,-1.,1.83697019872103E-16));
#53792=DIRECTION('',(0.,-1.83697019872103E-16,-1.));
#53793=DIRECTION('center_axis',(0.,-1.,1.83697019872103E-16));
#53794=DIRECTION('ref_axis',(0.,-1.83697019872103E-16,-1.));
#53795=DIRECTION('',(0.,1.83697019872103E-16,1.));
#53796=DIRECTION('',(1.,0.,0.));
#53797=DIRECTION('center_axis',(0.,1.83697019872103E-16,1.));
#53798=DIRECTION('ref_axis',(0.,-1.,1.83697019872103E-16));
#53799=DIRECTION('',(0.,1.,-1.83697019872103E-16));
#53800=DIRECTION('center_axis',(-1.,0.,0.));
#53801=DIRECTION('ref_axis',(0.,1.,0.));
#53802=DIRECTION('center_axis',(1.,0.,0.));
#53803=DIRECTION('ref_axis',(0.,0.,-1.));
#53804=DIRECTION('center_axis',(0.,0.965925826289068,-0.258819045102522));
#53805=DIRECTION('ref_axis',(0.,0.258819045102522,0.965925826289068));
#53806=DIRECTION('',(0.,-0.258819045102522,-0.965925826289068));
#53807=DIRECTION('',(1.,0.,0.));
#53808=DIRECTION('',(0.,0.258819045102522,0.965925826289068));
#53809=DIRECTION('center_axis',(1.,0.,0.));
#53810=DIRECTION('ref_axis',(0.,-0.965925826289068,0.258819045102522));
#53811=DIRECTION('',(0.,-0.965925826289068,0.258819045102522));
#53812=DIRECTION('',(0.,-0.258819045102522,-0.965925826289068));
#53813=DIRECTION('center_axis',(0.,-0.965925826289068,0.258819045102522));
#53814=DIRECTION('ref_axis',(0.,-0.258819045102522,-0.965925826289068));
#53815=DIRECTION('',(0.,0.258819045102522,0.965925826289068));
#53816=DIRECTION('',(1.,0.,0.));
#53817=DIRECTION('center_axis',(0.,0.258819045102522,0.965925826289068));
#53818=DIRECTION('ref_axis',(0.,-0.965925826289068,0.258819045102522));
#53819=DIRECTION('',(0.,0.965925826289068,-0.258819045102522));
#53820=DIRECTION('center_axis',(-1.,0.,0.));
#53821=DIRECTION('ref_axis',(0.,1.,0.));
#53822=DIRECTION('center_axis',(1.,0.,0.));
#53823=DIRECTION('ref_axis',(0.,0.,-1.));
#53824=DIRECTION('center_axis',(0.,0.866025403784438,-0.5));
#53825=DIRECTION('ref_axis',(0.,0.5,0.866025403784438));
#53826=DIRECTION('',(0.,-0.5,-0.866025403784438));
#53827=DIRECTION('',(1.,0.,0.));
#53828=DIRECTION('',(0.,0.5,0.866025403784438));
#53829=DIRECTION('center_axis',(1.,0.,0.));
#53830=DIRECTION('ref_axis',(0.,-0.866025403784438,0.5));
#53831=DIRECTION('',(0.,-0.866025403784438,0.5));
#53832=DIRECTION('',(0.,-0.5,-0.866025403784438));
#53833=DIRECTION('center_axis',(0.,-0.866025403784438,0.5));
#53834=DIRECTION('ref_axis',(0.,-0.5,-0.866025403784438));
#53835=DIRECTION('',(0.,0.5,0.866025403784438));
#53836=DIRECTION('',(1.,0.,0.));
#53837=DIRECTION('center_axis',(0.,0.5,0.866025403784438));
#53838=DIRECTION('ref_axis',(0.,-0.866025403784438,0.5));
#53839=DIRECTION('',(0.,0.866025403784438,-0.5));
#53840=DIRECTION('center_axis',(-1.,0.,0.));
#53841=DIRECTION('ref_axis',(0.,1.,0.));
#53842=DIRECTION('center_axis',(1.,0.,0.));
#53843=DIRECTION('ref_axis',(0.,0.,-1.));
#53844=DIRECTION('center_axis',(0.,0.707106781186547,-0.707106781186548));
#53845=DIRECTION('ref_axis',(0.,0.707106781186548,0.707106781186547));
#53846=DIRECTION('',(0.,-0.707106781186548,-0.707106781186547));
#53847=DIRECTION('',(1.,0.,0.));
#53848=DIRECTION('',(0.,0.707106781186548,0.707106781186547));
#53849=DIRECTION('center_axis',(1.,0.,0.));
#53850=DIRECTION('ref_axis',(0.,-0.707106781186547,0.707106781186548));
#53851=DIRECTION('',(0.,-0.707106781186547,0.707106781186548));
#53852=DIRECTION('',(0.,-0.707106781186548,-0.707106781186547));
#53853=DIRECTION('center_axis',(0.,-0.707106781186547,0.707106781186548));
#53854=DIRECTION('ref_axis',(0.,-0.707106781186548,-0.707106781186547));
#53855=DIRECTION('',(0.,0.707106781186548,0.707106781186547));
#53856=DIRECTION('',(1.,0.,0.));
#53857=DIRECTION('center_axis',(0.,0.707106781186548,0.707106781186547));
#53858=DIRECTION('ref_axis',(0.,-0.707106781186547,0.707106781186548));
#53859=DIRECTION('',(0.,0.707106781186547,-0.707106781186548));
#53860=DIRECTION('center_axis',(-1.,0.,0.));
#53861=DIRECTION('ref_axis',(0.,1.,0.));
#53862=DIRECTION('center_axis',(1.,0.,0.));
#53863=DIRECTION('ref_axis',(0.,0.,-1.));
#53864=DIRECTION('center_axis',(0.,0.5,-0.866025403784439));
#53865=DIRECTION('ref_axis',(0.,0.866025403784439,0.5));
#53866=DIRECTION('',(0.,-0.866025403784439,-0.5));
#53867=DIRECTION('',(1.,0.,0.));
#53868=DIRECTION('',(0.,0.866025403784439,0.5));
#53869=DIRECTION('center_axis',(1.,0.,0.));
#53870=DIRECTION('ref_axis',(0.,-0.5,0.866025403784439));
#53871=DIRECTION('',(0.,-0.5,0.866025403784439));
#53872=DIRECTION('',(0.,-0.866025403784439,-0.5));
#53873=DIRECTION('center_axis',(0.,-0.5,0.866025403784439));
#53874=DIRECTION('ref_axis',(0.,-0.866025403784439,-0.5));
#53875=DIRECTION('',(0.,0.866025403784439,0.5));
#53876=DIRECTION('',(1.,0.,0.));
#53877=DIRECTION('center_axis',(0.,0.866025403784439,0.5));
#53878=DIRECTION('ref_axis',(0.,-0.5,0.866025403784439));
#53879=DIRECTION('',(0.,0.5,-0.866025403784439));
#53880=DIRECTION('center_axis',(-1.,0.,0.));
#53881=DIRECTION('ref_axis',(0.,1.,0.));
#53882=DIRECTION('center_axis',(1.,0.,0.));
#53883=DIRECTION('ref_axis',(0.,0.,-1.));
#53884=DIRECTION('center_axis',(0.,0.25881904510252,-0.965925826289068));
#53885=DIRECTION('ref_axis',(0.,0.965925826289068,0.25881904510252));
#53886=DIRECTION('',(0.,-0.965925826289068,-0.25881904510252));
#53887=DIRECTION('',(1.,0.,0.));
#53888=DIRECTION('',(0.,0.965925826289068,0.25881904510252));
#53889=DIRECTION('center_axis',(1.,0.,0.));
#53890=DIRECTION('ref_axis',(0.,-0.25881904510252,0.965925826289068));
#53891=DIRECTION('',(0.,-0.25881904510252,0.965925826289068));
#53892=DIRECTION('',(0.,-0.965925826289068,-0.25881904510252));
#53893=DIRECTION('center_axis',(0.,-0.25881904510252,0.965925826289068));
#53894=DIRECTION('ref_axis',(0.,-0.965925826289068,-0.25881904510252));
#53895=DIRECTION('',(0.,0.965925826289068,0.25881904510252));
#53896=DIRECTION('',(1.,0.,0.));
#53897=DIRECTION('center_axis',(0.,0.965925826289068,0.25881904510252));
#53898=DIRECTION('ref_axis',(0.,-0.25881904510252,0.965925826289068));
#53899=DIRECTION('',(0.,0.25881904510252,-0.965925826289068));
#53900=DIRECTION('center_axis',(-1.,0.,0.));
#53901=DIRECTION('ref_axis',(0.,1.,0.));
#53902=DIRECTION('center_axis',(1.,0.,0.));
#53903=DIRECTION('ref_axis',(0.,0.,-1.));
#53904=DIRECTION('center_axis',(0.,-1.22464679914735E-16,-1.));
#53905=DIRECTION('ref_axis',(0.,1.,-1.22464679914735E-16));
#53906=DIRECTION('',(0.,-1.,1.22464679914735E-16));
#53907=DIRECTION('',(1.,0.,0.));
#53908=DIRECTION('',(0.,1.,-1.22464679914735E-16));
#53909=DIRECTION('center_axis',(1.,0.,0.));
#53910=DIRECTION('ref_axis',(0.,1.22464679914735E-16,1.));
#53911=DIRECTION('',(0.,1.22464679914735E-16,1.));
#53912=DIRECTION('',(0.,-1.,1.22464679914735E-16));
#53913=DIRECTION('center_axis',(0.,1.22464679914735E-16,1.));
#53914=DIRECTION('ref_axis',(0.,-1.,1.22464679914735E-16));
#53915=DIRECTION('',(0.,1.,-1.22464679914735E-16));
#53916=DIRECTION('',(1.,0.,0.));
#53917=DIRECTION('center_axis',(0.,1.,-1.22464679914735E-16));
#53918=DIRECTION('ref_axis',(0.,1.22464679914735E-16,1.));
#53919=DIRECTION('',(0.,-1.22464679914735E-16,-1.));
#53920=DIRECTION('center_axis',(-1.,0.,0.));
#53921=DIRECTION('ref_axis',(0.,1.,0.));
#53922=DIRECTION('center_axis',(1.,0.,0.));
#53923=DIRECTION('ref_axis',(0.,0.,-1.));
#53924=DIRECTION('center_axis',(0.,-0.258819045102521,-0.965925826289068));
#53925=DIRECTION('ref_axis',(0.,0.965925826289068,-0.258819045102521));
#53926=DIRECTION('',(0.,-0.965925826289068,0.258819045102521));
#53927=DIRECTION('',(1.,0.,0.));
#53928=DIRECTION('',(0.,0.965925826289068,-0.258819045102521));
#53929=DIRECTION('center_axis',(1.,0.,0.));
#53930=DIRECTION('ref_axis',(0.,0.258819045102521,0.965925826289068));
#53931=DIRECTION('',(0.,0.258819045102521,0.965925826289068));
#53932=DIRECTION('',(0.,-0.965925826289068,0.258819045102521));
#53933=DIRECTION('center_axis',(0.,0.258819045102521,0.965925826289068));
#53934=DIRECTION('ref_axis',(0.,-0.965925826289068,0.258819045102521));
#53935=DIRECTION('',(0.,0.965925826289068,-0.258819045102521));
#53936=DIRECTION('',(1.,0.,0.));
#53937=DIRECTION('center_axis',(0.,0.965925826289068,-0.258819045102521));
#53938=DIRECTION('ref_axis',(0.,0.258819045102521,0.965925826289068));
#53939=DIRECTION('',(0.,-0.258819045102521,-0.965925826289068));
#53940=DIRECTION('center_axis',(-1.,0.,0.));
#53941=DIRECTION('ref_axis',(0.,1.,0.));
#53942=DIRECTION('center_axis',(1.,0.,0.));
#53943=DIRECTION('ref_axis',(0.,0.,-1.));
#53944=DIRECTION('center_axis',(0.,-0.5,-0.866025403784438));
#53945=DIRECTION('ref_axis',(0.,0.866025403784438,-0.5));
#53946=DIRECTION('',(0.,-0.866025403784438,0.5));
#53947=DIRECTION('',(1.,0.,0.));
#53948=DIRECTION('',(0.,0.866025403784438,-0.5));
#53949=DIRECTION('center_axis',(1.,0.,0.));
#53950=DIRECTION('ref_axis',(0.,0.5,0.866025403784438));
#53951=DIRECTION('',(0.,0.5,0.866025403784438));
#53952=DIRECTION('',(0.,-0.866025403784438,0.5));
#53953=DIRECTION('center_axis',(0.,0.5,0.866025403784438));
#53954=DIRECTION('ref_axis',(0.,-0.866025403784438,0.5));
#53955=DIRECTION('',(0.,0.866025403784438,-0.5));
#53956=DIRECTION('',(1.,0.,0.));
#53957=DIRECTION('center_axis',(0.,0.866025403784438,-0.5));
#53958=DIRECTION('ref_axis',(0.,0.5,0.866025403784438));
#53959=DIRECTION('',(0.,-0.5,-0.866025403784438));
#53960=DIRECTION('center_axis',(-1.,0.,0.));
#53961=DIRECTION('ref_axis',(0.,1.,0.));
#53962=DIRECTION('center_axis',(1.,0.,0.));
#53963=DIRECTION('ref_axis',(0.,0.,-1.));
#53964=DIRECTION('center_axis',(0.,-0.707106781186548,-0.707106781186547));
#53965=DIRECTION('ref_axis',(0.,0.707106781186547,-0.707106781186548));
#53966=DIRECTION('',(0.,-0.707106781186547,0.707106781186548));
#53967=DIRECTION('',(1.,0.,0.));
#53968=DIRECTION('',(0.,0.707106781186547,-0.707106781186548));
#53969=DIRECTION('center_axis',(1.,0.,0.));
#53970=DIRECTION('ref_axis',(0.,0.707106781186548,0.707106781186547));
#53971=DIRECTION('',(0.,0.707106781186548,0.707106781186547));
#53972=DIRECTION('',(0.,-0.707106781186547,0.707106781186548));
#53973=DIRECTION('center_axis',(0.,0.707106781186548,0.707106781186547));
#53974=DIRECTION('ref_axis',(0.,-0.707106781186547,0.707106781186548));
#53975=DIRECTION('',(0.,0.707106781186547,-0.707106781186548));
#53976=DIRECTION('',(1.,0.,0.));
#53977=DIRECTION('center_axis',(0.,0.707106781186547,-0.707106781186548));
#53978=DIRECTION('ref_axis',(0.,0.707106781186548,0.707106781186547));
#53979=DIRECTION('',(0.,-0.707106781186548,-0.707106781186547));
#53980=DIRECTION('center_axis',(-1.,0.,0.));
#53981=DIRECTION('ref_axis',(0.,1.,0.));
#53982=DIRECTION('center_axis',(1.,0.,0.));
#53983=DIRECTION('ref_axis',(0.,0.,-1.));
#53984=DIRECTION('center_axis',(0.,-0.866025403784439,-0.5));
#53985=DIRECTION('ref_axis',(0.,0.5,-0.866025403784439));
#53986=DIRECTION('',(0.,-0.5,0.866025403784439));
#53987=DIRECTION('',(1.,0.,0.));
#53988=DIRECTION('',(0.,0.5,-0.866025403784439));
#53989=DIRECTION('center_axis',(1.,0.,0.));
#53990=DIRECTION('ref_axis',(0.,0.866025403784439,0.5));
#53991=DIRECTION('',(0.,0.866025403784439,0.5));
#53992=DIRECTION('',(0.,-0.5,0.866025403784439));
#53993=DIRECTION('center_axis',(0.,0.866025403784439,0.5));
#53994=DIRECTION('ref_axis',(0.,-0.5,0.866025403784439));
#53995=DIRECTION('',(0.,0.5,-0.866025403784439));
#53996=DIRECTION('',(1.,0.,0.));
#53997=DIRECTION('center_axis',(0.,0.5,-0.866025403784439));
#53998=DIRECTION('ref_axis',(0.,0.866025403784439,0.5));
#53999=DIRECTION('',(0.,-0.866025403784439,-0.5));
#54000=DIRECTION('center_axis',(-1.,0.,0.));
#54001=DIRECTION('ref_axis',(0.,1.,0.));
#54002=DIRECTION('center_axis',(1.,0.,0.));
#54003=DIRECTION('ref_axis',(0.,0.,-1.));
#54004=DIRECTION('center_axis',(0.,-0.965925826289068,-0.258819045102521));
#54005=DIRECTION('ref_axis',(0.,0.258819045102521,-0.965925826289068));
#54006=DIRECTION('',(0.,-0.258819045102521,0.965925826289068));
#54007=DIRECTION('',(1.,0.,0.));
#54008=DIRECTION('',(0.,0.258819045102521,-0.965925826289068));
#54009=DIRECTION('center_axis',(1.,0.,0.));
#54010=DIRECTION('ref_axis',(0.,0.965925826289068,0.258819045102521));
#54011=DIRECTION('',(0.,0.965925826289068,0.258819045102521));
#54012=DIRECTION('',(0.,-0.258819045102521,0.965925826289068));
#54013=DIRECTION('center_axis',(0.,0.965925826289068,0.258819045102521));
#54014=DIRECTION('ref_axis',(0.,-0.258819045102521,0.965925826289068));
#54015=DIRECTION('',(0.,0.258819045102521,-0.965925826289068));
#54016=DIRECTION('',(1.,0.,0.));
#54017=DIRECTION('center_axis',(0.,0.258819045102521,-0.965925826289068));
#54018=DIRECTION('ref_axis',(0.,0.965925826289068,0.258819045102521));
#54019=DIRECTION('',(0.,-0.965925826289068,-0.258819045102521));
#54020=DIRECTION('center_axis',(-1.,0.,0.));
#54021=DIRECTION('ref_axis',(0.,1.,0.));
#54022=DIRECTION('center_axis',(1.,0.,0.));
#54023=DIRECTION('ref_axis',(0.,0.,-1.));
#54024=DIRECTION('center_axis',(0.,-1.,6.12323399573677E-17));
#54025=DIRECTION('ref_axis',(0.,-6.12323399573677E-17,-1.));
#54026=DIRECTION('',(0.,6.12323399573677E-17,1.));
#54027=DIRECTION('',(1.,0.,0.));
#54028=DIRECTION('',(0.,-6.12323399573677E-17,-1.));
#54029=DIRECTION('center_axis',(1.,0.,0.));
#54030=DIRECTION('ref_axis',(0.,1.,-6.12323399573677E-17));
#54031=DIRECTION('',(0.,1.,-6.12323399573677E-17));
#54032=DIRECTION('',(0.,6.12323399573677E-17,1.));
#54033=DIRECTION('center_axis',(0.,1.,-6.12323399573677E-17));
#54034=DIRECTION('ref_axis',(0.,6.12323399573677E-17,1.));
#54035=DIRECTION('',(0.,-6.12323399573677E-17,-1.));
#54036=DIRECTION('',(1.,0.,0.));
#54037=DIRECTION('center_axis',(0.,-6.12323399573677E-17,-1.));
#54038=DIRECTION('ref_axis',(0.,1.,-6.12323399573677E-17));
#54039=DIRECTION('',(0.,-1.,6.12323399573677E-17));
#54040=DIRECTION('center_axis',(-1.,0.,0.));
#54041=DIRECTION('ref_axis',(0.,1.,0.));
#54042=DIRECTION('center_axis',(1.,0.,0.));
#54043=DIRECTION('ref_axis',(0.,0.,-1.));
#54044=DIRECTION('center_axis',(0.,-0.965925826289068,0.258819045102521));
#54045=DIRECTION('ref_axis',(0.,-0.258819045102521,-0.965925826289068));
#54046=DIRECTION('',(0.,0.258819045102521,0.965925826289068));
#54047=DIRECTION('',(1.,0.,0.));
#54048=DIRECTION('',(0.,-0.258819045102521,-0.965925826289068));
#54049=DIRECTION('center_axis',(1.,0.,0.));
#54050=DIRECTION('ref_axis',(0.,0.965925826289068,-0.258819045102521));
#54051=DIRECTION('',(0.,0.965925826289068,-0.258819045102521));
#54052=DIRECTION('',(0.,0.258819045102521,0.965925826289068));
#54053=DIRECTION('center_axis',(0.,0.965925826289068,-0.258819045102521));
#54054=DIRECTION('ref_axis',(0.,0.258819045102521,0.965925826289068));
#54055=DIRECTION('',(0.,-0.258819045102521,-0.965925826289068));
#54056=DIRECTION('',(1.,0.,0.));
#54057=DIRECTION('center_axis',(0.,-0.258819045102521,-0.965925826289068));
#54058=DIRECTION('ref_axis',(0.,0.965925826289068,-0.258819045102521));
#54059=DIRECTION('',(0.,-0.965925826289068,0.258819045102521));
#54060=DIRECTION('center_axis',(-1.,0.,0.));
#54061=DIRECTION('ref_axis',(0.,1.,0.));
#54062=DIRECTION('center_axis',(1.,0.,0.));
#54063=DIRECTION('ref_axis',(0.,0.,-1.));
#54064=DIRECTION('center_axis',(0.,-0.866025403784439,0.5));
#54065=DIRECTION('ref_axis',(0.,-0.5,-0.866025403784439));
#54066=DIRECTION('',(0.,0.5,0.866025403784439));
#54067=DIRECTION('',(1.,0.,0.));
#54068=DIRECTION('',(0.,-0.5,-0.866025403784439));
#54069=DIRECTION('center_axis',(1.,0.,0.));
#54070=DIRECTION('ref_axis',(0.,0.866025403784439,-0.5));
#54071=DIRECTION('',(0.,0.866025403784439,-0.5));
#54072=DIRECTION('',(0.,0.5,0.866025403784439));
#54073=DIRECTION('center_axis',(0.,0.866025403784439,-0.5));
#54074=DIRECTION('ref_axis',(0.,0.5,0.866025403784439));
#54075=DIRECTION('',(0.,-0.5,-0.866025403784439));
#54076=DIRECTION('',(1.,0.,0.));
#54077=DIRECTION('center_axis',(0.,-0.5,-0.866025403784439));
#54078=DIRECTION('ref_axis',(0.,0.866025403784439,-0.5));
#54079=DIRECTION('',(0.,-0.866025403784439,0.5));
#54080=DIRECTION('center_axis',(-1.,0.,0.));
#54081=DIRECTION('ref_axis',(0.,1.,0.));
#54082=DIRECTION('center_axis',(1.,0.,0.));
#54083=DIRECTION('ref_axis',(0.,0.,-1.));
#54084=DIRECTION('center_axis',(0.,-0.707106781186548,0.707106781186548));
#54085=DIRECTION('ref_axis',(0.,-0.707106781186548,-0.707106781186548));
#54086=DIRECTION('',(0.,0.707106781186548,0.707106781186548));
#54087=DIRECTION('',(1.,0.,0.));
#54088=DIRECTION('',(0.,-0.707106781186548,-0.707106781186548));
#54089=DIRECTION('center_axis',(1.,0.,0.));
#54090=DIRECTION('ref_axis',(0.,0.707106781186548,-0.707106781186548));
#54091=DIRECTION('',(0.,0.707106781186548,-0.707106781186548));
#54092=DIRECTION('',(0.,0.707106781186548,0.707106781186548));
#54093=DIRECTION('center_axis',(0.,0.707106781186548,-0.707106781186548));
#54094=DIRECTION('ref_axis',(0.,0.707106781186548,0.707106781186548));
#54095=DIRECTION('',(0.,-0.707106781186548,-0.707106781186548));
#54096=DIRECTION('',(1.,0.,0.));
#54097=DIRECTION('center_axis',(0.,-0.707106781186548,-0.707106781186548));
#54098=DIRECTION('ref_axis',(0.,0.707106781186548,-0.707106781186548));
#54099=DIRECTION('',(0.,-0.707106781186548,0.707106781186548));
#54100=DIRECTION('center_axis',(-1.,0.,0.));
#54101=DIRECTION('ref_axis',(0.,1.,0.));
#54102=DIRECTION('center_axis',(1.,0.,0.));
#54103=DIRECTION('ref_axis',(0.,0.,-1.));
#54104=DIRECTION('center_axis',(0.,-0.5,0.866025403784439));
#54105=DIRECTION('ref_axis',(0.,-0.866025403784439,-0.5));
#54106=DIRECTION('',(0.,0.866025403784439,0.5));
#54107=DIRECTION('',(1.,0.,0.));
#54108=DIRECTION('',(0.,-0.866025403784439,-0.5));
#54109=DIRECTION('center_axis',(1.,0.,0.));
#54110=DIRECTION('ref_axis',(0.,0.5,-0.866025403784439));
#54111=DIRECTION('',(0.,0.5,-0.866025403784439));
#54112=DIRECTION('',(0.,0.866025403784439,0.5));
#54113=DIRECTION('center_axis',(0.,0.5,-0.866025403784439));
#54114=DIRECTION('ref_axis',(0.,0.866025403784439,0.5));
#54115=DIRECTION('',(0.,-0.866025403784439,-0.5));
#54116=DIRECTION('',(1.,0.,0.));
#54117=DIRECTION('center_axis',(0.,-0.866025403784439,-0.5));
#54118=DIRECTION('ref_axis',(0.,0.5,-0.866025403784439));
#54119=DIRECTION('',(0.,-0.5,0.866025403784439));
#54120=DIRECTION('center_axis',(-1.,0.,0.));
#54121=DIRECTION('ref_axis',(0.,1.,0.));
#54122=DIRECTION('center_axis',(1.,0.,0.));
#54123=DIRECTION('ref_axis',(0.,0.,-1.));
#54124=DIRECTION('center_axis',(0.,-0.258819045102521,0.965925826289068));
#54125=DIRECTION('ref_axis',(0.,-0.965925826289068,-0.258819045102521));
#54126=DIRECTION('',(0.,0.965925826289068,0.258819045102521));
#54127=DIRECTION('',(1.,0.,0.));
#54128=DIRECTION('',(0.,-0.965925826289068,-0.258819045102521));
#54129=DIRECTION('center_axis',(1.,0.,0.));
#54130=DIRECTION('ref_axis',(0.,0.258819045102521,-0.965925826289068));
#54131=DIRECTION('',(0.,0.258819045102521,-0.965925826289068));
#54132=DIRECTION('',(0.,0.965925826289068,0.258819045102521));
#54133=DIRECTION('center_axis',(0.,0.258819045102521,-0.965925826289068));
#54134=DIRECTION('ref_axis',(0.,0.965925826289068,0.258819045102521));
#54135=DIRECTION('',(0.,-0.965925826289068,-0.258819045102521));
#54136=DIRECTION('',(1.,0.,0.));
#54137=DIRECTION('center_axis',(0.,-0.965925826289068,-0.258819045102521));
#54138=DIRECTION('ref_axis',(0.,0.258819045102521,-0.965925826289068));
#54139=DIRECTION('',(0.,-0.258819045102521,0.965925826289068));
#54140=DIRECTION('center_axis',(-1.,0.,0.));
#54141=DIRECTION('ref_axis',(0.,1.,0.));
#54142=DIRECTION('center_axis',(1.,0.,0.));
#54143=DIRECTION('ref_axis',(0.,0.,-1.));
#54144=DIRECTION('center_axis',(0.,0.,1.));
#54145=DIRECTION('ref_axis',(0.,-1.,0.));
#54146=DIRECTION('',(0.,1.,0.));
#54147=DIRECTION('',(1.,0.,0.));
#54148=DIRECTION('',(0.,-1.,0.));
#54149=DIRECTION('center_axis',(1.,0.,0.));
#54150=DIRECTION('ref_axis',(0.,0.,-1.));
#54151=DIRECTION('',(0.,0.,-1.));
#54152=DIRECTION('',(0.,1.,0.));
#54153=DIRECTION('center_axis',(0.,0.,-1.));
#54154=DIRECTION('ref_axis',(0.,1.,0.));
#54155=DIRECTION('',(0.,-1.,0.));
#54156=DIRECTION('',(1.,0.,0.));
#54157=DIRECTION('center_axis',(0.,-1.,0.));
#54158=DIRECTION('ref_axis',(0.,0.,-1.));
#54159=DIRECTION('',(0.,0.,1.));
#54160=DIRECTION('center_axis',(0.,0.258819045102522,0.965925826289068));
#54161=DIRECTION('ref_axis',(0.,-0.965925826289068,0.258819045102522));
#54162=DIRECTION('',(0.,-0.965925826289068,0.258819045102522));
#54163=DIRECTION('',(1.,0.,0.));
#54164=DIRECTION('',(0.,-0.965925826289068,0.258819045102522));
#54165=DIRECTION('center_axis',(0.,-0.965925826289068,0.258819045102522));
#54166=DIRECTION('ref_axis',(0.,-0.258819045102522,-0.965925826289068));
#54167=DIRECTION('',(0.,-0.258819045102522,-0.965925826289068));
#54168=DIRECTION('',(0.,-0.258819045102522,-0.965925826289068));
#54169=DIRECTION('',(1.,0.,0.));
#54170=DIRECTION('center_axis',(0.,-0.258819045102522,-0.965925826289068));
#54171=DIRECTION('ref_axis',(0.,0.965925826289068,-0.258819045102522));
#54172=DIRECTION('',(0.,0.965925826289068,-0.258819045102522));
#54173=DIRECTION('',(0.,0.965925826289068,-0.258819045102522));
#54174=DIRECTION('center_axis',(1.,0.,0.));
#54175=DIRECTION('ref_axis',(0.,-0.258819045102522,-0.965925826289068));
#54176=DIRECTION('center_axis',(-1.,0.,0.));
#54177=DIRECTION('ref_axis',(0.,0.,1.));
#54178=DIRECTION('center_axis',(1.,0.,0.));
#54179=DIRECTION('ref_axis',(0.,0.,-1.));
#54180=DIRECTION('',(0.,-0.866025403784438,0.5));
#54181=DIRECTION('',(0.,-0.5,-0.866025403784438));
#54182=DIRECTION('',(0.,0.866025403784438,-0.5));
#54183=DIRECTION('center_axis',(1.,0.,0.));
#54184=DIRECTION('ref_axis',(0.,0.,-1.));
#54185=DIRECTION('',(0.,-0.707106781186547,0.707106781186548));
#54186=DIRECTION('',(0.,-0.707106781186548,-0.707106781186547));
#54187=DIRECTION('',(0.,0.707106781186547,-0.707106781186548));
#54188=DIRECTION('center_axis',(1.,0.,0.));
#54189=DIRECTION('ref_axis',(0.,0.,-1.));
#54190=DIRECTION('',(0.,-0.499999999999999,0.866025403784439));
#54191=DIRECTION('',(0.,-0.866025403784439,-0.499999999999999));
#54192=DIRECTION('',(0.,0.499999999999999,-0.866025403784439));
#54193=DIRECTION('center_axis',(1.,0.,0.));
#54194=DIRECTION('ref_axis',(0.,0.,-1.));
#54195=DIRECTION('',(0.,-0.25881904510252,0.965925826289068));
#54196=DIRECTION('',(0.,-0.965925826289068,-0.25881904510252));
#54197=DIRECTION('',(0.,0.25881904510252,-0.965925826289068));
#54198=DIRECTION('center_axis',(1.,0.,0.));
#54199=DIRECTION('ref_axis',(0.,0.,-1.));
#54200=DIRECTION('',(0.,1.83697019872103E-16,1.));
#54201=DIRECTION('',(0.,-1.,1.83697019872103E-16));
#54202=DIRECTION('',(0.,-1.83697019872103E-16,-1.));
#54203=DIRECTION('center_axis',(1.,0.,0.));
#54204=DIRECTION('ref_axis',(0.,0.,-1.));
#54205=DIRECTION('',(0.,0.258819045102522,0.965925826289068));
#54206=DIRECTION('',(0.,-0.965925826289068,0.258819045102522));
#54207=DIRECTION('',(0.,-0.258819045102522,-0.965925826289068));
#54208=DIRECTION('center_axis',(1.,0.,0.));
#54209=DIRECTION('ref_axis',(0.,0.,-1.));
#54210=DIRECTION('',(0.,0.5,0.866025403784438));
#54211=DIRECTION('',(0.,-0.866025403784438,0.5));
#54212=DIRECTION('',(0.,-0.5,-0.866025403784438));
#54213=DIRECTION('center_axis',(1.,0.,0.));
#54214=DIRECTION('ref_axis',(0.,0.,-1.));
#54215=DIRECTION('',(0.,0.707106781186548,0.707106781186547));
#54216=DIRECTION('',(0.,-0.707106781186547,0.707106781186548));
#54217=DIRECTION('',(0.,-0.707106781186548,-0.707106781186547));
#54218=DIRECTION('center_axis',(1.,0.,0.));
#54219=DIRECTION('ref_axis',(0.,0.,-1.));
#54220=DIRECTION('',(0.,0.866025403784439,0.5));
#54221=DIRECTION('',(0.,-0.5,0.866025403784439));
#54222=DIRECTION('',(0.,-0.866025403784439,-0.5));
#54223=DIRECTION('center_axis',(1.,0.,0.));
#54224=DIRECTION('ref_axis',(0.,0.,-1.));
#54225=DIRECTION('',(0.,0.965925826289068,0.25881904510252));
#54226=DIRECTION('',(0.,-0.25881904510252,0.965925826289068));
#54227=DIRECTION('',(0.,-0.965925826289068,-0.25881904510252));
#54228=DIRECTION('center_axis',(1.,0.,0.));
#54229=DIRECTION('ref_axis',(0.,0.,-1.));
#54230=DIRECTION('',(0.,1.,-1.22464679914735E-16));
#54231=DIRECTION('',(0.,1.22464679914735E-16,1.));
#54232=DIRECTION('',(0.,-1.,1.22464679914735E-16));
#54233=DIRECTION('center_axis',(1.,0.,0.));
#54234=DIRECTION('ref_axis',(0.,0.,-1.));
#54235=DIRECTION('',(0.,0.965925826289068,-0.258819045102521));
#54236=DIRECTION('',(0.,0.258819045102521,0.965925826289068));
#54237=DIRECTION('',(0.,-0.965925826289068,0.258819045102521));
#54238=DIRECTION('center_axis',(1.,0.,0.));
#54239=DIRECTION('ref_axis',(0.,0.,-1.));
#54240=DIRECTION('',(0.,0.866025403784438,-0.5));
#54241=DIRECTION('',(0.,0.5,0.866025403784438));
#54242=DIRECTION('',(0.,-0.866025403784438,0.5));
#54243=DIRECTION('center_axis',(1.,0.,0.));
#54244=DIRECTION('ref_axis',(0.,0.,-1.));
#54245=DIRECTION('',(0.,0.707106781186547,-0.707106781186548));
#54246=DIRECTION('',(0.,0.707106781186548,0.707106781186547));
#54247=DIRECTION('',(0.,-0.707106781186547,0.707106781186548));
#54248=DIRECTION('center_axis',(1.,0.,0.));
#54249=DIRECTION('ref_axis',(0.,0.,-1.));
#54250=DIRECTION('',(0.,0.5,-0.866025403784439));
#54251=DIRECTION('',(0.,0.866025403784439,0.5));
#54252=DIRECTION('',(0.,-0.5,0.866025403784439));
#54253=DIRECTION('center_axis',(1.,0.,0.));
#54254=DIRECTION('ref_axis',(0.,0.,-1.));
#54255=DIRECTION('',(0.,0.258819045102521,-0.965925826289068));
#54256=DIRECTION('',(0.,0.965925826289068,0.258819045102521));
#54257=DIRECTION('',(0.,-0.258819045102521,0.965925826289068));
#54258=DIRECTION('center_axis',(1.,0.,0.));
#54259=DIRECTION('ref_axis',(0.,0.,-1.));
#54260=DIRECTION('',(0.,-6.12323399573677E-17,-1.));
#54261=DIRECTION('',(0.,1.,-6.12323399573677E-17));
#54262=DIRECTION('',(0.,6.12323399573677E-17,1.));
#54263=DIRECTION('center_axis',(1.,0.,0.));
#54264=DIRECTION('ref_axis',(0.,0.,-1.));
#54265=DIRECTION('',(0.,-0.258819045102521,-0.965925826289068));
#54266=DIRECTION('',(0.,0.965925826289068,-0.258819045102521));
#54267=DIRECTION('',(0.,0.258819045102521,0.965925826289068));
#54268=DIRECTION('center_axis',(1.,0.,0.));
#54269=DIRECTION('ref_axis',(0.,0.,-1.));
#54270=DIRECTION('',(0.,-0.5,-0.866025403784439));
#54271=DIRECTION('',(0.,0.866025403784439,-0.5));
#54272=DIRECTION('',(0.,0.5,0.866025403784439));
#54273=DIRECTION('center_axis',(1.,0.,0.));
#54274=DIRECTION('ref_axis',(0.,0.,-1.));
#54275=DIRECTION('',(0.,-0.707106781186548,-0.707106781186548));
#54276=DIRECTION('',(0.,0.707106781186548,-0.707106781186548));
#54277=DIRECTION('',(0.,0.707106781186548,0.707106781186548));
#54278=DIRECTION('center_axis',(1.,0.,0.));
#54279=DIRECTION('ref_axis',(0.,0.,-1.));
#54280=DIRECTION('',(0.,-0.866025403784439,-0.5));
#54281=DIRECTION('',(0.,0.5,-0.866025403784439));
#54282=DIRECTION('',(0.,0.866025403784439,0.5));
#54283=DIRECTION('center_axis',(1.,0.,0.));
#54284=DIRECTION('ref_axis',(0.,0.,-1.));
#54285=DIRECTION('',(0.,-0.965925826289068,-0.258819045102521));
#54286=DIRECTION('',(0.,0.258819045102521,-0.965925826289068));
#54287=DIRECTION('',(0.,0.965925826289068,0.258819045102521));
#54288=DIRECTION('center_axis',(1.,0.,0.));
#54289=DIRECTION('ref_axis',(0.,0.,-1.));
#54290=DIRECTION('',(0.,-1.,0.));
#54291=DIRECTION('',(0.,0.,-1.));
#54292=DIRECTION('',(0.,1.,0.));
#54293=DIRECTION('center_axis',(1.,0.,0.));
#54294=DIRECTION('ref_axis',(0.,0.,-1.));
#54295=DIRECTION('center_axis',(1.,0.,0.));
#54296=DIRECTION('ref_axis',(0.,1.,0.));
#54297=DIRECTION('center_axis',(1.,0.,0.));
#54298=DIRECTION('ref_axis',(0.,1.,0.));
#54299=DIRECTION('center_axis',(0.,0.5,0.866025403784438));
#54300=DIRECTION('ref_axis',(0.,-0.866025403784438,0.5));
#54301=DIRECTION('',(0.,-0.866025403784438,0.5));
#54302=DIRECTION('',(1.,0.,0.));
#54303=DIRECTION('center_axis',(0.,-0.866025403784438,0.5));
#54304=DIRECTION('ref_axis',(0.,-0.5,-0.866025403784438));
#54305=DIRECTION('',(0.,-0.5,-0.866025403784438));
#54306=DIRECTION('',(1.,0.,0.));
#54307=DIRECTION('center_axis',(0.,-0.5,-0.866025403784438));
#54308=DIRECTION('ref_axis',(0.,0.866025403784438,-0.5));
#54309=DIRECTION('',(0.,0.866025403784438,-0.5));
#54310=DIRECTION('center_axis',(1.,0.,0.));
#54311=DIRECTION('ref_axis',(0.,-0.5,-0.866025403784438));
#54312=DIRECTION('center_axis',(1.,0.,0.));
#54313=DIRECTION('ref_axis',(0.,1.,0.));
#54314=DIRECTION('center_axis',(0.,0.707106781186548,0.707106781186547));
#54315=DIRECTION('ref_axis',(0.,-0.707106781186547,0.707106781186548));
#54316=DIRECTION('',(0.,-0.707106781186547,0.707106781186548));
#54317=DIRECTION('',(1.,0.,0.));
#54318=DIRECTION('center_axis',(0.,-0.707106781186547,0.707106781186548));
#54319=DIRECTION('ref_axis',(0.,-0.707106781186548,-0.707106781186547));
#54320=DIRECTION('',(0.,-0.707106781186548,-0.707106781186547));
#54321=DIRECTION('',(1.,0.,0.));
#54322=DIRECTION('center_axis',(0.,-0.707106781186548,-0.707106781186547));
#54323=DIRECTION('ref_axis',(0.,0.707106781186547,-0.707106781186548));
#54324=DIRECTION('',(0.,0.707106781186547,-0.707106781186548));
#54325=DIRECTION('center_axis',(1.,0.,0.));
#54326=DIRECTION('ref_axis',(0.,-0.707106781186548,-0.707106781186547));
#54327=DIRECTION('center_axis',(1.,0.,0.));
#54328=DIRECTION('ref_axis',(0.,1.,0.));
#54329=DIRECTION('center_axis',(0.,0.866025403784439,0.499999999999999));
#54330=DIRECTION('ref_axis',(0.,-0.499999999999999,0.866025403784439));
#54331=DIRECTION('',(0.,-0.499999999999999,0.866025403784439));
#54332=DIRECTION('',(1.,0.,0.));
#54333=DIRECTION('center_axis',(0.,-0.499999999999999,0.866025403784439));
#54334=DIRECTION('ref_axis',(0.,-0.866025403784439,-0.499999999999999));
#54335=DIRECTION('',(0.,-0.866025403784439,-0.499999999999999));
#54336=DIRECTION('',(1.,0.,0.));
#54337=DIRECTION('center_axis',(0.,-0.866025403784439,-0.499999999999999));
#54338=DIRECTION('ref_axis',(0.,0.499999999999999,-0.866025403784439));
#54339=DIRECTION('',(0.,0.499999999999999,-0.866025403784439));
#54340=DIRECTION('center_axis',(1.,0.,0.));
#54341=DIRECTION('ref_axis',(0.,-0.866025403784439,-0.499999999999999));
#54342=DIRECTION('center_axis',(1.,0.,0.));
#54343=DIRECTION('ref_axis',(0.,1.,0.));
#54344=DIRECTION('center_axis',(0.,0.965925826289068,0.25881904510252));
#54345=DIRECTION('ref_axis',(0.,-0.25881904510252,0.965925826289068));
#54346=DIRECTION('',(0.,-0.25881904510252,0.965925826289068));
#54347=DIRECTION('',(1.,0.,0.));
#54348=DIRECTION('center_axis',(0.,-0.25881904510252,0.965925826289068));
#54349=DIRECTION('ref_axis',(0.,-0.965925826289068,-0.25881904510252));
#54350=DIRECTION('',(0.,-0.965925826289068,-0.25881904510252));
#54351=DIRECTION('',(1.,0.,0.));
#54352=DIRECTION('center_axis',(0.,-0.965925826289068,-0.25881904510252));
#54353=DIRECTION('ref_axis',(0.,0.25881904510252,-0.965925826289068));
#54354=DIRECTION('',(0.,0.25881904510252,-0.965925826289068));
#54355=DIRECTION('center_axis',(1.,0.,0.));
#54356=DIRECTION('ref_axis',(0.,-0.965925826289068,-0.25881904510252));
#54357=DIRECTION('center_axis',(1.,0.,0.));
#54358=DIRECTION('ref_axis',(0.,1.,0.));
#54359=DIRECTION('center_axis',(0.,1.,-1.83697019872103E-16));
#54360=DIRECTION('ref_axis',(0.,1.83697019872103E-16,1.));
#54361=DIRECTION('',(0.,1.83697019872103E-16,1.));
#54362=DIRECTION('',(1.,0.,0.));
#54363=DIRECTION('center_axis',(0.,1.83697019872103E-16,1.));
#54364=DIRECTION('ref_axis',(0.,-1.,1.83697019872103E-16));
#54365=DIRECTION('',(0.,-1.,1.83697019872103E-16));
#54366=DIRECTION('',(1.,0.,0.));
#54367=DIRECTION('center_axis',(0.,-1.,1.83697019872103E-16));
#54368=DIRECTION('ref_axis',(0.,-1.83697019872103E-16,-1.));
#54369=DIRECTION('',(0.,-1.83697019872103E-16,-1.));
#54370=DIRECTION('center_axis',(1.,0.,0.));
#54371=DIRECTION('ref_axis',(0.,-1.,1.83697019872103E-16));
#54372=DIRECTION('center_axis',(1.,0.,0.));
#54373=DIRECTION('ref_axis',(0.,1.,0.));
#54374=DIRECTION('center_axis',(0.,0.965925826289068,-0.258819045102522));
#54375=DIRECTION('ref_axis',(0.,0.258819045102522,0.965925826289068));
#54376=DIRECTION('',(0.,0.258819045102522,0.965925826289068));
#54377=DIRECTION('',(1.,0.,0.));
#54378=DIRECTION('center_axis',(0.,0.258819045102522,0.965925826289068));
#54379=DIRECTION('ref_axis',(0.,-0.965925826289068,0.258819045102522));
#54380=DIRECTION('',(0.,-0.965925826289068,0.258819045102522));
#54381=DIRECTION('',(1.,0.,0.));
#54382=DIRECTION('center_axis',(0.,-0.965925826289068,0.258819045102522));
#54383=DIRECTION('ref_axis',(0.,-0.258819045102522,-0.965925826289068));
#54384=DIRECTION('',(0.,-0.258819045102522,-0.965925826289068));
#54385=DIRECTION('center_axis',(1.,0.,0.));
#54386=DIRECTION('ref_axis',(0.,-0.965925826289068,0.258819045102522));
#54387=DIRECTION('center_axis',(1.,0.,0.));
#54388=DIRECTION('ref_axis',(0.,1.,0.));
#54389=DIRECTION('center_axis',(0.,0.866025403784438,-0.5));
#54390=DIRECTION('ref_axis',(0.,0.5,0.866025403784438));
#54391=DIRECTION('',(0.,0.5,0.866025403784438));
#54392=DIRECTION('',(1.,0.,0.));
#54393=DIRECTION('center_axis',(0.,0.5,0.866025403784438));
#54394=DIRECTION('ref_axis',(0.,-0.866025403784438,0.5));
#54395=DIRECTION('',(0.,-0.866025403784438,0.5));
#54396=DIRECTION('',(1.,0.,0.));
#54397=DIRECTION('center_axis',(0.,-0.866025403784438,0.5));
#54398=DIRECTION('ref_axis',(0.,-0.5,-0.866025403784438));
#54399=DIRECTION('',(0.,-0.5,-0.866025403784438));
#54400=DIRECTION('center_axis',(1.,0.,0.));
#54401=DIRECTION('ref_axis',(0.,-0.866025403784438,0.5));
#54402=DIRECTION('center_axis',(1.,0.,0.));
#54403=DIRECTION('ref_axis',(0.,1.,0.));
#54404=DIRECTION('center_axis',(0.,0.707106781186547,-0.707106781186548));
#54405=DIRECTION('ref_axis',(0.,0.707106781186548,0.707106781186547));
#54406=DIRECTION('',(0.,0.707106781186548,0.707106781186547));
#54407=DIRECTION('',(1.,0.,0.));
#54408=DIRECTION('center_axis',(0.,0.707106781186548,0.707106781186547));
#54409=DIRECTION('ref_axis',(0.,-0.707106781186547,0.707106781186548));
#54410=DIRECTION('',(0.,-0.707106781186547,0.707106781186548));
#54411=DIRECTION('',(1.,0.,0.));
#54412=DIRECTION('center_axis',(0.,-0.707106781186547,0.707106781186548));
#54413=DIRECTION('ref_axis',(0.,-0.707106781186548,-0.707106781186547));
#54414=DIRECTION('',(0.,-0.707106781186548,-0.707106781186547));
#54415=DIRECTION('center_axis',(1.,0.,0.));
#54416=DIRECTION('ref_axis',(0.,-0.707106781186547,0.707106781186548));
#54417=DIRECTION('center_axis',(1.,0.,0.));
#54418=DIRECTION('ref_axis',(0.,1.,0.));
#54419=DIRECTION('center_axis',(0.,0.5,-0.866025403784439));
#54420=DIRECTION('ref_axis',(0.,0.866025403784439,0.5));
#54421=DIRECTION('',(0.,0.866025403784439,0.5));
#54422=DIRECTION('',(1.,0.,0.));
#54423=DIRECTION('center_axis',(0.,0.866025403784439,0.5));
#54424=DIRECTION('ref_axis',(0.,-0.5,0.866025403784439));
#54425=DIRECTION('',(0.,-0.5,0.866025403784439));
#54426=DIRECTION('',(1.,0.,0.));
#54427=DIRECTION('center_axis',(0.,-0.5,0.866025403784439));
#54428=DIRECTION('ref_axis',(0.,-0.866025403784439,-0.5));
#54429=DIRECTION('',(0.,-0.866025403784439,-0.5));
#54430=DIRECTION('center_axis',(1.,0.,0.));
#54431=DIRECTION('ref_axis',(0.,-0.5,0.866025403784439));
#54432=DIRECTION('center_axis',(1.,0.,0.));
#54433=DIRECTION('ref_axis',(0.,1.,0.));
#54434=DIRECTION('center_axis',(0.,0.25881904510252,-0.965925826289068));
#54435=DIRECTION('ref_axis',(0.,0.965925826289068,0.25881904510252));
#54436=DIRECTION('',(0.,0.965925826289068,0.25881904510252));
#54437=DIRECTION('',(1.,0.,0.));
#54438=DIRECTION('center_axis',(0.,0.965925826289068,0.25881904510252));
#54439=DIRECTION('ref_axis',(0.,-0.25881904510252,0.965925826289068));
#54440=DIRECTION('',(0.,-0.25881904510252,0.965925826289068));
#54441=DIRECTION('',(1.,0.,0.));
#54442=DIRECTION('center_axis',(0.,-0.25881904510252,0.965925826289068));
#54443=DIRECTION('ref_axis',(0.,-0.965925826289068,-0.25881904510252));
#54444=DIRECTION('',(0.,-0.965925826289068,-0.25881904510252));
#54445=DIRECTION('center_axis',(1.,0.,0.));
#54446=DIRECTION('ref_axis',(0.,-0.25881904510252,0.965925826289068));
#54447=DIRECTION('center_axis',(1.,0.,0.));
#54448=DIRECTION('ref_axis',(0.,1.,0.));
#54449=DIRECTION('center_axis',(0.,-1.22464679914735E-16,-1.));
#54450=DIRECTION('ref_axis',(0.,1.,-1.22464679914735E-16));
#54451=DIRECTION('',(0.,1.,-1.22464679914735E-16));
#54452=DIRECTION('',(1.,0.,0.));
#54453=DIRECTION('center_axis',(0.,1.,-1.22464679914735E-16));
#54454=DIRECTION('ref_axis',(0.,1.22464679914735E-16,1.));
#54455=DIRECTION('',(0.,1.22464679914735E-16,1.));
#54456=DIRECTION('',(1.,0.,0.));
#54457=DIRECTION('center_axis',(0.,1.22464679914735E-16,1.));
#54458=DIRECTION('ref_axis',(0.,-1.,1.22464679914735E-16));
#54459=DIRECTION('',(0.,-1.,1.22464679914735E-16));
#54460=DIRECTION('center_axis',(1.,0.,0.));
#54461=DIRECTION('ref_axis',(0.,1.22464679914735E-16,1.));
#54462=DIRECTION('center_axis',(1.,0.,0.));
#54463=DIRECTION('ref_axis',(0.,1.,0.));
#54464=DIRECTION('center_axis',(0.,-0.258819045102521,-0.965925826289068));
#54465=DIRECTION('ref_axis',(0.,0.965925826289068,-0.258819045102521));
#54466=DIRECTION('',(0.,0.965925826289068,-0.258819045102521));
#54467=DIRECTION('',(1.,0.,0.));
#54468=DIRECTION('center_axis',(0.,0.965925826289068,-0.258819045102521));
#54469=DIRECTION('ref_axis',(0.,0.258819045102521,0.965925826289068));
#54470=DIRECTION('',(0.,0.258819045102521,0.965925826289068));
#54471=DIRECTION('',(1.,0.,0.));
#54472=DIRECTION('center_axis',(0.,0.258819045102521,0.965925826289068));
#54473=DIRECTION('ref_axis',(0.,-0.965925826289068,0.258819045102521));
#54474=DIRECTION('',(0.,-0.965925826289068,0.258819045102521));
#54475=DIRECTION('center_axis',(1.,0.,0.));
#54476=DIRECTION('ref_axis',(0.,0.258819045102521,0.965925826289068));
#54477=DIRECTION('center_axis',(1.,0.,0.));
#54478=DIRECTION('ref_axis',(0.,1.,0.));
#54479=DIRECTION('center_axis',(0.,-0.5,-0.866025403784438));
#54480=DIRECTION('ref_axis',(0.,0.866025403784438,-0.5));
#54481=DIRECTION('',(0.,0.866025403784438,-0.5));
#54482=DIRECTION('',(1.,0.,0.));
#54483=DIRECTION('center_axis',(0.,0.866025403784438,-0.5));
#54484=DIRECTION('ref_axis',(0.,0.5,0.866025403784438));
#54485=DIRECTION('',(0.,0.5,0.866025403784438));
#54486=DIRECTION('',(1.,0.,0.));
#54487=DIRECTION('center_axis',(0.,0.5,0.866025403784438));
#54488=DIRECTION('ref_axis',(0.,-0.866025403784438,0.5));
#54489=DIRECTION('',(0.,-0.866025403784438,0.5));
#54490=DIRECTION('center_axis',(1.,0.,0.));
#54491=DIRECTION('ref_axis',(0.,0.5,0.866025403784438));
#54492=DIRECTION('center_axis',(1.,0.,0.));
#54493=DIRECTION('ref_axis',(0.,1.,0.));
#54494=DIRECTION('center_axis',(0.,-0.707106781186548,-0.707106781186547));
#54495=DIRECTION('ref_axis',(0.,0.707106781186547,-0.707106781186548));
#54496=DIRECTION('',(0.,0.707106781186547,-0.707106781186548));
#54497=DIRECTION('',(1.,0.,0.));
#54498=DIRECTION('center_axis',(0.,0.707106781186547,-0.707106781186548));
#54499=DIRECTION('ref_axis',(0.,0.707106781186548,0.707106781186547));
#54500=DIRECTION('',(0.,0.707106781186548,0.707106781186547));
#54501=DIRECTION('',(1.,0.,0.));
#54502=DIRECTION('center_axis',(0.,0.707106781186548,0.707106781186547));
#54503=DIRECTION('ref_axis',(0.,-0.707106781186547,0.707106781186548));
#54504=DIRECTION('',(0.,-0.707106781186547,0.707106781186548));
#54505=DIRECTION('center_axis',(1.,0.,0.));
#54506=DIRECTION('ref_axis',(0.,0.707106781186548,0.707106781186547));
#54507=DIRECTION('center_axis',(1.,0.,0.));
#54508=DIRECTION('ref_axis',(0.,1.,0.));
#54509=DIRECTION('center_axis',(0.,-0.866025403784439,-0.5));
#54510=DIRECTION('ref_axis',(0.,0.5,-0.866025403784439));
#54511=DIRECTION('',(0.,0.5,-0.866025403784439));
#54512=DIRECTION('',(1.,0.,0.));
#54513=DIRECTION('center_axis',(0.,0.5,-0.866025403784439));
#54514=DIRECTION('ref_axis',(0.,0.866025403784439,0.5));
#54515=DIRECTION('',(0.,0.866025403784439,0.5));
#54516=DIRECTION('',(1.,0.,0.));
#54517=DIRECTION('center_axis',(0.,0.866025403784439,0.5));
#54518=DIRECTION('ref_axis',(0.,-0.5,0.866025403784439));
#54519=DIRECTION('',(0.,-0.5,0.866025403784439));
#54520=DIRECTION('center_axis',(1.,0.,0.));
#54521=DIRECTION('ref_axis',(0.,0.866025403784439,0.5));
#54522=DIRECTION('center_axis',(1.,0.,0.));
#54523=DIRECTION('ref_axis',(0.,1.,0.));
#54524=DIRECTION('center_axis',(0.,-0.965925826289068,-0.258819045102521));
#54525=DIRECTION('ref_axis',(0.,0.258819045102521,-0.965925826289068));
#54526=DIRECTION('',(0.,0.258819045102521,-0.965925826289068));
#54527=DIRECTION('',(1.,0.,0.));
#54528=DIRECTION('center_axis',(0.,0.258819045102521,-0.965925826289068));
#54529=DIRECTION('ref_axis',(0.,0.965925826289068,0.258819045102521));
#54530=DIRECTION('',(0.,0.965925826289068,0.258819045102521));
#54531=DIRECTION('',(1.,0.,0.));
#54532=DIRECTION('center_axis',(0.,0.965925826289068,0.258819045102521));
#54533=DIRECTION('ref_axis',(0.,-0.258819045102521,0.965925826289068));
#54534=DIRECTION('',(0.,-0.258819045102521,0.965925826289068));
#54535=DIRECTION('center_axis',(1.,0.,0.));
#54536=DIRECTION('ref_axis',(0.,0.965925826289068,0.258819045102521));
#54537=DIRECTION('center_axis',(1.,0.,0.));
#54538=DIRECTION('ref_axis',(0.,1.,0.));
#54539=DIRECTION('center_axis',(0.,-1.,6.12323399573677E-17));
#54540=DIRECTION('ref_axis',(0.,-6.12323399573677E-17,-1.));
#54541=DIRECTION('',(0.,-6.12323399573677E-17,-1.));
#54542=DIRECTION('',(1.,0.,0.));
#54543=DIRECTION('center_axis',(0.,-6.12323399573677E-17,-1.));
#54544=DIRECTION('ref_axis',(0.,1.,-6.12323399573677E-17));
#54545=DIRECTION('',(0.,1.,-6.12323399573677E-17));
#54546=DIRECTION('',(1.,0.,0.));
#54547=DIRECTION('center_axis',(0.,1.,-6.12323399573677E-17));
#54548=DIRECTION('ref_axis',(0.,6.12323399573677E-17,1.));
#54549=DIRECTION('',(0.,6.12323399573677E-17,1.));
#54550=DIRECTION('center_axis',(1.,0.,0.));
#54551=DIRECTION('ref_axis',(0.,1.,-6.12323399573677E-17));
#54552=DIRECTION('center_axis',(1.,0.,0.));
#54553=DIRECTION('ref_axis',(0.,1.,0.));
#54554=DIRECTION('center_axis',(0.,-0.965925826289068,0.258819045102521));
#54555=DIRECTION('ref_axis',(0.,-0.258819045102521,-0.965925826289068));
#54556=DIRECTION('',(0.,-0.258819045102521,-0.965925826289068));
#54557=DIRECTION('',(1.,0.,0.));
#54558=DIRECTION('center_axis',(0.,-0.258819045102521,-0.965925826289068));
#54559=DIRECTION('ref_axis',(0.,0.965925826289068,-0.258819045102521));
#54560=DIRECTION('',(0.,0.965925826289068,-0.258819045102521));
#54561=DIRECTION('',(1.,0.,0.));
#54562=DIRECTION('center_axis',(0.,0.965925826289068,-0.258819045102521));
#54563=DIRECTION('ref_axis',(0.,0.258819045102521,0.965925826289068));
#54564=DIRECTION('',(0.,0.258819045102521,0.965925826289068));
#54565=DIRECTION('center_axis',(1.,0.,0.));
#54566=DIRECTION('ref_axis',(0.,0.965925826289068,-0.258819045102521));
#54567=DIRECTION('center_axis',(1.,0.,0.));
#54568=DIRECTION('ref_axis',(0.,1.,0.));
#54569=DIRECTION('center_axis',(0.,-0.866025403784439,0.5));
#54570=DIRECTION('ref_axis',(0.,-0.5,-0.866025403784439));
#54571=DIRECTION('',(0.,-0.5,-0.866025403784439));
#54572=DIRECTION('',(1.,0.,0.));
#54573=DIRECTION('center_axis',(0.,-0.5,-0.866025403784439));
#54574=DIRECTION('ref_axis',(0.,0.866025403784439,-0.5));
#54575=DIRECTION('',(0.,0.866025403784439,-0.5));
#54576=DIRECTION('',(1.,0.,0.));
#54577=DIRECTION('center_axis',(0.,0.866025403784439,-0.5));
#54578=DIRECTION('ref_axis',(0.,0.5,0.866025403784439));
#54579=DIRECTION('',(0.,0.5,0.866025403784439));
#54580=DIRECTION('center_axis',(1.,0.,0.));
#54581=DIRECTION('ref_axis',(0.,0.866025403784439,-0.5));
#54582=DIRECTION('center_axis',(1.,0.,0.));
#54583=DIRECTION('ref_axis',(0.,1.,0.));
#54584=DIRECTION('center_axis',(0.,-0.707106781186548,0.707106781186548));
#54585=DIRECTION('ref_axis',(0.,-0.707106781186548,-0.707106781186548));
#54586=DIRECTION('',(0.,-0.707106781186548,-0.707106781186548));
#54587=DIRECTION('',(1.,0.,0.));
#54588=DIRECTION('center_axis',(0.,-0.707106781186548,-0.707106781186548));
#54589=DIRECTION('ref_axis',(0.,0.707106781186548,-0.707106781186548));
#54590=DIRECTION('',(0.,0.707106781186548,-0.707106781186548));
#54591=DIRECTION('',(1.,0.,0.));
#54592=DIRECTION('center_axis',(0.,0.707106781186548,-0.707106781186548));
#54593=DIRECTION('ref_axis',(0.,0.707106781186548,0.707106781186548));
#54594=DIRECTION('',(0.,0.707106781186548,0.707106781186548));
#54595=DIRECTION('center_axis',(1.,0.,0.));
#54596=DIRECTION('ref_axis',(0.,0.707106781186548,-0.707106781186548));
#54597=DIRECTION('center_axis',(1.,0.,0.));
#54598=DIRECTION('ref_axis',(0.,1.,0.));
#54599=DIRECTION('center_axis',(0.,-0.5,0.866025403784439));
#54600=DIRECTION('ref_axis',(0.,-0.866025403784439,-0.5));
#54601=DIRECTION('',(0.,-0.866025403784439,-0.5));
#54602=DIRECTION('',(1.,0.,0.));
#54603=DIRECTION('center_axis',(0.,-0.866025403784439,-0.5));
#54604=DIRECTION('ref_axis',(0.,0.5,-0.866025403784439));
#54605=DIRECTION('',(0.,0.5,-0.866025403784439));
#54606=DIRECTION('',(1.,0.,0.));
#54607=DIRECTION('center_axis',(0.,0.5,-0.866025403784439));
#54608=DIRECTION('ref_axis',(0.,0.866025403784439,0.5));
#54609=DIRECTION('',(0.,0.866025403784439,0.5));
#54610=DIRECTION('center_axis',(1.,0.,0.));
#54611=DIRECTION('ref_axis',(0.,0.5,-0.866025403784439));
#54612=DIRECTION('center_axis',(1.,0.,0.));
#54613=DIRECTION('ref_axis',(0.,1.,0.));
#54614=DIRECTION('center_axis',(0.,-0.258819045102521,0.965925826289068));
#54615=DIRECTION('ref_axis',(0.,-0.965925826289068,-0.258819045102521));
#54616=DIRECTION('',(0.,-0.965925826289068,-0.258819045102521));
#54617=DIRECTION('',(1.,0.,0.));
#54618=DIRECTION('center_axis',(0.,-0.965925826289068,-0.258819045102521));
#54619=DIRECTION('ref_axis',(0.,0.258819045102521,-0.965925826289068));
#54620=DIRECTION('',(0.,0.258819045102521,-0.965925826289068));
#54621=DIRECTION('',(1.,0.,0.));
#54622=DIRECTION('center_axis',(0.,0.258819045102521,-0.965925826289068));
#54623=DIRECTION('ref_axis',(0.,0.965925826289068,0.258819045102521));
#54624=DIRECTION('',(0.,0.965925826289068,0.258819045102521));
#54625=DIRECTION('center_axis',(1.,0.,0.));
#54626=DIRECTION('ref_axis',(0.,0.258819045102521,-0.965925826289068));
#54627=DIRECTION('center_axis',(1.,0.,0.));
#54628=DIRECTION('ref_axis',(0.,1.,0.));
#54629=DIRECTION('center_axis',(0.,0.,1.));
#54630=DIRECTION('ref_axis',(0.,-1.,0.));
#54631=DIRECTION('',(0.,-1.,0.));
#54632=DIRECTION('',(1.,0.,0.));
#54633=DIRECTION('center_axis',(0.,-1.,0.));
#54634=DIRECTION('ref_axis',(0.,0.,-1.));
#54635=DIRECTION('',(0.,0.,-1.));
#54636=DIRECTION('',(1.,0.,0.));
#54637=DIRECTION('center_axis',(0.,0.,-1.));
#54638=DIRECTION('ref_axis',(0.,1.,0.));
#54639=DIRECTION('',(0.,1.,0.));
#54640=DIRECTION('center_axis',(1.,0.,0.));
#54641=DIRECTION('ref_axis',(0.,0.,-1.));
#54642=DIRECTION('center_axis',(1.,0.,0.));
#54643=DIRECTION('ref_axis',(0.,0.,-1.));
#83021=CARTESIAN_POINT('',(0.,0.,0.));
#83022=CARTESIAN_POINT('Origin',(516.,12.2681871124402,-2.51079369406472));
#83023=CARTESIAN_POINT('',(536.,10.8192983730066,-2.12256512641094));
#83024=CARTESIAN_POINT('',(536.,11.1818124546495,-2.21970048183205));
#83025=CARTESIAN_POINT('',(536.,6.23115069813357,-0.893174662173959));
#83026=CARTESIAN_POINT('',(516.,10.8192983730066,-2.12256512641094));
#83027=CARTESIAN_POINT('',(516.,10.8192983730066,-2.12256512641094));
#83028=CARTESIAN_POINT('',(516.,11.7625631611684,-2.37531216464761));
#83029=CARTESIAN_POINT('',(516.,12.2681871124402,-2.51079369406472));
#83030=CARTESIAN_POINT('',(535.4,11.7625631611684,-2.37531216464761));
#83031=CARTESIAN_POINT('',(338.,11.7625631611684,-2.37531216464761));
#83032=CARTESIAN_POINT('Ctrl Pts',(536.,11.1818124546495,-2.21970048183205));
#83033=CARTESIAN_POINT('Ctrl Pts',(535.707724069012,11.4647422849793,-2.29551130138361));
#83034=CARTESIAN_POINT('Ctrl Pts',(535.4,11.7625631611684,-2.37531216464761));
#83035=CARTESIAN_POINT('Origin',(516.,11.3496284588966,-3.04112377995463));
#83036=CARTESIAN_POINT('',(516.,11.3743345935147,-3.82420090408121));
#83037=CARTESIAN_POINT('Origin',(516.,0.,0.));
#83038=CARTESIAN_POINT('',(516.,10.4310698053529,-3.57145386584454));
#83039=CARTESIAN_POINT('',(516.,10.8192983730066,-2.12256512641094));
#83040=CARTESIAN_POINT('',(516.,10.4310698053529,-3.57145386584454));
#83041=CARTESIAN_POINT('Origin',(516.,10.4310698053529,-3.57145386584454));
#83042=CARTESIAN_POINT('',(536.,10.7935838869957,-3.66858922126565));
#83043=CARTESIAN_POINT('',(536.,10.4310698053529,-3.57145386584454));
#83044=CARTESIAN_POINT('',(536.,5.11847776076298,-2.14794911778067));
#83045=CARTESIAN_POINT('',(535.4,11.3743345935147,-3.82420090408121));
#83046=CARTESIAN_POINT('Ctrl Pts',(535.4,11.3743345935147,-3.82420090408121));
#83047=CARTESIAN_POINT('Ctrl Pts',(535.707724073612,11.0765137128733,-3.74440003962422));
#83048=CARTESIAN_POINT('Ctrl Pts',(536.,10.7935838869957,-3.66858922126565));
#83049=CARTESIAN_POINT('',(338.,11.3743345935147,-3.82420090408121));
#83050=CARTESIAN_POINT('',(516.,10.4310698053529,-3.57145386584454));
#83051=CARTESIAN_POINT('Origin',(516.,10.8192983730066,-2.12256512641094));
#83052=CARTESIAN_POINT('',(536.,10.7222412310932,-2.48478731126934));
#83053=CARTESIAN_POINT('Origin',(338.,0.,0.));
#83054=CARTESIAN_POINT('',(535.4,10.7469875144545,-5.33875073066342));
#83055=CARTESIAN_POINT('Origin',(535.4,0.,0.));
#83056=CARTESIAN_POINT('',(516.,10.7469875144545,-5.33875073066342));
#83057=CARTESIAN_POINT('',(338.,10.7469875144545,-5.33875073066342));
#83058=CARTESIAN_POINT('',(516.,9.9969875144545,-6.63778883634007));
#83059=CARTESIAN_POINT('Origin',(516.,0.,0.));
#83060=CARTESIAN_POINT('',(535.4,9.9969875144545,-6.63778883634007));
#83061=CARTESIAN_POINT('',(338.,9.9969875144545,-6.63778883634007));
#83062=CARTESIAN_POINT('',(535.4,8.99902242886707,-7.93836225708725));
#83063=CARTESIAN_POINT('Origin',(535.4,0.,0.));
#83064=CARTESIAN_POINT('',(516.,8.99902242886707,-7.93836225708725));
#83065=CARTESIAN_POINT('',(338.,8.99902242886707,-7.93836225708725));
#83066=CARTESIAN_POINT('',(516.,7.93836225708725,-8.99902242886707));
#83067=CARTESIAN_POINT('Origin',(516.,0.,0.));
#83068=CARTESIAN_POINT('',(535.4,7.93836225708725,-8.99902242886707));
#83069=CARTESIAN_POINT('',(338.,7.93836225708725,-8.99902242886707));
#83070=CARTESIAN_POINT('',(535.4,6.63778883634006,-9.9969875144545));
#83071=CARTESIAN_POINT('Origin',(535.4,0.,0.));
#83072=CARTESIAN_POINT('',(516.,6.63778883634006,-9.9969875144545));
#83073=CARTESIAN_POINT('',(338.,6.63778883634006,-9.9969875144545));
#83074=CARTESIAN_POINT('',(516.,5.3387507306634,-10.7469875144545));
#83075=CARTESIAN_POINT('Origin',(516.,0.,0.));
#83076=CARTESIAN_POINT('',(535.4,5.3387507306634,-10.7469875144545));
#83077=CARTESIAN_POINT('',(338.,5.3387507306634,-10.7469875144545));
#83078=CARTESIAN_POINT('',(535.4,3.82420090408119,-11.3743345935147));
#83079=CARTESIAN_POINT('Origin',(535.4,0.,0.));
#83080=CARTESIAN_POINT('',(516.,3.82420090408119,-11.3743345935147));
#83081=CARTESIAN_POINT('',(338.,3.82420090408119,-11.3743345935147));
#83082=CARTESIAN_POINT('',(516.,2.37531216464759,-11.7625631611685));
#83083=CARTESIAN_POINT('Origin',(516.,0.,0.));
#83084=CARTESIAN_POINT('',(535.4,2.37531216464759,-11.7625631611685));
#83085=CARTESIAN_POINT('',(338.,2.37531216464759,-11.7625631611685));
#83086=CARTESIAN_POINT('',(535.4,0.749999999999998,-11.9765395670035));
#83087=CARTESIAN_POINT('Origin',(535.4,0.,0.));
#83088=CARTESIAN_POINT('',(516.,0.749999999999998,-11.9765395670035));
#83089=CARTESIAN_POINT('',(338.,0.749999999999998,-11.9765395670035));
#83090=CARTESIAN_POINT('',(516.,-0.750000000000002,-11.9765395670035));
#83091=CARTESIAN_POINT('Origin',(516.,0.,0.));
#83092=CARTESIAN_POINT('',(535.4,-0.750000000000002,-11.9765395670035));
#83093=CARTESIAN_POINT('',(338.,-0.750000000000002,-11.9765395670035));
#83094=CARTESIAN_POINT('',(535.4,-2.37531216464761,-11.7625631611684));
#83095=CARTESIAN_POINT('Origin',(535.4,0.,0.));
#83096=CARTESIAN_POINT('',(516.,-2.37531216464761,-11.7625631611684));
#83097=CARTESIAN_POINT('',(338.,-2.37531216464761,-11.7625631611684));
#83098=CARTESIAN_POINT('',(516.,-3.82420090408121,-11.3743345935147));
#83099=CARTESIAN_POINT('Origin',(516.,0.,0.));
#83100=CARTESIAN_POINT('',(535.4,-3.82420090408121,-11.3743345935147));
#83101=CARTESIAN_POINT('',(338.,-3.82420090408121,-11.3743345935147));
#83102=CARTESIAN_POINT('',(535.4,-5.33875073066342,-10.7469875144545));
#83103=CARTESIAN_POINT('Origin',(535.4,0.,0.));
#83104=CARTESIAN_POINT('',(516.,-5.33875073066342,-10.7469875144545));
#83105=CARTESIAN_POINT('',(338.,-5.33875073066342,-10.7469875144545));
#83106=CARTESIAN_POINT('',(516.,-6.63778883634007,-9.9969875144545));
#83107=CARTESIAN_POINT('Origin',(516.,0.,0.));
#83108=CARTESIAN_POINT('',(535.4,-6.63778883634007,-9.9969875144545));
#83109=CARTESIAN_POINT('',(338.,-6.63778883634007,-9.9969875144545));
#83110=CARTESIAN_POINT('',(535.4,-7.93836225708725,-8.99902242886707));
#83111=CARTESIAN_POINT('Origin',(535.4,0.,0.));
#83112=CARTESIAN_POINT('',(516.,-7.93836225708725,-8.99902242886707));
#83113=CARTESIAN_POINT('',(338.,-7.93836225708725,-8.99902242886707));
#83114=CARTESIAN_POINT('',(516.,-8.99902242886708,-7.93836225708725));
#83115=CARTESIAN_POINT('Origin',(516.,0.,0.));
#83116=CARTESIAN_POINT('',(535.4,-8.99902242886708,-7.93836225708725));
#83117=CARTESIAN_POINT('',(338.,-8.99902242886708,-7.93836225708725));
#83118=CARTESIAN_POINT('',(535.4,-9.9969875144545,-6.63778883634007));
#83119=CARTESIAN_POINT('Origin',(535.4,0.,0.));
#83120=CARTESIAN_POINT('',(516.,-9.9969875144545,-6.63778883634007));
#83121=CARTESIAN_POINT('',(338.,-9.9969875144545,-6.63778883634007));
#83122=CARTESIAN_POINT('',(516.,-10.7469875144545,-5.33875073066341));
#83123=CARTESIAN_POINT('Origin',(516.,0.,0.));
#83124=CARTESIAN_POINT('',(535.4,-10.7469875144545,-5.33875073066341));
#83125=CARTESIAN_POINT('',(338.,-10.7469875144545,-5.33875073066341));
#83126=CARTESIAN_POINT('',(535.4,-11.3743345935147,-3.82420090408119));
#83127=CARTESIAN_POINT('Origin',(535.4,0.,0.));
#83128=CARTESIAN_POINT('',(516.,-11.3743345935147,-3.82420090408119));
#83129=CARTESIAN_POINT('',(338.,-11.3743345935147,-3.82420090408119));
#83130=CARTESIAN_POINT('',(516.,-11.7625631611685,-2.37531216464759));
#83131=CARTESIAN_POINT('Origin',(516.,0.,0.));
#83132=CARTESIAN_POINT('',(535.4,-11.7625631611685,-2.37531216464759));
#83133=CARTESIAN_POINT('',(338.,-11.7625631611685,-2.37531216464759));
#83134=CARTESIAN_POINT('',(535.4,-11.9765395670035,-0.749999999999999));
#83135=CARTESIAN_POINT('Origin',(535.4,0.,0.));
#83136=CARTESIAN_POINT('',(516.,-11.9765395670035,-0.749999999999999));
#83137=CARTESIAN_POINT('',(338.,-11.9765395670035,-0.749999999999999));
#83138=CARTESIAN_POINT('',(516.,-12.,-1.46957615897682E-15));
#83139=CARTESIAN_POINT('Origin',(516.,0.,0.));
#83140=CARTESIAN_POINT('',(160.,-12.,-1.46957615897682E-15));
#83141=CARTESIAN_POINT('',(338.,-12.,-1.46957615897682E-15));
#83142=CARTESIAN_POINT('',(160.,-11.9765395670035,-0.749999999999999));
#83143=CARTESIAN_POINT('Origin',(160.,0.,0.));
#83144=CARTESIAN_POINT('',(140.6,-11.9765395670035,-0.749999999999999));
#83145=CARTESIAN_POINT('',(338.,-11.9765395670035,-0.749999999999999));
#83146=CARTESIAN_POINT('',(140.6,-11.7625631611685,-2.37531216464759));
#83147=CARTESIAN_POINT('Origin',(140.6,0.,0.));
#83148=CARTESIAN_POINT('',(160.,-11.7625631611685,-2.37531216464759));
#83149=CARTESIAN_POINT('',(338.,-11.7625631611685,-2.37531216464759));
#83150=CARTESIAN_POINT('',(160.,-11.3743345935147,-3.82420090408119));
#83151=CARTESIAN_POINT('Origin',(160.,0.,0.));
#83152=CARTESIAN_POINT('',(140.6,-11.3743345935147,-3.82420090408119));
#83153=CARTESIAN_POINT('',(338.,-11.3743345935147,-3.82420090408119));
#83154=CARTESIAN_POINT('',(140.6,-10.7469875144545,-5.33875073066341));
#83155=CARTESIAN_POINT('Origin',(140.6,0.,0.));
#83156=CARTESIAN_POINT('',(160.,-10.7469875144545,-5.33875073066341));
#83157=CARTESIAN_POINT('',(338.,-10.7469875144545,-5.33875073066341));
#83158=CARTESIAN_POINT('',(160.,-9.9969875144545,-6.63778883634007));
#83159=CARTESIAN_POINT('Origin',(160.,0.,0.));
#83160=CARTESIAN_POINT('',(140.6,-9.9969875144545,-6.63778883634007));
#83161=CARTESIAN_POINT('',(338.,-9.9969875144545,-6.63778883634007));
#83162=CARTESIAN_POINT('',(140.6,-8.99902242886708,-7.93836225708725));
#83163=CARTESIAN_POINT('Origin',(140.6,0.,0.));
#83164=CARTESIAN_POINT('',(160.,-8.99902242886708,-7.93836225708725));
#83165=CARTESIAN_POINT('',(338.,-8.99902242886708,-7.93836225708725));
#83166=CARTESIAN_POINT('',(160.,-7.93836225708725,-8.99902242886707));
#83167=CARTESIAN_POINT('Origin',(160.,0.,0.));
#83168=CARTESIAN_POINT('',(140.6,-7.93836225708725,-8.99902242886707));
#83169=CARTESIAN_POINT('',(338.,-7.93836225708725,-8.99902242886707));
#83170=CARTESIAN_POINT('',(140.6,-6.63778883634007,-9.9969875144545));
#83171=CARTESIAN_POINT('Origin',(140.6,0.,0.));
#83172=CARTESIAN_POINT('',(160.,-6.63778883634007,-9.9969875144545));
#83173=CARTESIAN_POINT('',(338.,-6.63778883634007,-9.9969875144545));
#83174=CARTESIAN_POINT('',(160.,-5.33875073066342,-10.7469875144545));
#83175=CARTESIAN_POINT('Origin',(160.,0.,0.));
#83176=CARTESIAN_POINT('',(140.6,-5.33875073066342,-10.7469875144545));
#83177=CARTESIAN_POINT('',(338.,-5.33875073066342,-10.7469875144545));
#83178=CARTESIAN_POINT('',(140.6,-3.82420090408121,-11.3743345935147));
#83179=CARTESIAN_POINT('Origin',(140.6,0.,0.));
#83180=CARTESIAN_POINT('',(160.,-3.82420090408121,-11.3743345935147));
#83181=CARTESIAN_POINT('',(338.,-3.82420090408121,-11.3743345935147));
#83182=CARTESIAN_POINT('',(160.,-2.37531216464761,-11.7625631611684));
#83183=CARTESIAN_POINT('Origin',(160.,0.,0.));
#83184=CARTESIAN_POINT('',(140.6,-2.37531216464761,-11.7625631611684));
#83185=CARTESIAN_POINT('',(338.,-2.37531216464761,-11.7625631611684));
#83186=CARTESIAN_POINT('',(140.6,-0.750000000000002,-11.9765395670035));
#83187=CARTESIAN_POINT('Origin',(140.6,0.,0.));
#83188=CARTESIAN_POINT('',(160.,-0.750000000000002,-11.9765395670035));
#83189=CARTESIAN_POINT('',(338.,-0.750000000000002,-11.9765395670035));
#83190=CARTESIAN_POINT('',(160.,0.749999999999998,-11.9765395670035));
#83191=CARTESIAN_POINT('Origin',(160.,0.,0.));
#83192=CARTESIAN_POINT('',(140.6,0.749999999999998,-11.9765395670035));
#83193=CARTESIAN_POINT('',(338.,0.749999999999998,-11.9765395670035));
#83194=CARTESIAN_POINT('',(140.6,2.37531216464759,-11.7625631611685));
#83195=CARTESIAN_POINT('Origin',(140.6,0.,0.));
#83196=CARTESIAN_POINT('',(160.,2.37531216464759,-11.7625631611685));
#83197=CARTESIAN_POINT('',(338.,2.37531216464759,-11.7625631611685));
#83198=CARTESIAN_POINT('',(160.,3.82420090408119,-11.3743345935147));
#83199=CARTESIAN_POINT('Origin',(160.,0.,0.));
#83200=CARTESIAN_POINT('',(140.6,3.82420090408119,-11.3743345935147));
#83201=CARTESIAN_POINT('',(338.,3.82420090408119,-11.3743345935147));
#83202=CARTESIAN_POINT('',(140.6,5.3387507306634,-10.7469875144545));
#83203=CARTESIAN_POINT('Origin',(140.6,0.,0.));
#83204=CARTESIAN_POINT('',(160.,5.3387507306634,-10.7469875144545));
#83205=CARTESIAN_POINT('',(338.,5.3387507306634,-10.7469875144545));
#83206=CARTESIAN_POINT('',(160.,6.63778883634006,-9.9969875144545));
#83207=CARTESIAN_POINT('Origin',(160.,0.,0.));
#83208=CARTESIAN_POINT('',(140.6,6.63778883634006,-9.9969875144545));
#83209=CARTESIAN_POINT('',(338.,6.63778883634006,-9.9969875144545));
#83210=CARTESIAN_POINT('',(140.6,7.93836225708725,-8.99902242886707));
#83211=CARTESIAN_POINT('Origin',(140.6,0.,0.));
#83212=CARTESIAN_POINT('',(160.,7.93836225708725,-8.99902242886707));
#83213=CARTESIAN_POINT('',(338.,7.93836225708725,-8.99902242886707));
#83214=CARTESIAN_POINT('',(160.,8.99902242886707,-7.93836225708725));
#83215=CARTESIAN_POINT('Origin',(160.,0.,0.));
#83216=CARTESIAN_POINT('',(140.6,8.99902242886707,-7.93836225708725));
#83217=CARTESIAN_POINT('',(338.,8.99902242886707,-7.93836225708725));
#83218=CARTESIAN_POINT('',(140.6,9.9969875144545,-6.63778883634007));
#83219=CARTESIAN_POINT('Origin',(140.6,0.,0.));
#83220=CARTESIAN_POINT('',(160.,9.9969875144545,-6.63778883634007));
#83221=CARTESIAN_POINT('',(338.,9.9969875144545,-6.63778883634007));
#83222=CARTESIAN_POINT('',(160.,10.7469875144545,-5.33875073066342));
#83223=CARTESIAN_POINT('Origin',(160.,0.,0.));
#83224=CARTESIAN_POINT('',(140.6,10.7469875144545,-5.33875073066342));
#83225=CARTESIAN_POINT('',(338.,10.7469875144545,-5.33875073066342));
#83226=CARTESIAN_POINT('',(140.6,11.3743345935147,-3.82420090408121));
#83227=CARTESIAN_POINT('Origin',(140.6,0.,0.));
#83228=CARTESIAN_POINT('',(160.,11.3743345935147,-3.82420090408121));
#83229=CARTESIAN_POINT('',(338.,11.3743345935147,-3.82420090408121));
#83230=CARTESIAN_POINT('',(160.,11.7625631611684,-2.37531216464761));
#83231=CARTESIAN_POINT('Origin',(160.,0.,0.));
#83232=CARTESIAN_POINT('',(140.6,11.7625631611684,-2.37531216464761));
#83233=CARTESIAN_POINT('',(338.,11.7625631611684,-2.37531216464761));
#83234=CARTESIAN_POINT('',(140.6,11.9765395670035,-0.75));
#83235=CARTESIAN_POINT('Origin',(140.6,0.,0.));
#83236=CARTESIAN_POINT('',(160.,11.9765395670035,-0.75));
#83237=CARTESIAN_POINT('',(338.,11.9765395670035,-0.75));
#83238=CARTESIAN_POINT('',(160.,11.9765395670035,0.75));
#83239=CARTESIAN_POINT('Origin',(160.,0.,0.));
#83240=CARTESIAN_POINT('',(140.6,11.9765395670035,0.75));
#83241=CARTESIAN_POINT('',(338.,11.9765395670035,0.75));
#83242=CARTESIAN_POINT('',(140.6,11.7625631611685,2.3753121646476));
#83243=CARTESIAN_POINT('Origin',(140.6,0.,0.));
#83244=CARTESIAN_POINT('',(160.,11.7625631611685,2.3753121646476));
#83245=CARTESIAN_POINT('',(338.,11.7625631611685,2.3753121646476));
#83246=CARTESIAN_POINT('',(160.,11.3743345935147,3.8242009040812));
#83247=CARTESIAN_POINT('Origin',(160.,0.,0.));
#83248=CARTESIAN_POINT('',(140.6,11.3743345935147,3.8242009040812));
#83249=CARTESIAN_POINT('',(338.,11.3743345935147,3.8242009040812));
#83250=CARTESIAN_POINT('',(140.6,10.7469875144545,5.33875073066341));
#83251=CARTESIAN_POINT('Origin',(140.6,0.,0.));
#83252=CARTESIAN_POINT('',(160.,10.7469875144545,5.33875073066341));
#83253=CARTESIAN_POINT('',(338.,10.7469875144545,5.33875073066341));
#83254=CARTESIAN_POINT('',(160.,9.9969875144545,6.63778883634007));
#83255=CARTESIAN_POINT('Origin',(160.,0.,0.));
#83256=CARTESIAN_POINT('',(140.6,9.9969875144545,6.63778883634007));
#83257=CARTESIAN_POINT('',(338.,9.9969875144545,6.63778883634007));
#83258=CARTESIAN_POINT('',(140.6,8.99902242886707,7.93836225708725));
#83259=CARTESIAN_POINT('Origin',(140.6,0.,0.));
#83260=CARTESIAN_POINT('',(160.,8.99902242886707,7.93836225708725));
#83261=CARTESIAN_POINT('',(338.,8.99902242886707,7.93836225708725));
#83262=CARTESIAN_POINT('',(160.,7.93836225708725,8.99902242886707));
#83263=CARTESIAN_POINT('Origin',(160.,0.,0.));
#83264=CARTESIAN_POINT('',(140.6,7.93836225708725,8.99902242886707));
#83265=CARTESIAN_POINT('',(338.,7.93836225708725,8.99902242886707));
#83266=CARTESIAN_POINT('',(140.6,6.63778883634007,9.9969875144545));
#83267=CARTESIAN_POINT('Origin',(140.6,0.,0.));
#83268=CARTESIAN_POINT('',(160.,6.63778883634007,9.9969875144545));
#83269=CARTESIAN_POINT('',(338.,6.63778883634007,9.9969875144545));
#83270=CARTESIAN_POINT('',(160.,5.33875073066341,10.7469875144545));
#83271=CARTESIAN_POINT('Origin',(160.,0.,0.));
#83272=CARTESIAN_POINT('',(140.6,5.33875073066341,10.7469875144545));
#83273=CARTESIAN_POINT('',(338.,5.33875073066341,10.7469875144545));
#83274=CARTESIAN_POINT('',(140.6,3.8242009040812,11.3743345935147));
#83275=CARTESIAN_POINT('Origin',(140.6,0.,0.));
#83276=CARTESIAN_POINT('',(160.,3.8242009040812,11.3743345935147));
#83277=CARTESIAN_POINT('',(338.,3.8242009040812,11.3743345935147));
#83278=CARTESIAN_POINT('',(160.,2.3753121646476,11.7625631611685));
#83279=CARTESIAN_POINT('Origin',(160.,0.,0.));
#83280=CARTESIAN_POINT('',(140.6,2.3753121646476,11.7625631611685));
#83281=CARTESIAN_POINT('',(338.,2.3753121646476,11.7625631611685));
#83282=CARTESIAN_POINT('',(140.6,0.750000000000001,11.9765395670035));
#83283=CARTESIAN_POINT('Origin',(140.6,0.,0.));
#83284=CARTESIAN_POINT('',(160.,0.750000000000001,11.9765395670035));
#83285=CARTESIAN_POINT('',(338.,0.750000000000001,11.9765395670035));
#83286=CARTESIAN_POINT('',(160.,-0.749999999999999,11.9765395670035));
#83287=CARTESIAN_POINT('Origin',(160.,0.,0.));
#83288=CARTESIAN_POINT('',(140.6,-0.749999999999999,11.9765395670035));
#83289=CARTESIAN_POINT('',(338.,-0.749999999999999,11.9765395670035));
#83290=CARTESIAN_POINT('',(140.6,-2.3753121646476,11.7625631611685));
#83291=CARTESIAN_POINT('Origin',(140.6,0.,0.));
#83292=CARTESIAN_POINT('',(160.,-2.3753121646476,11.7625631611685));
#83293=CARTESIAN_POINT('',(338.,-2.3753121646476,11.7625631611685));
#83294=CARTESIAN_POINT('',(160.,-3.8242009040812,11.3743345935147));
#83295=CARTESIAN_POINT('Origin',(160.,0.,0.));
#83296=CARTESIAN_POINT('',(140.6,-3.8242009040812,11.3743345935147));
#83297=CARTESIAN_POINT('',(338.,-3.8242009040812,11.3743345935147));
#83298=CARTESIAN_POINT('',(140.6,-5.33875073066341,10.7469875144545));
#83299=CARTESIAN_POINT('Origin',(140.6,0.,0.));
#83300=CARTESIAN_POINT('',(160.,-5.33875073066341,10.7469875144545));
#83301=CARTESIAN_POINT('',(338.,-5.33875073066341,10.7469875144545));
#83302=CARTESIAN_POINT('',(160.,-6.63778883634007,9.9969875144545));
#83303=CARTESIAN_POINT('Origin',(160.,0.,0.));
#83304=CARTESIAN_POINT('',(140.6,-6.63778883634007,9.9969875144545));
#83305=CARTESIAN_POINT('',(338.,-6.63778883634007,9.9969875144545));
#83306=CARTESIAN_POINT('',(140.6,-7.93836225708725,8.99902242886707));
#83307=CARTESIAN_POINT('Origin',(140.6,0.,0.));
#83308=CARTESIAN_POINT('',(160.,-7.93836225708725,8.99902242886707));
#83309=CARTESIAN_POINT('',(338.,-7.93836225708725,8.99902242886707));
#83310=CARTESIAN_POINT('',(160.,-8.99902242886707,7.93836225708725));
#83311=CARTESIAN_POINT('Origin',(160.,0.,0.));
#83312=CARTESIAN_POINT('',(140.6,-8.99902242886707,7.93836225708725));
#83313=CARTESIAN_POINT('',(338.,-8.99902242886707,7.93836225708725));
#83314=CARTESIAN_POINT('',(140.6,-9.99698751445449,6.63778883634007));
#83315=CARTESIAN_POINT('Origin',(140.6,0.,0.));
#83316=CARTESIAN_POINT('',(160.,-9.99698751445449,6.63778883634007));
#83317=CARTESIAN_POINT('',(338.,-9.99698751445449,6.63778883634007));
#83318=CARTESIAN_POINT('',(160.,-10.7469875144545,5.33875073066342));
#83319=CARTESIAN_POINT('Origin',(160.,0.,0.));
#83320=CARTESIAN_POINT('',(140.6,-10.7469875144545,5.33875073066342));
#83321=CARTESIAN_POINT('',(338.,-10.7469875144545,5.33875073066342));
#83322=CARTESIAN_POINT('',(140.6,-11.3743345935147,3.8242009040812));
#83323=CARTESIAN_POINT('Origin',(140.6,0.,0.));
#83324=CARTESIAN_POINT('',(160.,-11.3743345935147,3.8242009040812));
#83325=CARTESIAN_POINT('',(338.,-11.3743345935147,3.8242009040812));
#83326=CARTESIAN_POINT('',(160.,-11.7625631611685,2.3753121646476));
#83327=CARTESIAN_POINT('Origin',(160.,0.,0.));
#83328=CARTESIAN_POINT('',(140.6,-11.7625631611685,2.3753121646476));
#83329=CARTESIAN_POINT('',(338.,-11.7625631611685,2.3753121646476));
#83330=CARTESIAN_POINT('',(140.6,-11.9765395670035,0.750000000000002));
#83331=CARTESIAN_POINT('Origin',(140.6,0.,0.));
#83332=CARTESIAN_POINT('',(160.,-11.9765395670035,0.750000000000002));
#83333=CARTESIAN_POINT('',(338.,-11.9765395670035,0.750000000000002));
#83334=CARTESIAN_POINT('Origin',(160.,0.,0.));
#83335=CARTESIAN_POINT('',(516.,-11.9765395670035,0.750000000000002));
#83336=CARTESIAN_POINT('Origin',(516.,0.,0.));
#83337=CARTESIAN_POINT('',(535.4,-11.9765395670035,0.750000000000002));
#83338=CARTESIAN_POINT('',(338.,-11.9765395670035,0.750000000000002));
#83339=CARTESIAN_POINT('',(535.4,-11.7625631611685,2.3753121646476));
#83340=CARTESIAN_POINT('Origin',(535.4,0.,0.));
#83341=CARTESIAN_POINT('',(516.,-11.7625631611685,2.3753121646476));
#83342=CARTESIAN_POINT('',(338.,-11.7625631611685,2.3753121646476));
#83343=CARTESIAN_POINT('',(516.,-11.3743345935147,3.8242009040812));
#83344=CARTESIAN_POINT('Origin',(516.,0.,0.));
#83345=CARTESIAN_POINT('',(535.4,-11.3743345935147,3.8242009040812));
#83346=CARTESIAN_POINT('',(338.,-11.3743345935147,3.8242009040812));
#83347=CARTESIAN_POINT('',(535.4,-10.7469875144545,5.33875073066342));
#83348=CARTESIAN_POINT('Origin',(535.4,0.,0.));
#83349=CARTESIAN_POINT('',(516.,-10.7469875144545,5.33875073066342));
#83350=CARTESIAN_POINT('',(338.,-10.7469875144545,5.33875073066342));
#83351=CARTESIAN_POINT('',(516.,-9.99698751445449,6.63778883634007));
#83352=CARTESIAN_POINT('Origin',(516.,0.,0.));
#83353=CARTESIAN_POINT('',(535.4,-9.99698751445449,6.63778883634007));
#83354=CARTESIAN_POINT('',(338.,-9.99698751445449,6.63778883634007));
#83355=CARTESIAN_POINT('',(535.4,-8.99902242886707,7.93836225708725));
#83356=CARTESIAN_POINT('Origin',(535.4,0.,0.));
#83357=CARTESIAN_POINT('',(516.,-8.99902242886707,7.93836225708725));
#83358=CARTESIAN_POINT('',(338.,-8.99902242886707,7.93836225708725));
#83359=CARTESIAN_POINT('',(516.,-7.93836225708725,8.99902242886707));
#83360=CARTESIAN_POINT('Origin',(516.,0.,0.));
#83361=CARTESIAN_POINT('',(535.4,-7.93836225708725,8.99902242886707));
#83362=CARTESIAN_POINT('',(338.,-7.93836225708725,8.99902242886707));
#83363=CARTESIAN_POINT('',(535.4,-6.63778883634007,9.9969875144545));
#83364=CARTESIAN_POINT('Origin',(535.4,0.,0.));
#83365=CARTESIAN_POINT('',(516.,-6.63778883634007,9.9969875144545));
#83366=CARTESIAN_POINT('',(338.,-6.63778883634007,9.9969875144545));
#83367=CARTESIAN_POINT('',(516.,-5.33875073066341,10.7469875144545));
#83368=CARTESIAN_POINT('Origin',(516.,0.,0.));
#83369=CARTESIAN_POINT('',(535.4,-5.33875073066341,10.7469875144545));
#83370=CARTESIAN_POINT('',(338.,-5.33875073066341,10.7469875144545));
#83371=CARTESIAN_POINT('',(535.4,-3.8242009040812,11.3743345935147));
#83372=CARTESIAN_POINT('Origin',(535.4,0.,0.));
#83373=CARTESIAN_POINT('',(516.,-3.8242009040812,11.3743345935147));
#83374=CARTESIAN_POINT('',(338.,-3.8242009040812,11.3743345935147));
#83375=CARTESIAN_POINT('',(516.,-2.3753121646476,11.7625631611685));
#83376=CARTESIAN_POINT('Origin',(516.,0.,0.));
#83377=CARTESIAN_POINT('',(535.4,-2.3753121646476,11.7625631611685));
#83378=CARTESIAN_POINT('',(338.,-2.3753121646476,11.7625631611685));
#83379=CARTESIAN_POINT('',(535.4,-0.749999999999999,11.9765395670035));
#83380=CARTESIAN_POINT('Origin',(535.4,0.,0.));
#83381=CARTESIAN_POINT('',(516.,-0.749999999999999,11.9765395670035));
#83382=CARTESIAN_POINT('',(338.,-0.749999999999999,11.9765395670035));
#83383=CARTESIAN_POINT('',(516.,0.750000000000001,11.9765395670035));
#83384=CARTESIAN_POINT('Origin',(516.,0.,0.));
#83385=CARTESIAN_POINT('',(535.4,0.750000000000001,11.9765395670035));
#83386=CARTESIAN_POINT('',(338.,0.750000000000001,11.9765395670035));
#83387=CARTESIAN_POINT('',(535.4,2.3753121646476,11.7625631611685));
#83388=CARTESIAN_POINT('Origin',(535.4,0.,0.));
#83389=CARTESIAN_POINT('',(516.,2.3753121646476,11.7625631611685));
#83390=CARTESIAN_POINT('',(338.,2.3753121646476,11.7625631611685));
#83391=CARTESIAN_POINT('',(516.,3.8242009040812,11.3743345935147));
#83392=CARTESIAN_POINT('Origin',(516.,0.,0.));
#83393=CARTESIAN_POINT('',(535.4,3.8242009040812,11.3743345935147));
#83394=CARTESIAN_POINT('',(338.,3.8242009040812,11.3743345935147));
#83395=CARTESIAN_POINT('',(535.4,5.33875073066341,10.7469875144545));
#83396=CARTESIAN_POINT('Origin',(535.4,0.,0.));
#83397=CARTESIAN_POINT('',(516.,5.33875073066341,10.7469875144545));
#83398=CARTESIAN_POINT('',(338.,5.33875073066341,10.7469875144545));
#83399=CARTESIAN_POINT('',(516.,6.63778883634007,9.9969875144545));
#83400=CARTESIAN_POINT('Origin',(516.,0.,0.));
#83401=CARTESIAN_POINT('',(535.4,6.63778883634007,9.9969875144545));
#83402=CARTESIAN_POINT('',(338.,6.63778883634007,9.9969875144545));
#83403=CARTESIAN_POINT('',(535.4,7.93836225708725,8.99902242886707));
#83404=CARTESIAN_POINT('Origin',(535.4,0.,0.));
#83405=CARTESIAN_POINT('',(516.,7.93836225708725,8.99902242886707));
#83406=CARTESIAN_POINT('',(338.,7.93836225708725,8.99902242886707));
#83407=CARTESIAN_POINT('',(516.,8.99902242886707,7.93836225708725));
#83408=CARTESIAN_POINT('Origin',(516.,0.,0.));
#83409=CARTESIAN_POINT('',(535.4,8.99902242886707,7.93836225708725));
#83410=CARTESIAN_POINT('',(338.,8.99902242886707,7.93836225708725));
#83411=CARTESIAN_POINT('',(535.4,9.9969875144545,6.63778883634007));
#83412=CARTESIAN_POINT('Origin',(535.4,0.,0.));
#83413=CARTESIAN_POINT('',(516.,9.9969875144545,6.63778883634007));
#83414=CARTESIAN_POINT('',(338.,9.9969875144545,6.63778883634007));
#83415=CARTESIAN_POINT('',(516.,10.7469875144545,5.33875073066341));
#83416=CARTESIAN_POINT('Origin',(516.,0.,0.));
#83417=CARTESIAN_POINT('',(535.4,10.7469875144545,5.33875073066341));
#83418=CARTESIAN_POINT('',(338.,10.7469875144545,5.33875073066341));
#83419=CARTESIAN_POINT('',(535.4,11.3743345935147,3.8242009040812));
#83420=CARTESIAN_POINT('Origin',(535.4,0.,0.));
#83421=CARTESIAN_POINT('',(516.,11.3743345935147,3.8242009040812));
#83422=CARTESIAN_POINT('',(338.,11.3743345935147,3.8242009040812));
#83423=CARTESIAN_POINT('',(516.,11.7625631611685,2.3753121646476));
#83424=CARTESIAN_POINT('Origin',(516.,0.,0.));
#83425=CARTESIAN_POINT('',(535.4,11.7625631611685,2.3753121646476));
#83426=CARTESIAN_POINT('',(338.,11.7625631611685,2.3753121646476));
#83427=CARTESIAN_POINT('',(535.4,11.9765395670035,0.75));
#83428=CARTESIAN_POINT('Origin',(535.4,0.,0.));
#83429=CARTESIAN_POINT('',(516.,11.9765395670035,0.75));
#83430=CARTESIAN_POINT('',(338.,11.9765395670035,0.75));
#83431=CARTESIAN_POINT('',(516.,11.9765395670035,-0.75));
#83432=CARTESIAN_POINT('Origin',(516.,0.,0.));
#83433=CARTESIAN_POINT('',(535.4,11.9765395670035,-0.75));
#83434=CARTESIAN_POINT('',(338.,11.9765395670035,-0.75));
#83435=CARTESIAN_POINT('Origin',(535.4,0.,0.));
#83436=CARTESIAN_POINT('Origin',(535.7,0.,0.));
#83437=CARTESIAN_POINT('',(536.,10.2263006755453,-5.03813204405572));
#83438=CARTESIAN_POINT('Origin',(536.,0.,0.));
#83439=CARTESIAN_POINT('Ctrl Pts',(536.,10.2263006755453,-5.03813204405572));
#83440=CARTESIAN_POINT('Ctrl Pts',(535.707724072371,10.4799686188494,-5.18458729940711));
#83441=CARTESIAN_POINT('Ctrl Pts',(535.4,10.7469875144545,-5.33875073066342));
#83442=CARTESIAN_POINT('Origin',(535.7,0.,0.));
#83443=CARTESIAN_POINT('',(536.,11.3753021937881,-0.75));
#83444=CARTESIAN_POINT('Ctrl Pts',(535.4,11.9765395670035,-0.75));
#83445=CARTESIAN_POINT('Ctrl Pts',(535.707724067994,11.668212708876,-0.75));
#83446=CARTESIAN_POINT('Ctrl Pts',(536.,11.3753021937881,-0.75));
#83447=CARTESIAN_POINT('Origin',(536.,0.,0.));
#83448=CARTESIAN_POINT('Origin',(516.,11.2003175473055,-5.60048094716168));
#83449=CARTESIAN_POINT('',(536.,9.90127944162882,-4.85048094716168));
#83450=CARTESIAN_POINT('',(536.,5.78765877365274,-2.47548094716167));
#83451=CARTESIAN_POINT('',(516.,9.90127944162882,-4.85048094716168));
#83452=CARTESIAN_POINT('',(516.,9.90127944162882,-4.85048094716168));
#83453=CARTESIAN_POINT('',(516.,11.2003175473055,-5.60048094716168));
#83454=CARTESIAN_POINT('Origin',(516.,10.1757984944672,-5.87500000000001));
#83455=CARTESIAN_POINT('',(516.,9.15127944162882,-6.14951905283833));
#83456=CARTESIAN_POINT('',(516.,9.90127944162882,-4.85048094716168));
#83457=CARTESIAN_POINT('',(516.,9.15127944162882,-6.14951905283833));
#83458=CARTESIAN_POINT('Origin',(516.,9.15127944162882,-6.14951905283833));
#83459=CARTESIAN_POINT('',(536.,9.47630067554534,-6.33717014973238));
#83460=CARTESIAN_POINT('',(536.,9.15127944162882,-6.14951905283833));
#83461=CARTESIAN_POINT('',(536.,4.38813972081441,-3.39951905283833));
#83462=CARTESIAN_POINT('Ctrl Pts',(535.4,9.99698751445449,-6.63778883634008));
#83463=CARTESIAN_POINT('Ctrl Pts',(535.707724068139,9.72996862252186,-6.48362540720405));
#83464=CARTESIAN_POINT('Ctrl Pts',(536.,9.47630067554533,-6.33717014973238));
#83465=CARTESIAN_POINT('',(516.,9.15127944162882,-6.14951905283833));
#83466=CARTESIAN_POINT('Origin',(516.,9.90127944162882,-4.85048094716168));
#83467=CARTESIAN_POINT('',(536.,9.71377944162882,-5.17524047358084));
#83468=CARTESIAN_POINT('Origin',(535.7,0.,0.));
#83469=CARTESIAN_POINT('',(536.,8.57388340516368,-7.51322323338386));
#83470=CARTESIAN_POINT('Origin',(536.,0.,0.));
#83471=CARTESIAN_POINT('Ctrl Pts',(536.,8.57388340516367,-7.51322323338386));
#83472=CARTESIAN_POINT('Ctrl Pts',(535.707724069364,8.78100241569271,-7.7203422439129));
#83473=CARTESIAN_POINT('Ctrl Pts',(535.4,8.99902242886707,-7.93836225708725));
#83474=CARTESIAN_POINT('Origin',(516.,9.36916485072175,-8.30850467894194));
#83475=CARTESIAN_POINT('',(536.,8.30850467894193,-7.24784450716211));
#83476=CARTESIAN_POINT('',(536.,4.94974746830583,-3.88908729652601));
#83477=CARTESIAN_POINT('',(516.,8.30850467894193,-7.24784450716211));
#83478=CARTESIAN_POINT('',(516.,8.30850467894193,-7.24784450716211));
#83479=CARTESIAN_POINT('',(516.,9.36916485072175,-8.30850467894194));
#83480=CARTESIAN_POINT('Origin',(516.,8.30850467894193,-8.30850467894194));
#83481=CARTESIAN_POINT('',(516.,7.24784450716211,-8.30850467894194));
#83482=CARTESIAN_POINT('',(516.,8.30850467894193,-7.24784450716211));
#83483=CARTESIAN_POINT('',(516.,7.24784450716211,-8.30850467894194));
#83484=CARTESIAN_POINT('Origin',(516.,7.24784450716211,-8.30850467894194));
#83485=CARTESIAN_POINT('',(536.,7.51322323338385,-8.57388340516368));
#83486=CARTESIAN_POINT('',(536.,7.24784450716211,-8.30850467894194));
#83487=CARTESIAN_POINT('',(536.,3.3587572106361,-4.41941738241592));
#83488=CARTESIAN_POINT('Ctrl Pts',(535.4,7.93836225708725,-8.99902242886707));
#83489=CARTESIAN_POINT('Ctrl Pts',(535.707724065172,7.72034224688363,-8.78100241866346));
#83490=CARTESIAN_POINT('Ctrl Pts',(536.,7.51322323338385,-8.57388340516368));
#83491=CARTESIAN_POINT('',(516.,7.24784450716211,-8.30850467894194));
#83492=CARTESIAN_POINT('Origin',(516.,8.30850467894193,-7.24784450716211));
#83493=CARTESIAN_POINT('',(536.,8.04333963599698,-7.51300955010707));
#83494=CARTESIAN_POINT('Origin',(535.7,0.,0.));
#83495=CARTESIAN_POINT('',(536.,6.33717014973236,-9.47630067554534));
#83496=CARTESIAN_POINT('Origin',(536.,0.,0.));
#83497=CARTESIAN_POINT('Ctrl Pts',(536.,6.33717014973236,-9.47630067554534));
#83498=CARTESIAN_POINT('Ctrl Pts',(535.707724067523,6.48362540751262,-9.72996862305635));
#83499=CARTESIAN_POINT('Ctrl Pts',(535.4,6.63778883634006,-9.9969875144545));
#83500=CARTESIAN_POINT('Origin',(516.,6.89951905283832,-10.4503175473055));
#83501=CARTESIAN_POINT('',(536.,6.14951905283832,-9.15127944162883));
#83502=CARTESIAN_POINT('',(536.,3.77451905283832,-5.03765877365275));
#83503=CARTESIAN_POINT('',(516.,6.14951905283832,-9.15127944162883));
#83504=CARTESIAN_POINT('',(516.,6.14951905283832,-9.15127944162883));
#83505=CARTESIAN_POINT('',(516.,6.89951905283832,-10.4503175473055));
#83506=CARTESIAN_POINT('Origin',(516.,5.87499999999999,-10.1757984944672));
#83507=CARTESIAN_POINT('',(516.,4.85048094716166,-9.90127944162883));
#83508=CARTESIAN_POINT('',(516.,6.14951905283832,-9.15127944162883));
#83509=CARTESIAN_POINT('',(516.,4.85048094716166,-9.90127944162883));
#83510=CARTESIAN_POINT('Origin',(516.,4.85048094716166,-9.90127944162883));
#83511=CARTESIAN_POINT('',(536.,5.03813204405571,-10.2263006755453));
#83512=CARTESIAN_POINT('',(536.,4.85048094716166,-9.90127944162883));
#83513=CARTESIAN_POINT('',(536.,2.10048094716167,-5.13813972081441));
#83514=CARTESIAN_POINT('Ctrl Pts',(535.4,5.3387507306634,-10.7469875144545));
#83515=CARTESIAN_POINT('Ctrl Pts',(535.707724067538,5.18458730182822,-10.4799686230429));
#83516=CARTESIAN_POINT('Ctrl Pts',(536.,5.03813204405571,-10.2263006755453));
#83517=CARTESIAN_POINT('',(516.,4.85048094716166,-9.90127944162883));
#83518=CARTESIAN_POINT('Origin',(516.,6.14951905283832,-9.15127944162883));
#83519=CARTESIAN_POINT('',(536.,5.82475952641916,-9.33877944162883));
#83520=CARTESIAN_POINT('Origin',(535.7,0.,0.));
#83521=CARTESIAN_POINT('',(536.,3.66858922126564,-10.7935838869957));
#83522=CARTESIAN_POINT('Origin',(536.,0.,0.));
#83523=CARTESIAN_POINT('Ctrl Pts',(536.,3.66858922126564,-10.7935838869957));
#83524=CARTESIAN_POINT('Ctrl Pts',(535.707724073367,3.74440003968782,-11.0765137131107));
#83525=CARTESIAN_POINT('Ctrl Pts',(535.4,3.82420090408119,-11.3743345935147));
#83526=CARTESIAN_POINT('Origin',(516.,3.9596824334983,-11.8799585447865));
#83527=CARTESIAN_POINT('',(536.,3.57145386584452,-10.4310698053529));
#83528=CARTESIAN_POINT('',(536.,2.34206340160755,-5.84292213047979));
#83529=CARTESIAN_POINT('',(516.,3.57145386584452,-10.4310698053529));
#83530=CARTESIAN_POINT('',(516.,3.57145386584452,-10.4310698053529));
#83531=CARTESIAN_POINT('',(516.,3.9596824334983,-11.8799585447865));
#83532=CARTESIAN_POINT('Origin',(516.,3.04112377995461,-11.3496284588966));
#83533=CARTESIAN_POINT('',(516.,2.12256512641092,-10.8192983730066));
#83534=CARTESIAN_POINT('',(516.,3.57145386584452,-10.4310698053529));
#83535=CARTESIAN_POINT('',(516.,2.12256512641092,-10.8192983730066));
#83536=CARTESIAN_POINT('Origin',(516.,2.12256512641092,-10.8192983730066));
#83537=CARTESIAN_POINT('',(536.,2.21970048183204,-11.1818124546495));
#83538=CARTESIAN_POINT('',(536.,2.12256512641092,-10.8192983730066));
#83539=CARTESIAN_POINT('',(536.,0.699060378347061,-5.50670632841677));
#83540=CARTESIAN_POINT('Ctrl Pts',(535.4,2.37531216464759,-11.7625631611685));
#83541=CARTESIAN_POINT('Ctrl Pts',(535.707724065234,2.29551130236342,-11.4647422886361));
#83542=CARTESIAN_POINT('Ctrl Pts',(536.,2.21970048183203,-11.1818124546495));
#83543=CARTESIAN_POINT('',(516.,2.12256512641092,-10.8192983730066));
#83544=CARTESIAN_POINT('Origin',(516.,3.57145386584452,-10.4310698053529));
#83545=CARTESIAN_POINT('',(536.,3.20923168098612,-10.5281269472663));
#83546=CARTESIAN_POINT('Origin',(535.7,0.,0.));
#83547=CARTESIAN_POINT('',(536.,0.749999999999998,-11.3753021937881));
#83548=CARTESIAN_POINT('Origin',(536.,0.,0.));
#83549=CARTESIAN_POINT('Ctrl Pts',(536.,0.749999999999998,-11.3753021937881));
#83550=CARTESIAN_POINT('Ctrl Pts',(535.707724072196,0.749999999999998,-11.6682127046657));
#83551=CARTESIAN_POINT('Ctrl Pts',(535.4,0.749999999999998,-11.9765395670035));
#83552=CARTESIAN_POINT('Origin',(516.,0.749999999999998,-12.5));
#83553=CARTESIAN_POINT('',(536.,0.749999999999998,-11.));
#83554=CARTESIAN_POINT('',(536.,0.749999999999999,-6.25));
#83555=CARTESIAN_POINT('',(516.,0.749999999999998,-11.));
#83556=CARTESIAN_POINT('',(516.,0.749999999999998,-11.));
#83557=CARTESIAN_POINT('',(516.,0.749999999999998,-12.5));
#83558=CARTESIAN_POINT('Origin',(516.,-2.15843998349721E-15,-11.75));
#83559=CARTESIAN_POINT('',(516.,-0.750000000000002,-11.));
#83560=CARTESIAN_POINT('',(516.,0.749999999999998,-11.));
#83561=CARTESIAN_POINT('',(516.,-0.750000000000002,-11.));
#83562=CARTESIAN_POINT('Origin',(516.,-0.750000000000002,-11.));
#83563=CARTESIAN_POINT('',(536.,-0.750000000000002,-11.3753021937881));
#83564=CARTESIAN_POINT('',(536.,-0.750000000000002,-11.));
#83565=CARTESIAN_POINT('',(536.,-0.750000000000001,-5.5));
#83566=CARTESIAN_POINT('Ctrl Pts',(535.4,-0.750000000000002,-11.9765395670035));
#83567=CARTESIAN_POINT('Ctrl Pts',(535.707724072196,-0.750000000000002,
-11.6682127046657));
#83568=CARTESIAN_POINT('Ctrl Pts',(536.,-0.750000000000002,-11.3753021937881));
#83569=CARTESIAN_POINT('',(516.,-0.750000000000002,-11.));
#83570=CARTESIAN_POINT('Origin',(516.,0.749999999999998,-11.));
#83571=CARTESIAN_POINT('',(536.,0.374999999999998,-11.));
#83572=CARTESIAN_POINT('Origin',(535.7,0.,0.));
#83573=CARTESIAN_POINT('',(536.,-2.21970048183205,-11.1818124546495));
#83574=CARTESIAN_POINT('Origin',(536.,0.,0.));
#83575=CARTESIAN_POINT('Ctrl Pts',(536.,-2.21970048183205,-11.1818124546495));
#83576=CARTESIAN_POINT('Ctrl Pts',(535.707724069012,-2.29551130138365,-11.4647422849795));
#83577=CARTESIAN_POINT('Ctrl Pts',(535.4,-2.37531216464761,-11.7625631611684));
#83578=CARTESIAN_POINT('Origin',(516.,-2.51079369406472,-12.2681871124402));
#83579=CARTESIAN_POINT('',(536.,-2.12256512641094,-10.8192983730066));
#83580=CARTESIAN_POINT('',(536.,-0.893174662173959,-6.23115069813357));
#83581=CARTESIAN_POINT('',(516.,-2.12256512641094,-10.8192983730066));
#83582=CARTESIAN_POINT('',(516.,-2.12256512641094,-10.8192983730066));
#83583=CARTESIAN_POINT('',(516.,-2.51079369406472,-12.2681871124402));
#83584=CARTESIAN_POINT('Origin',(516.,-3.04112377995463,-11.3496284588966));
#83585=CARTESIAN_POINT('',(516.,-3.57145386584454,-10.4310698053529));
#83586=CARTESIAN_POINT('',(516.,-2.12256512641094,-10.8192983730066));
#83587=CARTESIAN_POINT('',(516.,-3.57145386584454,-10.4310698053529));
#83588=CARTESIAN_POINT('Origin',(516.,-3.57145386584454,-10.4310698053529));
#83589=CARTESIAN_POINT('',(536.,-3.66858922126565,-10.7935838869957));
#83590=CARTESIAN_POINT('',(536.,-3.57145386584454,-10.4310698053529));
#83591=CARTESIAN_POINT('',(536.,-2.14794911778067,-5.11847776076298));
#83592=CARTESIAN_POINT('Ctrl Pts',(535.4,-3.82420090408121,-11.3743345935147));
#83593=CARTESIAN_POINT('Ctrl Pts',(535.707724069553,-3.7444000406769,-11.0765137168019));
#83594=CARTESIAN_POINT('Ctrl Pts',(536.,-3.66858922126565,-10.7935838869957));
#83595=CARTESIAN_POINT('',(516.,-3.57145386584454,-10.4310698053529));
#83596=CARTESIAN_POINT('Origin',(516.,-2.12256512641094,-10.8192983730066));
#83597=CARTESIAN_POINT('',(536.,-2.48478731126934,-10.7222412310932));
#83598=CARTESIAN_POINT('Origin',(535.7,0.,0.));
#83599=CARTESIAN_POINT('',(536.,-5.03813204405572,-10.2263006755453));
#83600=CARTESIAN_POINT('Origin',(536.,0.,0.));
#83601=CARTESIAN_POINT('Ctrl Pts',(536.,-5.03813204405572,-10.2263006755453));
#83602=CARTESIAN_POINT('Ctrl Pts',(535.707724072523,-5.18458729933076,-10.4799686187172));
#83603=CARTESIAN_POINT('Ctrl Pts',(535.4,-5.33875073066342,-10.7469875144545));
#83604=CARTESIAN_POINT('Origin',(516.,-5.60048094716168,-11.2003175473055));
#83605=CARTESIAN_POINT('',(536.,-4.85048094716168,-9.90127944162882));
#83606=CARTESIAN_POINT('',(536.,-2.47548094716167,-5.78765877365274));
#83607=CARTESIAN_POINT('',(516.,-4.85048094716168,-9.90127944162882));
#83608=CARTESIAN_POINT('',(516.,-4.85048094716168,-9.90127944162882));
#83609=CARTESIAN_POINT('',(516.,-5.60048094716168,-11.2003175473055));
#83610=CARTESIAN_POINT('Origin',(516.,-5.87500000000001,-10.1757984944672));
#83611=CARTESIAN_POINT('',(516.,-6.14951905283833,-9.15127944162882));
#83612=CARTESIAN_POINT('',(516.,-4.85048094716168,-9.90127944162882));
#83613=CARTESIAN_POINT('',(516.,-6.14951905283833,-9.15127944162882));
#83614=CARTESIAN_POINT('Origin',(516.,-6.14951905283833,-9.15127944162882));
#83615=CARTESIAN_POINT('',(536.,-6.33717014973238,-9.47630067554534));
#83616=CARTESIAN_POINT('',(536.,-6.14951905283833,-9.15127944162882));
#83617=CARTESIAN_POINT('',(536.,-3.39951905283833,-4.38813972081441));
#83618=CARTESIAN_POINT('Ctrl Pts',(535.4,-6.63778883634008,-9.99698751445449));
#83619=CARTESIAN_POINT('Ctrl Pts',(535.707724067986,-6.48362540728046,-9.7299686226542));
#83620=CARTESIAN_POINT('Ctrl Pts',(536.,-6.33717014973238,-9.47630067554533));
#83621=CARTESIAN_POINT('',(516.,-6.14951905283833,-9.15127944162882));
#83622=CARTESIAN_POINT('Origin',(516.,-4.85048094716168,-9.90127944162882));
#83623=CARTESIAN_POINT('',(536.,-5.17524047358084,-9.71377944162882));
#83624=CARTESIAN_POINT('Origin',(535.7,0.,0.));
#83625=CARTESIAN_POINT('',(536.,-7.51322323338386,-8.57388340516367));
#83626=CARTESIAN_POINT('Origin',(536.,0.,0.));
#83627=CARTESIAN_POINT('Ctrl Pts',(536.,-7.51322323338386,-8.57388340516367));
#83628=CARTESIAN_POINT('Ctrl Pts',(535.70772406487,-7.72034224709731,-8.78100241887712));
#83629=CARTESIAN_POINT('Ctrl Pts',(535.4,-7.93836225708725,-8.99902242886707));
#83630=CARTESIAN_POINT('Origin',(516.,-8.30850467894194,-9.36916485072175));
#83631=CARTESIAN_POINT('',(536.,-7.24784450716212,-8.30850467894193));
#83632=CARTESIAN_POINT('',(536.,-3.88908729652601,-4.94974746830583));
#83633=CARTESIAN_POINT('',(516.,-7.24784450716212,-8.30850467894193));
#83634=CARTESIAN_POINT('',(516.,-7.24784450716212,-8.30850467894193));
#83635=CARTESIAN_POINT('',(516.,-8.30850467894194,-9.36916485072175));
#83636=CARTESIAN_POINT('Origin',(516.,-8.30850467894194,-8.30850467894193));
#83637=CARTESIAN_POINT('',(516.,-8.30850467894194,-7.24784450716211));
#83638=CARTESIAN_POINT('',(516.,-7.24784450716212,-8.30850467894193));
#83639=CARTESIAN_POINT('',(516.,-8.30850467894194,-7.24784450716211));
#83640=CARTESIAN_POINT('Origin',(516.,-8.30850467894194,-7.24784450716211));
#83641=CARTESIAN_POINT('',(536.,-8.57388340516368,-7.51322323338385));
#83642=CARTESIAN_POINT('',(536.,-8.30850467894194,-7.24784450716211));
#83643=CARTESIAN_POINT('',(536.,-4.41941738241592,-3.3587572106361));
#83644=CARTESIAN_POINT('Ctrl Pts',(535.4,-8.99902242886708,-7.93836225708724));
#83645=CARTESIAN_POINT('Ctrl Pts',(535.707724071117,-8.78100241445101,-7.72034224267118));
#83646=CARTESIAN_POINT('Ctrl Pts',(536.,-8.57388340516368,-7.51322323338385));
#83647=CARTESIAN_POINT('',(516.,-8.30850467894194,-7.24784450716211));
#83648=CARTESIAN_POINT('Origin',(516.,-7.24784450716212,-8.30850467894193));
#83649=CARTESIAN_POINT('',(536.,-7.51300955010707,-8.04333963599697));
#83650=CARTESIAN_POINT('Origin',(535.7,0.,0.));
#83651=CARTESIAN_POINT('',(536.,-9.47630067554534,-6.33717014973237));
#83652=CARTESIAN_POINT('Origin',(536.,0.,0.));
#83653=CARTESIAN_POINT('Ctrl Pts',(536.,-9.47630067554534,-6.33717014973237));
#83654=CARTESIAN_POINT('Ctrl Pts',(535.707724077208,-9.72996861465175,-6.48362540266023));
#83655=CARTESIAN_POINT('Ctrl Pts',(535.4,-9.9969875144545,-6.63778883634007));
#83656=CARTESIAN_POINT('Origin',(516.,-10.4503175473055,-6.89951905283833));
#83657=CARTESIAN_POINT('',(536.,-9.15127944162883,-6.14951905283833));
#83658=CARTESIAN_POINT('',(536.,-5.03765877365274,-3.77451905283833));
#83659=CARTESIAN_POINT('',(516.,-9.15127944162883,-6.14951905283833));
#83660=CARTESIAN_POINT('',(516.,-9.15127944162883,-6.14951905283833));
#83661=CARTESIAN_POINT('',(516.,-10.4503175473055,-6.89951905283833));
#83662=CARTESIAN_POINT('Origin',(516.,-10.1757984944672,-5.875));
#83663=CARTESIAN_POINT('',(516.,-9.90127944162883,-4.85048094716167));
#83664=CARTESIAN_POINT('',(516.,-9.15127944162883,-6.14951905283833));
#83665=CARTESIAN_POINT('',(516.,-9.90127944162883,-4.85048094716167));
#83666=CARTESIAN_POINT('Origin',(516.,-9.90127944162883,-4.85048094716167));
#83667=CARTESIAN_POINT('',(536.,-10.2263006755453,-5.03813204405571));
#83668=CARTESIAN_POINT('',(536.,-9.90127944162883,-4.85048094716167));
#83669=CARTESIAN_POINT('',(536.,-5.13813972081441,-2.10048094716167));
#83670=CARTESIAN_POINT('Ctrl Pts',(535.4,-10.7469875144545,-5.33875073066341));
#83671=CARTESIAN_POINT('Ctrl Pts',(535.707724072359,-10.4799686188595,-5.18458729941291));
#83672=CARTESIAN_POINT('Ctrl Pts',(536.,-10.2263006755453,-5.03813204405571));
#83673=CARTESIAN_POINT('',(516.,-9.90127944162883,-4.85048094716167));
#83674=CARTESIAN_POINT('Origin',(516.,-9.15127944162883,-6.14951905283833));
#83675=CARTESIAN_POINT('',(536.,-9.33877944162883,-5.82475952641916));
#83676=CARTESIAN_POINT('Origin',(535.7,0.,0.));
#83677=CARTESIAN_POINT('',(536.,-10.7935838869957,-3.66858922126564));
#83678=CARTESIAN_POINT('Origin',(536.,0.,0.));
#83679=CARTESIAN_POINT('Ctrl Pts',(536.,-10.7935838869957,-3.66858922126564));
#83680=CARTESIAN_POINT('Ctrl Pts',(535.707724073214,-11.0765137132584,-3.74440003972739));
#83681=CARTESIAN_POINT('Ctrl Pts',(535.4,-11.3743345935147,-3.82420090408119));
#83682=CARTESIAN_POINT('Origin',(516.,-11.8799585447865,-3.95968243349831));
#83683=CARTESIAN_POINT('',(536.,-10.4310698053529,-3.57145386584453));
#83684=CARTESIAN_POINT('',(536.,-5.84292213047979,-2.34206340160755));
#83685=CARTESIAN_POINT('',(516.,-10.4310698053529,-3.57145386584453));
#83686=CARTESIAN_POINT('',(516.,-10.4310698053529,-3.57145386584453));
#83687=CARTESIAN_POINT('',(516.,-11.8799585447865,-3.95968243349831));
#83688=CARTESIAN_POINT('Origin',(516.,-11.3496284588966,-3.04112377995461));
#83689=CARTESIAN_POINT('',(516.,-10.8192983730066,-2.12256512641092));
#83690=CARTESIAN_POINT('',(516.,-10.4310698053529,-3.57145386584453));
#83691=CARTESIAN_POINT('',(516.,-10.8192983730066,-2.12256512641092));
#83692=CARTESIAN_POINT('Origin',(516.,-10.8192983730066,-2.12256512641092));
#83693=CARTESIAN_POINT('',(536.,-11.1818124546495,-2.21970048183204));
#83694=CARTESIAN_POINT('',(536.,-10.8192983730066,-2.12256512641092));
#83695=CARTESIAN_POINT('',(536.,-5.50670632841677,-0.699060378347061));
#83696=CARTESIAN_POINT('Ctrl Pts',(535.4,-11.7625631611685,-2.37531216464759));
#83697=CARTESIAN_POINT('Ctrl Pts',(535.707724065083,-11.4647422887831,-2.29551130240282));
#83698=CARTESIAN_POINT('Ctrl Pts',(536.,-11.1818124546495,-2.21970048183204));
#83699=CARTESIAN_POINT('',(516.,-10.8192983730066,-2.12256512641092));
#83700=CARTESIAN_POINT('Origin',(516.,-10.4310698053529,-3.57145386584453));
#83701=CARTESIAN_POINT('',(536.,-10.5281269472663,-3.20923168098613));
#83702=CARTESIAN_POINT('Origin',(535.7,0.,0.));
#83703=CARTESIAN_POINT('',(536.,-11.3753021937881,-0.749999999999999));
#83704=CARTESIAN_POINT('Origin',(536.,0.,0.));
#83705=CARTESIAN_POINT('Ctrl Pts',(536.,-11.3753021937881,-0.749999999999999));
#83706=CARTESIAN_POINT('Ctrl Pts',(535.707724067994,-11.668212708876,-0.749999999999999));
#83707=CARTESIAN_POINT('Ctrl Pts',(535.4,-11.9765395670035,-0.749999999999999));
#83708=CARTESIAN_POINT('Origin',(516.,-12.5,-0.749999999999998));
#83709=CARTESIAN_POINT('',(536.,-11.,-0.749999999999999));
#83710=CARTESIAN_POINT('',(536.,-6.25,-0.749999999999999));
#83711=CARTESIAN_POINT('',(516.,-11.,-0.749999999999999));
#83712=CARTESIAN_POINT('',(516.,-11.,-0.749999999999999));
#83713=CARTESIAN_POINT('',(516.,-12.5,-0.749999999999998));
#83714=CARTESIAN_POINT('Origin',(516.,-11.75,1.43895998899814E-15));
#83715=CARTESIAN_POINT('',(516.,-11.,0.750000000000001));
#83716=CARTESIAN_POINT('',(516.,-11.,-0.749999999999999));
#83717=CARTESIAN_POINT('',(516.,-11.,0.750000000000001));
#83718=CARTESIAN_POINT('Origin',(516.,-11.,0.750000000000001));
#83719=CARTESIAN_POINT('',(536.,-11.3753021937881,0.750000000000001));
#83720=CARTESIAN_POINT('',(536.,-11.,0.750000000000001));
#83721=CARTESIAN_POINT('',(536.,-5.5,0.750000000000001));
#83722=CARTESIAN_POINT('Ctrl Pts',(535.4,-11.9765395670035,0.750000000000001));
#83723=CARTESIAN_POINT('Ctrl Pts',(535.707724067994,-11.668212708876,0.750000000000002));
#83724=CARTESIAN_POINT('Ctrl Pts',(536.,-11.3753021937881,0.750000000000002));
#83725=CARTESIAN_POINT('',(516.,-11.,0.750000000000001));
#83726=CARTESIAN_POINT('Origin',(516.,-11.,-0.749999999999999));
#83727=CARTESIAN_POINT('',(536.,-11.,-0.374999999999999));
#83728=CARTESIAN_POINT('Origin',(535.7,0.,0.));
#83729=CARTESIAN_POINT('',(536.,-11.1818124546495,2.21970048183204));
#83730=CARTESIAN_POINT('Origin',(536.,0.,0.));
#83731=CARTESIAN_POINT('Ctrl Pts',(536.,-11.1818124546495,2.21970048183204));
#83732=CARTESIAN_POINT('Ctrl Pts',(535.707724065255,-11.4647422886159,2.29551130235802));
#83733=CARTESIAN_POINT('Ctrl Pts',(535.4,-11.7625631611684,2.3753121646476));
#83734=CARTESIAN_POINT('Origin',(516.,-12.2681871124402,2.51079369406471));
#83735=CARTESIAN_POINT('',(536.,-10.8192983730066,2.12256512641093));
#83736=CARTESIAN_POINT('',(536.,-6.23115069813357,0.893174662173955));
#83737=CARTESIAN_POINT('',(516.,-10.8192983730066,2.12256512641093));
#83738=CARTESIAN_POINT('',(516.,-10.8192983730066,2.12256512641093));
#83739=CARTESIAN_POINT('',(516.,-12.2681871124402,2.51079369406471));
#83740=CARTESIAN_POINT('Origin',(516.,-11.3496284588966,3.04112377995462));
#83741=CARTESIAN_POINT('',(516.,-10.4310698053529,3.57145386584453));
#83742=CARTESIAN_POINT('',(516.,-10.8192983730066,2.12256512641093));
#83743=CARTESIAN_POINT('',(516.,-10.4310698053529,3.57145386584453));
#83744=CARTESIAN_POINT('Origin',(516.,-10.4310698053529,3.57145386584453));
#83745=CARTESIAN_POINT('',(536.,-10.7935838869957,3.66858922126565));
#83746=CARTESIAN_POINT('',(536.,-10.4310698053529,3.57145386584453));
#83747=CARTESIAN_POINT('',(536.,-5.11847776076298,2.14794911778067));
#83748=CARTESIAN_POINT('Ctrl Pts',(535.4,-11.3743345935147,3.8242009040812));
#83749=CARTESIAN_POINT('Ctrl Pts',(535.707724073633,-11.076513712853,3.74440003961878));
#83750=CARTESIAN_POINT('Ctrl Pts',(536.,-10.7935838869957,3.66858922126565));
#83751=CARTESIAN_POINT('',(516.,-10.4310698053529,3.57145386584453));
#83752=CARTESIAN_POINT('Origin',(516.,-10.8192983730066,2.12256512641093));
#83753=CARTESIAN_POINT('',(536.,-10.7222412310932,2.48478731126933));
#83754=CARTESIAN_POINT('Origin',(535.7,0.,0.));
#83755=CARTESIAN_POINT('',(536.,-10.2263006755453,5.03813204405572));
#83756=CARTESIAN_POINT('Origin',(536.,0.,0.));
#83757=CARTESIAN_POINT('Ctrl Pts',(536.,-10.2263006755453,5.03813204405572));
#83758=CARTESIAN_POINT('Ctrl Pts',(535.707724067529,-10.4799686230507,5.18458730183271));
#83759=CARTESIAN_POINT('Ctrl Pts',(535.4,-10.7469875144545,5.33875073066342));
#83760=CARTESIAN_POINT('Origin',(516.,-11.2003175473055,5.60048094716168));
#83761=CARTESIAN_POINT('',(536.,-9.90127944162882,4.85048094716167));
#83762=CARTESIAN_POINT('',(536.,-5.78765877365274,2.47548094716167));
#83763=CARTESIAN_POINT('',(516.,-9.90127944162882,4.85048094716167));
#83764=CARTESIAN_POINT('',(516.,-9.90127944162882,4.85048094716167));
#83765=CARTESIAN_POINT('',(516.,-11.2003175473055,5.60048094716168));
#83766=CARTESIAN_POINT('Origin',(516.,-10.1757984944672,5.875));
#83767=CARTESIAN_POINT('',(516.,-9.15127944162882,6.14951905283833));
#83768=CARTESIAN_POINT('',(516.,-9.90127944162882,4.85048094716167));
#83769=CARTESIAN_POINT('',(516.,-9.15127944162882,6.14951905283833));
#83770=CARTESIAN_POINT('Origin',(516.,-9.15127944162882,6.14951905283833));
#83771=CARTESIAN_POINT('',(536.,-9.47630067554534,6.33717014973237));
#83772=CARTESIAN_POINT('',(536.,-9.15127944162882,6.14951905283833));
#83773=CARTESIAN_POINT('',(536.,-4.38813972081441,3.39951905283833));
#83774=CARTESIAN_POINT('Ctrl Pts',(535.4,-9.9969875144545,6.63778883634007));
#83775=CARTESIAN_POINT('Ctrl Pts',(535.707724067522,-9.72996862305692,6.48362540751297));
#83776=CARTESIAN_POINT('Ctrl Pts',(536.,-9.47630067554533,6.33717014973238));
#83777=CARTESIAN_POINT('',(516.,-9.15127944162882,6.14951905283833));
#83778=CARTESIAN_POINT('Origin',(516.,-9.90127944162882,4.85048094716167));
#83779=CARTESIAN_POINT('',(536.,-9.71377944162882,5.17524047358084));
#83780=CARTESIAN_POINT('Origin',(535.7,0.,0.));
#83781=CARTESIAN_POINT('',(536.,-8.57388340516368,7.51322323338386));
#83782=CARTESIAN_POINT('Origin',(536.,0.,0.));
#83783=CARTESIAN_POINT('Ctrl Pts',(536.,-8.57388340516368,7.51322323338386));
#83784=CARTESIAN_POINT('Ctrl Pts',(535.707724067841,-8.78100241677203,7.72034224499221));
#83785=CARTESIAN_POINT('Ctrl Pts',(535.4,-8.99902242886707,7.93836225708725));
#83786=CARTESIAN_POINT('Origin',(516.,-9.36916485072175,8.30850467894193));
#83787=CARTESIAN_POINT('',(536.,-8.30850467894193,7.24784450716211));
#83788=CARTESIAN_POINT('',(536.,-4.94974746830583,3.88908729652601));
#83789=CARTESIAN_POINT('',(516.,-8.30850467894193,7.24784450716211));
#83790=CARTESIAN_POINT('',(516.,-8.30850467894193,7.24784450716211));
#83791=CARTESIAN_POINT('',(516.,-9.36916485072175,8.30850467894193));
#83792=CARTESIAN_POINT('Origin',(516.,-8.30850467894193,8.30850467894193));
#83793=CARTESIAN_POINT('',(516.,-7.24784450716211,8.30850467894193));
#83794=CARTESIAN_POINT('',(516.,-8.30850467894193,7.24784450716211));
#83795=CARTESIAN_POINT('',(516.,-7.24784450716211,8.30850467894193));
#83796=CARTESIAN_POINT('Origin',(516.,-7.24784450716211,8.30850467894193));
#83797=CARTESIAN_POINT('',(536.,-7.51322323338385,8.57388340516368));
#83798=CARTESIAN_POINT('',(536.,-7.24784450716211,8.30850467894193));
#83799=CARTESIAN_POINT('',(536.,-3.3587572106361,4.41941738241592));
#83800=CARTESIAN_POINT('Ctrl Pts',(535.4,-7.93836225708725,8.99902242886707));
#83801=CARTESIAN_POINT('Ctrl Pts',(535.707724067841,-7.72034224499221,8.78100241677203));
#83802=CARTESIAN_POINT('Ctrl Pts',(536.,-7.51322323338385,8.57388340516368));
#83803=CARTESIAN_POINT('',(516.,-7.24784450716211,8.30850467894193));
#83804=CARTESIAN_POINT('Origin',(516.,-8.30850467894193,7.24784450716211));
#83805=CARTESIAN_POINT('',(536.,-8.04333963599698,7.51300955010707));
#83806=CARTESIAN_POINT('Origin',(535.7,0.,0.));
#83807=CARTESIAN_POINT('',(536.,-6.33717014973237,9.47630067554534));
#83808=CARTESIAN_POINT('Origin',(536.,0.,0.));
#83809=CARTESIAN_POINT('Ctrl Pts',(536.,-6.33717014973237,9.47630067554534));
#83810=CARTESIAN_POINT('Ctrl Pts',(535.707724067684,-6.48362540743208,9.72996862291682));
#83811=CARTESIAN_POINT('Ctrl Pts',(535.4,-6.63778883634007,9.9969875144545));
#83812=CARTESIAN_POINT('Origin',(516.,-6.89951905283833,10.4503175473055));
#83813=CARTESIAN_POINT('',(536.,-6.14951905283833,9.15127944162883));
#83814=CARTESIAN_POINT('',(536.,-3.77451905283833,5.03765877365274));
#83815=CARTESIAN_POINT('',(516.,-6.14951905283833,9.15127944162883));
#83816=CARTESIAN_POINT('',(516.,-6.14951905283833,9.15127944162883));
#83817=CARTESIAN_POINT('',(516.,-6.89951905283833,10.4503175473055));
#83818=CARTESIAN_POINT('Origin',(516.,-5.875,10.1757984944672));
#83819=CARTESIAN_POINT('',(516.,-4.85048094716167,9.90127944162883));
#83820=CARTESIAN_POINT('',(516.,-6.14951905283833,9.15127944162883));
#83821=CARTESIAN_POINT('',(516.,-4.85048094716167,9.90127944162883));
#83822=CARTESIAN_POINT('Origin',(516.,-4.85048094716167,9.90127944162883));
#83823=CARTESIAN_POINT('',(536.,-5.03813204405571,10.2263006755453));
#83824=CARTESIAN_POINT('',(536.,-4.85048094716167,9.90127944162883));
#83825=CARTESIAN_POINT('',(536.,-2.10048094716167,5.13813972081441));
#83826=CARTESIAN_POINT('Ctrl Pts',(535.4,-5.33875073066341,10.7469875144545));
#83827=CARTESIAN_POINT('Ctrl Pts',(535.707724067682,-5.18458730175635,10.4799686229184));
#83828=CARTESIAN_POINT('Ctrl Pts',(536.,-5.03813204405571,10.2263006755453));
#83829=CARTESIAN_POINT('',(516.,-4.85048094716167,9.90127944162883));
#83830=CARTESIAN_POINT('Origin',(516.,-6.14951905283833,9.15127944162883));
#83831=CARTESIAN_POINT('',(536.,-5.82475952641916,9.33877944162883));
#83832=CARTESIAN_POINT('Origin',(535.7,0.,0.));
#83833=CARTESIAN_POINT('',(536.,-3.66858922126564,10.7935838869957));
#83834=CARTESIAN_POINT('Origin',(536.,0.,0.));
#83835=CARTESIAN_POINT('Ctrl Pts',(536.,-3.66858922126564,10.7935838869957));
#83836=CARTESIAN_POINT('Ctrl Pts',(535.707724060762,-3.74440004295685,11.0765137253109));
#83837=CARTESIAN_POINT('Ctrl Pts',(535.4,-3.8242009040812,11.3743345935147));
#83838=CARTESIAN_POINT('Origin',(516.,-3.95968243349831,11.8799585447865));
#83839=CARTESIAN_POINT('',(536.,-3.57145386584453,10.4310698053529));
#83840=CARTESIAN_POINT('',(536.,-2.34206340160756,5.84292213047979));
#83841=CARTESIAN_POINT('',(516.,-3.57145386584453,10.4310698053529));
#83842=CARTESIAN_POINT('',(516.,-3.57145386584453,10.4310698053529));
#83843=CARTESIAN_POINT('',(516.,-3.95968243349831,11.8799585447865));
#83844=CARTESIAN_POINT('Origin',(516.,-3.04112377995462,11.3496284588966));
#83845=CARTESIAN_POINT('',(516.,-2.12256512641093,10.8192983730066));
#83846=CARTESIAN_POINT('',(516.,-3.57145386584453,10.4310698053529));
#83847=CARTESIAN_POINT('',(516.,-2.12256512641093,10.8192983730066));
#83848=CARTESIAN_POINT('Origin',(516.,-2.12256512641093,10.8192983730066));
#83849=CARTESIAN_POINT('',(536.,-2.21970048183204,11.1818124546495));
#83850=CARTESIAN_POINT('',(536.,-2.12256512641093,10.8192983730066));
#83851=CARTESIAN_POINT('',(536.,-0.699060378347062,5.50670632841677));
#83852=CARTESIAN_POINT('Ctrl Pts',(535.4,-2.3753121646476,11.7625631611684));
#83853=CARTESIAN_POINT('Ctrl Pts',(535.707724068998,-2.29551130138738,11.4647422849935));
#83854=CARTESIAN_POINT('Ctrl Pts',(536.,-2.21970048183204,11.1818124546495));
#83855=CARTESIAN_POINT('',(516.,-2.12256512641093,10.8192983730066));
#83856=CARTESIAN_POINT('Origin',(516.,-3.57145386584453,10.4310698053529));
#83857=CARTESIAN_POINT('',(536.,-3.20923168098613,10.5281269472663));
#83858=CARTESIAN_POINT('Origin',(535.7,0.,0.));
#83859=CARTESIAN_POINT('',(536.,-0.749999999999999,11.3753021937881));
#83860=CARTESIAN_POINT('Origin',(536.,0.,0.));
#83861=CARTESIAN_POINT('Ctrl Pts',(536.,-0.749999999999999,11.3753021937881));
#83862=CARTESIAN_POINT('Ctrl Pts',(535.707724072196,-0.749999999999999,
11.6682127046657));
#83863=CARTESIAN_POINT('Ctrl Pts',(535.4,-0.749999999999999,11.9765395670035));
#83864=CARTESIAN_POINT('Origin',(516.,-0.749999999999999,12.5));
#83865=CARTESIAN_POINT('',(536.,-0.749999999999999,11.));
#83866=CARTESIAN_POINT('',(536.,-0.75,6.25));
#83867=CARTESIAN_POINT('',(516.,-0.749999999999999,11.));
#83868=CARTESIAN_POINT('',(516.,-0.749999999999999,11.));
#83869=CARTESIAN_POINT('',(516.,-0.749999999999999,12.5));
#83870=CARTESIAN_POINT('Origin',(516.,7.1947999449907E-16,11.75));
#83871=CARTESIAN_POINT('',(516.,0.750000000000001,11.));
#83872=CARTESIAN_POINT('',(516.,-0.749999999999999,11.));
#83873=CARTESIAN_POINT('',(516.,0.750000000000001,11.));
#83874=CARTESIAN_POINT('Origin',(516.,0.750000000000001,11.));
#83875=CARTESIAN_POINT('',(536.,0.750000000000001,11.3753021937881));
#83876=CARTESIAN_POINT('',(536.,0.750000000000001,11.));
#83877=CARTESIAN_POINT('',(536.,0.75,5.5));
#83878=CARTESIAN_POINT('Ctrl Pts',(535.4,0.750000000000001,11.9765395670035));
#83879=CARTESIAN_POINT('Ctrl Pts',(535.707724072196,0.750000000000001,11.6682127046657));
#83880=CARTESIAN_POINT('Ctrl Pts',(536.,0.750000000000001,11.3753021937881));
#83881=CARTESIAN_POINT('',(516.,0.750000000000001,11.));
#83882=CARTESIAN_POINT('Origin',(516.,-0.749999999999999,11.));
#83883=CARTESIAN_POINT('',(536.,-0.374999999999999,11.));
#83884=CARTESIAN_POINT('Origin',(535.7,0.,0.));
#83885=CARTESIAN_POINT('',(536.,2.21970048183204,11.1818124546495));
#83886=CARTESIAN_POINT('Origin',(536.,0.,0.));
#83887=CARTESIAN_POINT('Ctrl Pts',(536.,2.21970048183204,11.1818124546495));
#83888=CARTESIAN_POINT('Ctrl Pts',(535.707724065103,2.29551130239759,11.4647422887636));
#83889=CARTESIAN_POINT('Ctrl Pts',(535.4,2.3753121646476,11.7625631611684));
#83890=CARTESIAN_POINT('Origin',(516.,2.51079369406471,12.2681871124402));
#83891=CARTESIAN_POINT('',(536.,2.12256512641093,10.8192983730066));
#83892=CARTESIAN_POINT('',(536.,0.893174662173955,6.23115069813357));
#83893=CARTESIAN_POINT('',(516.,2.12256512641093,10.8192983730066));
#83894=CARTESIAN_POINT('',(516.,2.12256512641093,10.8192983730066));
#83895=CARTESIAN_POINT('',(516.,2.51079369406471,12.2681871124402));
#83896=CARTESIAN_POINT('Origin',(516.,3.04112377995462,11.3496284588966));
#83897=CARTESIAN_POINT('',(516.,3.57145386584453,10.4310698053529));
#83898=CARTESIAN_POINT('',(516.,2.12256512641093,10.8192983730066));
#83899=CARTESIAN_POINT('',(516.,3.57145386584453,10.4310698053529));
#83900=CARTESIAN_POINT('Origin',(516.,3.57145386584453,10.4310698053529));
#83901=CARTESIAN_POINT('',(536.,3.66858922126565,10.7935838869957));
#83902=CARTESIAN_POINT('',(536.,3.57145386584453,10.4310698053529));
#83903=CARTESIAN_POINT('',(536.,2.14794911778067,5.11847776076298));
#83904=CARTESIAN_POINT('Ctrl Pts',(535.4,3.8242009040812,11.3743345935147));
#83905=CARTESIAN_POINT('Ctrl Pts',(535.707724065364,3.74440004176344,11.076513720857));
#83906=CARTESIAN_POINT('Ctrl Pts',(536.,3.66858922126565,10.7935838869957));
#83907=CARTESIAN_POINT('',(516.,3.57145386584453,10.4310698053529));
#83908=CARTESIAN_POINT('Origin',(516.,2.12256512641093,10.8192983730066));
#83909=CARTESIAN_POINT('',(536.,2.48478731126933,10.7222412310932));
#83910=CARTESIAN_POINT('Origin',(535.7,0.,0.));
#83911=CARTESIAN_POINT('',(536.,5.03813204405571,10.2263006755453));
#83912=CARTESIAN_POINT('Origin',(536.,0.,0.));
#83913=CARTESIAN_POINT('Ctrl Pts',(536.,5.03813204405571,10.2263006755453));
#83914=CARTESIAN_POINT('Ctrl Pts',(535.707724067691,5.18458730175182,10.4799686229106));
#83915=CARTESIAN_POINT('Ctrl Pts',(535.4,5.33875073066341,10.7469875144545));
#83916=CARTESIAN_POINT('Origin',(516.,5.60048094716167,11.2003175473055));
#83917=CARTESIAN_POINT('',(536.,4.85048094716167,9.90127944162882));
#83918=CARTESIAN_POINT('',(536.,2.47548094716167,5.78765877365274));
#83919=CARTESIAN_POINT('',(516.,4.85048094716167,9.90127944162882));
#83920=CARTESIAN_POINT('',(516.,4.85048094716167,9.90127944162882));
#83921=CARTESIAN_POINT('',(516.,5.60048094716167,11.2003175473055));
#83922=CARTESIAN_POINT('Origin',(516.,5.875,10.1757984944672));
#83923=CARTESIAN_POINT('',(516.,6.14951905283833,9.15127944162883));
#83924=CARTESIAN_POINT('',(516.,4.85048094716167,9.90127944162882));
#83925=CARTESIAN_POINT('',(516.,6.14951905283833,9.15127944162883));
#83926=CARTESIAN_POINT('Origin',(516.,6.14951905283833,9.15127944162883));
#83927=CARTESIAN_POINT('',(536.,6.33717014973237,9.47630067554534));
#83928=CARTESIAN_POINT('',(536.,6.14951905283833,9.15127944162883));
#83929=CARTESIAN_POINT('',(536.,3.39951905283833,4.38813972081441));
#83930=CARTESIAN_POINT('Ctrl Pts',(535.4,6.63778883634007,9.9969875144545));
#83931=CARTESIAN_POINT('Ctrl Pts',(535.707724072531,6.48362540500314,9.72996861870978));
#83932=CARTESIAN_POINT('Ctrl Pts',(536.,6.33717014973237,9.47630067554534));
#83933=CARTESIAN_POINT('',(516.,6.14951905283833,9.15127944162883));
#83934=CARTESIAN_POINT('Origin',(516.,4.85048094716167,9.90127944162882));
#83935=CARTESIAN_POINT('',(536.,5.17524047358084,9.71377944162882));
#83936=CARTESIAN_POINT('Origin',(535.7,0.,0.));
#83937=CARTESIAN_POINT('',(536.,7.51322323338386,8.57388340516368));
#83938=CARTESIAN_POINT('Origin',(536.,0.,0.));
#83939=CARTESIAN_POINT('Ctrl Pts',(536.,7.51322323338386,8.57388340516368));
#83940=CARTESIAN_POINT('Ctrl Pts',(535.707724070812,7.72034224288731,8.78100241466713));
#83941=CARTESIAN_POINT('Ctrl Pts',(535.4,7.93836225708725,8.99902242886707));
#83942=CARTESIAN_POINT('Origin',(516.,8.30850467894193,9.36916485072176));
#83943=CARTESIAN_POINT('',(536.,7.24784450716211,8.30850467894193));
#83944=CARTESIAN_POINT('',(536.,3.88908729652601,4.94974746830583));
#83945=CARTESIAN_POINT('',(516.,7.24784450716211,8.30850467894193));
#83946=CARTESIAN_POINT('',(516.,7.24784450716211,8.30850467894193));
#83947=CARTESIAN_POINT('',(516.,8.30850467894193,9.36916485072176));
#83948=CARTESIAN_POINT('Origin',(516.,8.30850467894193,8.30850467894193));
#83949=CARTESIAN_POINT('',(516.,8.30850467894193,7.24784450716211));
#83950=CARTESIAN_POINT('',(516.,7.24784450716211,8.30850467894193));
#83951=CARTESIAN_POINT('',(516.,8.30850467894193,7.24784450716211));
#83952=CARTESIAN_POINT('Origin',(516.,8.30850467894193,7.24784450716211));
#83953=CARTESIAN_POINT('',(536.,8.57388340516368,7.51322323338386));
#83954=CARTESIAN_POINT('',(536.,8.30850467894193,7.24784450716211));
#83955=CARTESIAN_POINT('',(536.,4.41941738241592,3.3587572106361));
#83956=CARTESIAN_POINT('Ctrl Pts',(535.4,8.99902242886707,7.93836225708725));
#83957=CARTESIAN_POINT('Ctrl Pts',(535.707724070812,8.78100241466713,7.72034224288731));
#83958=CARTESIAN_POINT('Ctrl Pts',(536.,8.57388340516368,7.51322323338386));
#83959=CARTESIAN_POINT('',(516.,8.30850467894193,7.24784450716211));
#83960=CARTESIAN_POINT('Origin',(516.,7.24784450716211,8.30850467894193));
#83961=CARTESIAN_POINT('',(536.,7.51300955010707,8.04333963599698));
#83962=CARTESIAN_POINT('Origin',(535.7,0.,0.));
#83963=CARTESIAN_POINT('',(536.,9.47630067554534,6.33717014973237));
#83964=CARTESIAN_POINT('Origin',(536.,0.,0.));
#83965=CARTESIAN_POINT('Ctrl Pts',(536.,9.47630067554534,6.33717014973237));
#83966=CARTESIAN_POINT('Ctrl Pts',(535.707724067527,9.72996862305299,6.48362540751069));
#83967=CARTESIAN_POINT('Ctrl Pts',(535.4,9.9969875144545,6.63778883634007));
#83968=CARTESIAN_POINT('Origin',(516.,10.4503175473055,6.89951905283833));
#83969=CARTESIAN_POINT('',(536.,9.15127944162883,6.14951905283833));
#83970=CARTESIAN_POINT('',(536.,5.03765877365274,3.77451905283833));
#83971=CARTESIAN_POINT('',(516.,9.15127944162883,6.14951905283833));
#83972=CARTESIAN_POINT('',(516.,9.15127944162883,6.14951905283833));
#83973=CARTESIAN_POINT('',(516.,10.4503175473055,6.89951905283833));
#83974=CARTESIAN_POINT('Origin',(516.,10.1757984944672,5.875));
#83975=CARTESIAN_POINT('',(516.,9.90127944162883,4.85048094716167));
#83976=CARTESIAN_POINT('',(516.,9.15127944162883,6.14951905283833));
#83977=CARTESIAN_POINT('',(516.,9.90127944162883,4.85048094716167));
#83978=CARTESIAN_POINT('Origin',(516.,9.90127944162883,4.85048094716167));
#83979=CARTESIAN_POINT('',(536.,10.2263006755453,5.03813204405571));
#83980=CARTESIAN_POINT('',(536.,9.90127944162883,4.85048094716167));
#83981=CARTESIAN_POINT('',(536.,5.13813972081441,2.10048094716167));
#83982=CARTESIAN_POINT('Ctrl Pts',(535.4,10.7469875144545,5.33875073066341));
#83983=CARTESIAN_POINT('Ctrl Pts',(535.707724067527,10.479968623053,5.18458730183403));
#83984=CARTESIAN_POINT('Ctrl Pts',(536.,10.2263006755453,5.03813204405571));
#83985=CARTESIAN_POINT('',(516.,9.90127944162883,4.85048094716167));
#83986=CARTESIAN_POINT('Origin',(516.,9.15127944162883,6.14951905283833));
#83987=CARTESIAN_POINT('',(536.,9.33877944162883,5.82475952641916));
#83988=CARTESIAN_POINT('Origin',(535.7,0.,0.));
#83989=CARTESIAN_POINT('',(536.,10.7935838869957,3.66858922126564));
#83990=CARTESIAN_POINT('Origin',(536.,0.,0.));
#83991=CARTESIAN_POINT('Ctrl Pts',(536.,10.7935838869957,3.66858922126564));
#83992=CARTESIAN_POINT('Ctrl Pts',(535.707724069742,11.0765137166189,3.74440004062786));
#83993=CARTESIAN_POINT('Ctrl Pts',(535.4,11.3743345935147,3.8242009040812));
#83994=CARTESIAN_POINT('Origin',(516.,11.8799585447865,3.95968243349831));
#83995=CARTESIAN_POINT('',(536.,10.4310698053529,3.57145386584453));
#83996=CARTESIAN_POINT('',(536.,5.84292213047979,2.34206340160756));
#83997=CARTESIAN_POINT('',(516.,10.4310698053529,3.57145386584453));
#83998=CARTESIAN_POINT('',(516.,10.4310698053529,3.57145386584453));
#83999=CARTESIAN_POINT('',(516.,11.8799585447865,3.95968243349831));
#84000=CARTESIAN_POINT('Origin',(516.,11.3496284588966,3.04112377995462));
#84001=CARTESIAN_POINT('',(516.,10.8192983730066,2.12256512641093));
#84002=CARTESIAN_POINT('',(516.,10.4310698053529,3.57145386584453));
#84003=CARTESIAN_POINT('',(516.,10.8192983730066,2.12256512641093));
#84004=CARTESIAN_POINT('Origin',(516.,10.8192983730066,2.12256512641093));
#84005=CARTESIAN_POINT('',(536.,11.1818124546495,2.21970048183204));
#84006=CARTESIAN_POINT('',(536.,10.8192983730066,2.12256512641093));
#84007=CARTESIAN_POINT('',(536.,5.50670632841677,0.699060378347062));
#84008=CARTESIAN_POINT('Ctrl Pts',(535.4,11.7625631611684,2.3753121646476));
#84009=CARTESIAN_POINT('Ctrl Pts',(535.70772407393,11.464742280219,2.29551130010806));
#84010=CARTESIAN_POINT('Ctrl Pts',(536.,11.1818124546495,2.21970048183204));
#84011=CARTESIAN_POINT('',(516.,10.8192983730066,2.12256512641093));
#84012=CARTESIAN_POINT('Origin',(516.,10.4310698053529,3.57145386584453));
#84013=CARTESIAN_POINT('',(536.,10.5281269472663,3.20923168098613));
#84014=CARTESIAN_POINT('Origin',(535.7,0.,0.));
#84015=CARTESIAN_POINT('',(536.,11.3753021937881,0.75));
#84016=CARTESIAN_POINT('Origin',(536.,0.,0.));
#84017=CARTESIAN_POINT('Ctrl Pts',(536.,11.3753021937881,0.75));
#84018=CARTESIAN_POINT('Ctrl Pts',(535.707724067994,11.668212708876,0.75));
#84019=CARTESIAN_POINT('Ctrl Pts',(535.4,11.9765395670035,0.75));
#84020=CARTESIAN_POINT('Origin',(516.,12.5,0.75));
#84021=CARTESIAN_POINT('',(536.,11.,0.75));
#84022=CARTESIAN_POINT('',(536.,6.25,0.75));
#84023=CARTESIAN_POINT('',(516.,11.,0.75));
#84024=CARTESIAN_POINT('',(516.,11.,0.75));
#84025=CARTESIAN_POINT('',(516.,12.5,0.75));
#84026=CARTESIAN_POINT('Origin',(516.,11.75,0.));
#84027=CARTESIAN_POINT('',(516.,11.,-0.75));
#84028=CARTESIAN_POINT('',(516.,11.,0.75));
#84029=CARTESIAN_POINT('',(516.,11.,-0.75));
#84030=CARTESIAN_POINT('Origin',(516.,11.,-0.75));
#84031=CARTESIAN_POINT('',(536.,11.,-0.75));
#84032=CARTESIAN_POINT('',(536.,5.5,-0.75));
#84033=CARTESIAN_POINT('',(516.,11.,-0.75));
#84034=CARTESIAN_POINT('Origin',(516.,11.,0.75));
#84035=CARTESIAN_POINT('',(536.,11.,0.375));
#84036=CARTESIAN_POINT('Origin',(139.,12.2681871124402,-2.51079369406472));
#84037=CARTESIAN_POINT('',(160.,10.8192983730066,-2.12256512641094));
#84038=CARTESIAN_POINT('',(160.,12.2681871124402,-2.51079369406472));
#84039=CARTESIAN_POINT('',(140.,10.8192983730066,-2.12256512641094));
#84040=CARTESIAN_POINT('',(139.,10.8192983730066,-2.12256512641094));
#84041=CARTESIAN_POINT('',(140.,11.1818124546495,-2.21970048183205));
#84042=CARTESIAN_POINT('',(140.,11.5493230989192,-2.31817466217396));
#84043=CARTESIAN_POINT('Ctrl Pts',(140.6,11.7625631611684,-2.3753121646476));
#84044=CARTESIAN_POINT('Ctrl Pts',(140.292275931137,11.4647422851234,-2.29551130142221));
#84045=CARTESIAN_POINT('Ctrl Pts',(140.,11.1818124546495,-2.21970048183204));
#84046=CARTESIAN_POINT('Origin',(139.,10.8192983730066,-2.12256512641094));
#84047=CARTESIAN_POINT('',(140.,10.4310698053529,-3.57145386584454));
#84048=CARTESIAN_POINT('',(140.,11.1040688303075,-1.05978731126933));
#84049=CARTESIAN_POINT('',(160.,10.4310698053529,-3.57145386584454));
#84050=CARTESIAN_POINT('',(160.,10.8192983730066,-2.12256512641094));
#84051=CARTESIAN_POINT('',(139.,10.4310698053529,-3.57145386584454));
#84052=CARTESIAN_POINT('Origin',(139.,10.4310698053529,-3.57145386584454));
#84053=CARTESIAN_POINT('',(140.,10.7935838869957,-3.66858922126565));
#84054=CARTESIAN_POINT('Ctrl Pts',(140.,10.7935838869957,-3.66858922126565));
#84055=CARTESIAN_POINT('Ctrl Pts',(140.292275926639,11.076513713116,-3.74440003968926));
#84056=CARTESIAN_POINT('Ctrl Pts',(140.6,11.3743345935146,-3.82420090408121));
#84057=CARTESIAN_POINT('',(140.,10.4366501615486,-3.57294911778067));
#84058=CARTESIAN_POINT('',(160.,10.4310698053529,-3.57145386584454));
#84059=CARTESIAN_POINT('Origin',(160.,11.3496284588966,-3.04112377995463));
#84060=CARTESIAN_POINT('Origin',(140.,11.4,0.));
#84061=CARTESIAN_POINT('',(140.,10.2263006755453,-5.03813204405572));
#84062=CARTESIAN_POINT('Origin',(140.,0.,0.));
#84063=CARTESIAN_POINT('',(140.,9.90127944162882,-4.85048094716168));
#84064=CARTESIAN_POINT('',(140.,10.0626587736527,-4.94365334794733));
#84065=CARTESIAN_POINT('',(140.,9.15127944162882,-6.14951905283833));
#84066=CARTESIAN_POINT('',(140.,11.1387794416288,-2.70706807279519));
#84067=CARTESIAN_POINT('',(140.,9.47630067554534,-6.33717014973238));
#84068=CARTESIAN_POINT('',(140.,8.66313972081441,-5.86769145362398));
#84069=CARTESIAN_POINT('',(140.,8.57388340516368,-7.51322323338386));
#84070=CARTESIAN_POINT('Origin',(140.,0.,0.));
#84071=CARTESIAN_POINT('',(140.,8.30850467894193,-7.24784450716211));
#84072=CARTESIAN_POINT('',(140.,7.79974746830583,-6.73908729652601));
#84073=CARTESIAN_POINT('',(140.,7.24784450716211,-8.30850467894194));
#84074=CARTESIAN_POINT('',(140.,10.893339635997,-4.66300955010707));
#84075=CARTESIAN_POINT('',(140.,7.51322323338385,-8.57388340516368));
#84076=CARTESIAN_POINT('',(140.,6.2087572106361,-7.26941738241592));
#84077=CARTESIAN_POINT('',(140.,6.33717014973236,-9.47630067554534));
#84078=CARTESIAN_POINT('Origin',(140.,0.,0.));
#84079=CARTESIAN_POINT('',(140.,6.14951905283832,-9.15127944162883));
#84080=CARTESIAN_POINT('',(140.,5.19951905283832,-7.50583117443839));
#84081=CARTESIAN_POINT('',(140.,4.85048094716166,-9.90127944162883));
#84082=CARTESIAN_POINT('',(140.,10.0997595264192,-6.87060704084318));
#84083=CARTESIAN_POINT('',(140.,5.03813204405571,-10.2263006755453));
#84084=CARTESIAN_POINT('',(140.,3.52548094716166,-7.60631212160006));
#84085=CARTESIAN_POINT('',(140.,3.66858922126564,-10.7935838869957));
#84086=CARTESIAN_POINT('Origin',(140.,0.,0.));
#84087=CARTESIAN_POINT('',(140.,3.57145386584452,-10.4310698053529));
#84088=CARTESIAN_POINT('',(140.,2.7238910008219,-7.26792213047979));
#84089=CARTESIAN_POINT('',(140.,2.12256512641092,-10.8192983730066));
#84090=CARTESIAN_POINT('',(140.,8.52740408177178,-9.10312694726631));
#84091=CARTESIAN_POINT('',(140.,2.21970048183204,-11.1818124546495));
#84092=CARTESIAN_POINT('',(140.,1.08088797756141,-6.93170632841676));
#84093=CARTESIAN_POINT('',(140.,0.749999999999998,-11.3753021937881));
#84094=CARTESIAN_POINT('Origin',(140.,0.,0.));
#84095=CARTESIAN_POINT('',(140.,0.749999999999998,-11.));
#84096=CARTESIAN_POINT('',(140.,0.749999999999998,-6.25));
#84097=CARTESIAN_POINT('',(140.,-0.750000000000002,-11.));
#84098=CARTESIAN_POINT('',(140.,6.075,-11.));
#84099=CARTESIAN_POINT('',(140.,-0.750000000000002,-11.3753021937881));
#84100=CARTESIAN_POINT('',(140.,-0.750000000000001,-5.5));
#84101=CARTESIAN_POINT('',(140.,-2.21970048183205,-11.1818124546495));
#84102=CARTESIAN_POINT('Origin',(140.,0.,0.));
#84103=CARTESIAN_POINT('',(140.,-2.12256512641094,-10.8192983730066));
#84104=CARTESIAN_POINT('',(140.,-0.511347062959607,-4.80615069813356));
#84105=CARTESIAN_POINT('',(140.,-3.57145386584454,-10.4310698053529));
#84106=CARTESIAN_POINT('',(140.,2.83338508951631,-12.1472412310932));
#84107=CARTESIAN_POINT('',(140.,-3.66858922126565,-10.7935838869957));
#84108=CARTESIAN_POINT('',(140.,-1.76612151856632,-3.69347776076298));
#84109=CARTESIAN_POINT('',(140.,-5.03813204405572,-10.2263006755453));
#84110=CARTESIAN_POINT('Origin',(140.,0.,0.));
#84111=CARTESIAN_POINT('',(140.,-4.85048094716168,-9.90127944162882));
#84112=CARTESIAN_POINT('',(140.,-1.05048094716167,-3.31948637286709));
#84113=CARTESIAN_POINT('',(140.,-6.14951905283833,-9.15127944162882));
#84114=CARTESIAN_POINT('',(140.,-0.900240473580843,-12.1819518424145));
#84115=CARTESIAN_POINT('',(140.,-6.33717014973238,-9.47630067554534));
#84116=CARTESIAN_POINT('',(140.,-1.97451905283833,-1.91996732002876));
#84117=CARTESIAN_POINT('',(140.,-7.51322323338386,-8.57388340516367));
#84118=CARTESIAN_POINT('Origin',(140.,0.,0.));
#84119=CARTESIAN_POINT('',(140.,-7.24784450716212,-8.30850467894193));
#84120=CARTESIAN_POINT('',(140.,-1.03908729652601,-2.09974746830583));
#84121=CARTESIAN_POINT('',(140.,-8.30850467894194,-7.24784450716211));
#84122=CARTESIAN_POINT('',(140.,-4.66300955010707,-10.893339635997));
#84123=CARTESIAN_POINT('',(140.,-8.57388340516368,-7.51322323338385));
#84124=CARTESIAN_POINT('',(140.,-1.56941738241592,-0.508757210636098));
#84125=CARTESIAN_POINT('',(140.,-9.47630067554534,-6.33717014973237));
#84126=CARTESIAN_POINT('Origin',(140.,0.,0.));
#84127=CARTESIAN_POINT('',(140.,-9.15127944162883,-6.14951905283833));
#84128=CARTESIAN_POINT('',(140.,-0.762658773652741,-1.30634665205268));
#84129=CARTESIAN_POINT('',(140.,-9.90127944162883,-4.85048094716167));
#84130=CARTESIAN_POINT('',(140.,-7.91377944162883,-8.29293192720481));
#84131=CARTESIAN_POINT('',(140.,-10.2263006755453,-5.03813204405571));
#84132=CARTESIAN_POINT('',(140.,-0.863139720814411,0.367691453623979));
#84133=CARTESIAN_POINT('',(140.,-10.7935838869957,-3.66858922126564));
#84134=CARTESIAN_POINT('Origin',(140.,0.,0.));
#84135=CARTESIAN_POINT('',(140.,-10.4310698053529,-3.57145386584453));
#84136=CARTESIAN_POINT('',(140.,-0.524749729694136,-0.917063401607555));
#84137=CARTESIAN_POINT('',(140.,-10.8192983730066,-2.12256512641092));
#84138=CARTESIAN_POINT('',(140.,-10.146299348052,-4.63423168098612));
#84139=CARTESIAN_POINT('',(140.,-11.1818124546495,-2.21970048183204));
#84140=CARTESIAN_POINT('',(140.,-0.188533927631114,0.725939621652937));
#84141=CARTESIAN_POINT('',(140.,-11.3753021937881,-0.749999999999999));
#84142=CARTESIAN_POINT('Origin',(140.,0.,0.));
#84143=CARTESIAN_POINT('',(140.,-11.,-0.749999999999999));
#84144=CARTESIAN_POINT('',(140.,-0.549999999999999,-0.75));
#84145=CARTESIAN_POINT('',(140.,-11.,0.750000000000001));
#84146=CARTESIAN_POINT('',(140.,-11.,-0.374999999999998));
#84147=CARTESIAN_POINT('',(140.,-11.3753021937881,0.750000000000001));
#84148=CARTESIAN_POINT('',(140.,0.2,0.75));
#84149=CARTESIAN_POINT('',(140.,-11.1818124546495,2.21970048183204));
#84150=CARTESIAN_POINT('Origin',(140.,0.,0.));
#84151=CARTESIAN_POINT('',(140.,-10.8192983730066,2.12256512641093));
#84152=CARTESIAN_POINT('',(140.,-0.912978297347917,-0.531825337826046));
#84153=CARTESIAN_POINT('',(140.,-10.4310698053529,3.57145386584453));
#84154=CARTESIAN_POINT('',(140.,-10.3404136318788,3.90978731126933));
#84155=CARTESIAN_POINT('',(140.,-10.7935838869957,3.66858922126565));
#84156=CARTESIAN_POINT('',(140.,0.199694640022666,0.722949117780665));
#84157=CARTESIAN_POINT('',(140.,-10.2263006755453,5.03813204405572));
#84158=CARTESIAN_POINT('Origin',(140.,0.,0.));
#84159=CARTESIAN_POINT('',(140.,-9.90127944162882,4.85048094716167));
#84160=CARTESIAN_POINT('',(140.,-1.51265877365274,0.00730854637602196));
#84161=CARTESIAN_POINT('',(140.,-9.15127944162882,6.14951905283833));
#84162=CARTESIAN_POINT('',(140.,-8.28877944162882,7.64341287436649));
#84163=CARTESIAN_POINT('',(140.,-9.47630067554534,6.33717014973237));
#84164=CARTESIAN_POINT('',(140.,-0.113139720814414,0.931346652052679));
#84165=CARTESIAN_POINT('',(140.,-8.57388340516368,7.51322323338386));
#84166=CARTESIAN_POINT('Origin',(140.,0.,0.));
#84167=CARTESIAN_POINT('',(140.,-8.30850467894193,7.24784450716211));
#84168=CARTESIAN_POINT('',(140.,-2.09974746830583,1.03908729652601));
#84169=CARTESIAN_POINT('',(140.,-7.24784450716211,8.30850467894193));
#84170=CARTESIAN_POINT('',(140.,-5.19333963599698,10.3630095501071));
#84171=CARTESIAN_POINT('',(140.,-7.51322323338385,8.57388340516368));
#84172=CARTESIAN_POINT('',(140.,-0.5087572106361,1.56941738241592));
#84173=CARTESIAN_POINT('',(140.,-6.33717014973237,9.47630067554534));
#84174=CARTESIAN_POINT('Origin',(140.,0.,0.));
#84175=CARTESIAN_POINT('',(140.,-6.14951905283833,9.15127944162883));
#84176=CARTESIAN_POINT('',(140.,-2.34951905283833,2.56948637286709));
#84177=CARTESIAN_POINT('',(140.,-4.85048094716167,9.90127944162883));
#84178=CARTESIAN_POINT('',(140.,-1.54975952641916,11.8069518424145));
#84179=CARTESIAN_POINT('',(140.,-5.03813204405571,10.2263006755453));
#84180=CARTESIAN_POINT('',(140.,-0.675480947161672,2.66996732002876));
#84181=CARTESIAN_POINT('',(140.,-3.66858922126564,10.7935838869957));
#84182=CARTESIAN_POINT('Origin',(140.,0.,0.));
#84183=CARTESIAN_POINT('',(140.,-3.57145386584453,10.4310698053529));
#84184=CARTESIAN_POINT('',(140.,-1.9602358023932,4.41792213047979));
#84185=CARTESIAN_POINT('',(140.,-2.12256512641093,10.8192983730066));
#84186=CARTESIAN_POINT('',(140.,2.10894071979952,11.9531269472663));
#84187=CARTESIAN_POINT('',(140.,-2.21970048183204,11.1818124546495));
#84188=CARTESIAN_POINT('',(140.,-0.317232779132713,4.08170632841677));
#84189=CARTESIAN_POINT('',(140.,-0.749999999999999,11.3753021937881));
#84190=CARTESIAN_POINT('Origin',(140.,0.,0.));
#84191=CARTESIAN_POINT('',(140.,-0.749999999999999,11.));
#84192=CARTESIAN_POINT('',(140.,-0.75,6.25));
#84193=CARTESIAN_POINT('',(140.,0.750000000000001,11.));
#84194=CARTESIAN_POINT('',(140.,5.325,11.));
#84195=CARTESIAN_POINT('',(140.,0.750000000000001,11.3753021937881));
#84196=CARTESIAN_POINT('',(140.,0.750000000000002,5.5));
#84197=CARTESIAN_POINT('',(140.,2.21970048183204,11.1818124546495));
#84198=CARTESIAN_POINT('Origin',(140.,0.,0.));
#84199=CARTESIAN_POINT('',(140.,2.12256512641093,10.8192983730066));
#84200=CARTESIAN_POINT('',(140.,1.2750022613883,7.65615069813357));
#84201=CARTESIAN_POINT('',(140.,3.57145386584453,10.4310698053529));
#84202=CARTESIAN_POINT('',(140.,7.80295971205498,9.2972412310932));
#84203=CARTESIAN_POINT('',(140.,3.66858922126565,10.7935838869957));
#84204=CARTESIAN_POINT('',(140.,2.52977671699502,6.54347776076299));
#84205=CARTESIAN_POINT('',(140.,5.03813204405571,10.2263006755453));
#84206=CARTESIAN_POINT('Origin',(140.,0.,0.));
#84207=CARTESIAN_POINT('',(140.,4.85048094716167,9.90127944162882));
#84208=CARTESIAN_POINT('',(140.,3.90048094716167,8.25583117443839));
#84209=CARTESIAN_POINT('',(140.,6.14951905283833,9.15127944162883));
#84210=CARTESIAN_POINT('',(140.,9.45024047358084,7.24560704084317));
#84211=CARTESIAN_POINT('',(140.,6.33717014973237,9.47630067554534));
#84212=CARTESIAN_POINT('',(140.,4.82451905283833,6.85631212160006));
#84213=CARTESIAN_POINT('',(140.,7.51322323338386,8.57388340516368));
#84214=CARTESIAN_POINT('Origin',(140.,0.,0.));
#84215=CARTESIAN_POINT('',(140.,7.24784450716211,8.30850467894193));
#84216=CARTESIAN_POINT('',(140.,6.73908729652601,7.79974746830583));
#84217=CARTESIAN_POINT('',(140.,8.30850467894193,7.24784450716211));
#84218=CARTESIAN_POINT('',(140.,10.3630095501071,5.19333963599698));
#84219=CARTESIAN_POINT('',(140.,8.57388340516368,7.51322323338386));
#84220=CARTESIAN_POINT('',(140.,7.26941738241592,6.2087572106361));
#84221=CARTESIAN_POINT('',(140.,9.47630067554534,6.33717014973237));
#84222=CARTESIAN_POINT('Origin',(140.,0.,0.));
#84223=CARTESIAN_POINT('',(140.,9.15127944162883,6.14951905283833));
#84224=CARTESIAN_POINT('',(140.,9.31265877365274,6.24269145362398));
#84225=CARTESIAN_POINT('',(140.,9.90127944162883,4.85048094716167));
#84226=CARTESIAN_POINT('',(140.,10.7637794416288,3.35658712563351));
#84227=CARTESIAN_POINT('',(140.,10.2263006755453,5.03813204405571));
#84228=CARTESIAN_POINT('',(140.,9.41313972081441,4.56865334794732));
#84229=CARTESIAN_POINT('',(140.,10.7935838869957,3.66858922126564));
#84230=CARTESIAN_POINT('Origin',(140.,0.,0.));
#84231=CARTESIAN_POINT('',(140.,10.4310698053529,3.57145386584453));
#84232=CARTESIAN_POINT('',(140.,11.1610945312654,3.76706340160756));
#84233=CARTESIAN_POINT('',(140.,10.8192983730066,2.12256512641093));
#84234=CARTESIAN_POINT('',(140.,10.9099545464807,1.78423168098613));
#84235=CARTESIAN_POINT('',(140.,11.1818124546495,2.21970048183204));
#84236=CARTESIAN_POINT('',(140.,10.8248787292024,2.12406037834706));
#84237=CARTESIAN_POINT('',(140.,11.3753021937881,0.75));
#84238=CARTESIAN_POINT('Origin',(140.,0.,0.));
#84239=CARTESIAN_POINT('',(140.,11.,0.75));
#84240=CARTESIAN_POINT('',(140.,11.95,0.75));
#84241=CARTESIAN_POINT('',(140.,11.,-0.75));
#84242=CARTESIAN_POINT('',(140.,11.,0.375));
#84243=CARTESIAN_POINT('',(140.,11.3753021937881,-0.75));
#84244=CARTESIAN_POINT('',(140.,11.2,-0.75));
#84245=CARTESIAN_POINT('Origin',(140.,0.,0.));
#84246=CARTESIAN_POINT('Origin',(140.3,0.,0.));
#84247=CARTESIAN_POINT('Ctrl Pts',(140.6,10.7469875144545,-5.33875073066341));
#84248=CARTESIAN_POINT('Ctrl Pts',(140.292275933538,10.4799686239773,-5.18458730236772));
#84249=CARTESIAN_POINT('Ctrl Pts',(140.,10.2263006755453,-5.03813204405571));
#84250=CARTESIAN_POINT('Origin',(140.3,0.,0.));
#84251=CARTESIAN_POINT('Ctrl Pts',(140.,11.3753021937881,-0.75));
#84252=CARTESIAN_POINT('Ctrl Pts',(140.292275932325,11.6682127091966,-0.75));
#84253=CARTESIAN_POINT('Ctrl Pts',(140.6,11.9765395670035,-0.75));
#84254=CARTESIAN_POINT('Origin',(139.,11.2003175473055,-5.60048094716168));
#84255=CARTESIAN_POINT('',(160.,9.90127944162882,-4.85048094716168));
#84256=CARTESIAN_POINT('',(160.,11.2003175473055,-5.60048094716168));
#84257=CARTESIAN_POINT('',(139.,9.90127944162882,-4.85048094716168));
#84258=CARTESIAN_POINT('Origin',(139.,9.90127944162882,-4.85048094716168));
#84259=CARTESIAN_POINT('',(160.,9.15127944162882,-6.14951905283833));
#84260=CARTESIAN_POINT('',(160.,9.90127944162882,-4.85048094716168));
#84261=CARTESIAN_POINT('',(139.,9.15127944162882,-6.14951905283833));
#84262=CARTESIAN_POINT('Origin',(139.,9.15127944162882,-6.14951905283833));
#84263=CARTESIAN_POINT('Ctrl Pts',(140.,9.47630067554532,-6.33717014973237));
#84264=CARTESIAN_POINT('Ctrl Pts',(140.292275928709,9.72996861978615,-6.48362540562459));
#84265=CARTESIAN_POINT('Ctrl Pts',(140.6,9.99698751445448,-6.63778883634007));
#84266=CARTESIAN_POINT('',(160.,9.15127944162882,-6.14951905283833));
#84267=CARTESIAN_POINT('Origin',(160.,10.1757984944672,-5.87500000000001));
#84268=CARTESIAN_POINT('Origin',(140.3,0.,0.));
#84269=CARTESIAN_POINT('Ctrl Pts',(140.6,8.99902242886706,-7.93836225708724));
#84270=CARTESIAN_POINT('Ctrl Pts',(140.292275929211,8.78100241468296,-7.72034224290314));
#84271=CARTESIAN_POINT('Ctrl Pts',(140.,8.57388340516366,-7.51322323338384));
#84272=CARTESIAN_POINT('Origin',(139.,9.36916485072175,-8.30850467894194));
#84273=CARTESIAN_POINT('',(160.,8.30850467894193,-7.24784450716211));
#84274=CARTESIAN_POINT('',(160.,9.36916485072175,-8.30850467894194));
#84275=CARTESIAN_POINT('',(139.,8.30850467894193,-7.24784450716211));
#84276=CARTESIAN_POINT('Origin',(139.,8.30850467894193,-7.24784450716211));
#84277=CARTESIAN_POINT('',(160.,7.24784450716211,-8.30850467894194));
#84278=CARTESIAN_POINT('',(160.,8.30850467894193,-7.24784450716211));
#84279=CARTESIAN_POINT('',(139.,7.24784450716211,-8.30850467894194));
#84280=CARTESIAN_POINT('Origin',(139.,7.24784450716211,-8.30850467894194));
#84281=CARTESIAN_POINT('Ctrl Pts',(140.,7.51322323338384,-8.57388340516367));
#84282=CARTESIAN_POINT('Ctrl Pts',(140.2922759308,7.72034224402904,-8.78100241580887));
#84283=CARTESIAN_POINT('Ctrl Pts',(140.6,7.93836225708724,-8.99902242886706));
#84284=CARTESIAN_POINT('',(160.,7.24784450716211,-8.30850467894194));
#84285=CARTESIAN_POINT('Origin',(160.,8.30850467894193,-8.30850467894194));
#84286=CARTESIAN_POINT('Origin',(140.3,0.,0.));
#84287=CARTESIAN_POINT('Ctrl Pts',(140.6,6.63778883634005,-9.99698751445449));
#84288=CARTESIAN_POINT('Ctrl Pts',(140.292275932638,6.48362540759328,-9.72996862319606));
#84289=CARTESIAN_POINT('Ctrl Pts',(140.,6.33717014973235,-9.47630067554533));
#84290=CARTESIAN_POINT('Origin',(139.,6.89951905283832,-10.4503175473055));
#84291=CARTESIAN_POINT('',(160.,6.14951905283832,-9.15127944162883));
#84292=CARTESIAN_POINT('',(160.,6.89951905283832,-10.4503175473055));
#84293=CARTESIAN_POINT('',(139.,6.14951905283832,-9.15127944162883));
#84294=CARTESIAN_POINT('Origin',(139.,6.14951905283832,-9.15127944162883));
#84295=CARTESIAN_POINT('',(160.,4.85048094716166,-9.90127944162883));
#84296=CARTESIAN_POINT('',(160.,6.14951905283832,-9.15127944162883));
#84297=CARTESIAN_POINT('',(139.,4.85048094716166,-9.90127944162883));
#84298=CARTESIAN_POINT('Origin',(139.,4.85048094716166,-9.90127944162883));
#84299=CARTESIAN_POINT('Ctrl Pts',(140.,5.0381320440557,-10.2263006755453));
#84300=CARTESIAN_POINT('Ctrl Pts',(140.292275927961,5.18458729957318,-10.4799686191371));
#84301=CARTESIAN_POINT('Ctrl Pts',(140.6,5.3387507306634,-10.7469875144545));
#84302=CARTESIAN_POINT('',(160.,4.85048094716166,-9.90127944162883));
#84303=CARTESIAN_POINT('Origin',(160.,5.87499999999999,-10.1757984944672));
#84304=CARTESIAN_POINT('Origin',(140.3,0.,0.));
#84305=CARTESIAN_POINT('Ctrl Pts',(140.6,3.82420090408119,-11.3743345935147));
#84306=CARTESIAN_POINT('Ctrl Pts',(140.292275926391,3.7444000396249,-11.0765137128759));
#84307=CARTESIAN_POINT('Ctrl Pts',(140.,3.66858922126563,-10.7935838869957));
#84308=CARTESIAN_POINT('Origin',(139.,3.9596824334983,-11.8799585447865));
#84309=CARTESIAN_POINT('',(160.,3.57145386584452,-10.4310698053529));
#84310=CARTESIAN_POINT('',(160.,3.9596824334983,-11.8799585447865));
#84311=CARTESIAN_POINT('',(139.,3.57145386584452,-10.4310698053529));
#84312=CARTESIAN_POINT('Origin',(139.,3.57145386584452,-10.4310698053529));
#84313=CARTESIAN_POINT('',(160.,2.12256512641092,-10.8192983730066));
#84314=CARTESIAN_POINT('',(160.,3.57145386584452,-10.4310698053529));
#84315=CARTESIAN_POINT('',(139.,2.12256512641092,-10.8192983730066));
#84316=CARTESIAN_POINT('Origin',(139.,2.12256512641092,-10.8192983730066));
#84317=CARTESIAN_POINT('Ctrl Pts',(140.,2.21970048183203,-11.1818124546495));
#84318=CARTESIAN_POINT('Ctrl Pts',(140.292275926381,2.29551130018881,-11.4647422805204));
#84319=CARTESIAN_POINT('Ctrl Pts',(140.6,2.37531216464759,-11.7625631611684));
#84320=CARTESIAN_POINT('',(160.,2.12256512641092,-10.8192983730066));
#84321=CARTESIAN_POINT('Origin',(160.,3.04112377995461,-11.3496284588966));
#84322=CARTESIAN_POINT('Origin',(140.3,0.,0.));
#84323=CARTESIAN_POINT('Ctrl Pts',(140.6,0.749999999999998,-11.9765395670035));
#84324=CARTESIAN_POINT('Ctrl Pts',(140.292275932325,0.749999999999998,-11.6682127091966));
#84325=CARTESIAN_POINT('Ctrl Pts',(140.,0.749999999999998,-11.3753021937881));
#84326=CARTESIAN_POINT('Origin',(139.,0.749999999999998,-12.5));
#84327=CARTESIAN_POINT('',(160.,0.749999999999998,-11.));
#84328=CARTESIAN_POINT('',(160.,0.749999999999998,-12.5));
#84329=CARTESIAN_POINT('',(139.,0.749999999999998,-11.));
#84330=CARTESIAN_POINT('Origin',(139.,0.749999999999998,-11.));
#84331=CARTESIAN_POINT('',(160.,-0.750000000000002,-11.));
#84332=CARTESIAN_POINT('',(160.,0.749999999999998,-11.));
#84333=CARTESIAN_POINT('',(139.,-0.750000000000002,-11.));
#84334=CARTESIAN_POINT('Origin',(139.,-0.750000000000002,-11.));
#84335=CARTESIAN_POINT('Ctrl Pts',(140.,-0.750000000000002,-11.3753021937881));
#84336=CARTESIAN_POINT('Ctrl Pts',(140.292275932325,-0.750000000000002,
-11.6682127091966));
#84337=CARTESIAN_POINT('Ctrl Pts',(140.6,-0.750000000000002,-11.9765395670035));
#84338=CARTESIAN_POINT('',(160.,-0.750000000000002,-11.));
#84339=CARTESIAN_POINT('Origin',(160.,-2.15843998349721E-15,-11.75));
#84340=CARTESIAN_POINT('Origin',(140.3,0.,0.));
#84341=CARTESIAN_POINT('Ctrl Pts',(140.6,-2.3753121646476,-11.7625631611684));
#84342=CARTESIAN_POINT('Ctrl Pts',(140.292275930713,-2.29551130131228,-11.4647422847132));
#84343=CARTESIAN_POINT('Ctrl Pts',(140.,-2.21970048183204,-11.1818124546495));
#84344=CARTESIAN_POINT('Origin',(139.,-2.51079369406472,-12.2681871124402));
#84345=CARTESIAN_POINT('',(160.,-2.12256512641094,-10.8192983730066));
#84346=CARTESIAN_POINT('',(160.,-2.51079369406472,-12.2681871124402));
#84347=CARTESIAN_POINT('',(139.,-2.12256512641094,-10.8192983730066));
#84348=CARTESIAN_POINT('Origin',(139.,-2.12256512641094,-10.8192983730066));
#84349=CARTESIAN_POINT('',(160.,-3.57145386584454,-10.4310698053529));
#84350=CARTESIAN_POINT('',(160.,-2.12256512641094,-10.8192983730066));
#84351=CARTESIAN_POINT('',(139.,-3.57145386584454,-10.4310698053529));
#84352=CARTESIAN_POINT('Origin',(139.,-3.57145386584454,-10.4310698053529));
#84353=CARTESIAN_POINT('Ctrl Pts',(140.,-3.66858922126565,-10.7935838869957));
#84354=CARTESIAN_POINT('Ctrl Pts',(140.29227593562,-3.74440004201855,-11.076513721809));
#84355=CARTESIAN_POINT('Ctrl Pts',(140.6,-3.82420090408121,-11.3743345935146));
#84356=CARTESIAN_POINT('',(160.,-3.57145386584454,-10.4310698053529));
#84357=CARTESIAN_POINT('Origin',(160.,-3.04112377995463,-11.3496284588966));
#84358=CARTESIAN_POINT('Origin',(140.3,0.,0.));
#84359=CARTESIAN_POINT('Ctrl Pts',(140.6,-5.33875073066341,-10.7469875144545));
#84360=CARTESIAN_POINT('Ctrl Pts',(140.29227593353,-5.18458730236325,-10.4799686239696));
#84361=CARTESIAN_POINT('Ctrl Pts',(140.,-5.03813204405571,-10.2263006755453));
#84362=CARTESIAN_POINT('Origin',(139.,-5.60048094716168,-11.2003175473055));
#84363=CARTESIAN_POINT('',(160.,-4.85048094716168,-9.90127944162882));
#84364=CARTESIAN_POINT('',(160.,-5.60048094716168,-11.2003175473055));
#84365=CARTESIAN_POINT('',(139.,-4.85048094716168,-9.90127944162882));
#84366=CARTESIAN_POINT('Origin',(139.,-4.85048094716168,-9.90127944162882));
#84367=CARTESIAN_POINT('',(160.,-6.14951905283833,-9.15127944162882));
#84368=CARTESIAN_POINT('',(160.,-4.85048094716168,-9.90127944162882));
#84369=CARTESIAN_POINT('',(139.,-6.14951905283833,-9.15127944162882));
#84370=CARTESIAN_POINT('Origin',(139.,-6.14951905283833,-9.15127944162882));
#84371=CARTESIAN_POINT('Ctrl Pts',(140.,-6.33717014973237,-9.47630067554532));
#84372=CARTESIAN_POINT('Ctrl Pts',(140.292275928709,-6.48362540562459,-9.72996861978615));
#84373=CARTESIAN_POINT('Ctrl Pts',(140.6,-6.63778883634007,-9.99698751445448));
#84374=CARTESIAN_POINT('',(160.,-6.14951905283833,-9.15127944162882));
#84375=CARTESIAN_POINT('Origin',(160.,-5.87500000000001,-10.1757984944672));
#84376=CARTESIAN_POINT('Origin',(140.3,0.,0.));
#84377=CARTESIAN_POINT('Ctrl Pts',(140.6,-7.93836225708724,-8.99902242886705));
#84378=CARTESIAN_POINT('Ctrl Pts',(140.292275935305,-7.72034224722101,-8.78100241900082));
#84379=CARTESIAN_POINT('Ctrl Pts',(140.,-7.51322323338385,-8.57388340516366));
#84380=CARTESIAN_POINT('Origin',(139.,-8.30850467894194,-9.36916485072175));
#84381=CARTESIAN_POINT('',(160.,-7.24784450716212,-8.30850467894193));
#84382=CARTESIAN_POINT('',(160.,-8.30850467894194,-9.36916485072175));
#84383=CARTESIAN_POINT('',(139.,-7.24784450716212,-8.30850467894193));
#84384=CARTESIAN_POINT('Origin',(139.,-7.24784450716212,-8.30850467894193));
#84385=CARTESIAN_POINT('',(160.,-8.30850467894194,-7.24784450716211));
#84386=CARTESIAN_POINT('',(160.,-7.24784450716212,-8.30850467894193));
#84387=CARTESIAN_POINT('',(139.,-8.30850467894194,-7.24784450716211));
#84388=CARTESIAN_POINT('Origin',(139.,-8.30850467894194,-7.24784450716211));
#84389=CARTESIAN_POINT('Ctrl Pts',(140.,-8.57388340516367,-7.51322323338384));
#84390=CARTESIAN_POINT('Ctrl Pts',(140.292275923422,-8.78100241058084,-7.72034223880101));
#84391=CARTESIAN_POINT('Ctrl Pts',(140.6,-8.99902242886706,-7.93836225708723));
#84392=CARTESIAN_POINT('',(160.,-8.30850467894194,-7.24784450716211));
#84393=CARTESIAN_POINT('Origin',(160.,-8.30850467894194,-8.30850467894193));
#84394=CARTESIAN_POINT('Origin',(140.3,0.,0.));
#84395=CARTESIAN_POINT('Ctrl Pts',(140.6,-9.99698751445449,-6.63778883634006));
#84396=CARTESIAN_POINT('Ctrl Pts',(140.292275936844,-9.72996862684556,-6.48362540970033));
#84397=CARTESIAN_POINT('Ctrl Pts',(140.,-9.47630067554532,-6.33717014973236));
#84398=CARTESIAN_POINT('Origin',(139.,-10.4503175473055,-6.89951905283833));
#84399=CARTESIAN_POINT('',(160.,-9.15127944162883,-6.14951905283833));
#84400=CARTESIAN_POINT('',(160.,-10.4503175473055,-6.89951905283833));
#84401=CARTESIAN_POINT('',(139.,-9.15127944162883,-6.14951905283833));
#84402=CARTESIAN_POINT('Origin',(139.,-9.15127944162883,-6.14951905283833));
#84403=CARTESIAN_POINT('',(160.,-9.90127944162883,-4.85048094716167));
#84404=CARTESIAN_POINT('',(160.,-9.15127944162883,-6.14951905283833));
#84405=CARTESIAN_POINT('',(139.,-9.90127944162883,-4.85048094716167));
#84406=CARTESIAN_POINT('Origin',(139.,-9.90127944162883,-4.85048094716167));
#84407=CARTESIAN_POINT('Ctrl Pts',(140.,-10.2263006755453,-5.0381320440557));
#84408=CARTESIAN_POINT('Ctrl Pts',(140.292275924103,-10.4799686157891,-5.18458729764023));
#84409=CARTESIAN_POINT('Ctrl Pts',(140.6,-10.7469875144545,-5.3387507306634));
#84410=CARTESIAN_POINT('',(160.,-9.90127944162883,-4.85048094716167));
#84411=CARTESIAN_POINT('Origin',(160.,-10.1757984944672,-5.875));
#84412=CARTESIAN_POINT('Origin',(140.3,0.,0.));
#84413=CARTESIAN_POINT('Ctrl Pts',(140.6,-11.3743345935147,-3.82420090408119));
#84414=CARTESIAN_POINT('Ctrl Pts',(140.292275926391,-11.0765137128759,-3.74440003962491));
#84415=CARTESIAN_POINT('Ctrl Pts',(140.,-10.7935838869957,-3.66858922126563));
#84416=CARTESIAN_POINT('Origin',(139.,-11.8799585447865,-3.95968243349831));
#84417=CARTESIAN_POINT('',(160.,-10.4310698053529,-3.57145386584453));
#84418=CARTESIAN_POINT('',(160.,-11.8799585447865,-3.95968243349831));
#84419=CARTESIAN_POINT('',(139.,-10.4310698053529,-3.57145386584453));
#84420=CARTESIAN_POINT('Origin',(139.,-10.4310698053529,-3.57145386584453));
#84421=CARTESIAN_POINT('',(160.,-10.8192983730066,-2.12256512641092));
#84422=CARTESIAN_POINT('',(160.,-10.4310698053529,-3.57145386584453));
#84423=CARTESIAN_POINT('',(139.,-10.8192983730066,-2.12256512641092));
#84424=CARTESIAN_POINT('Origin',(139.,-10.8192983730066,-2.12256512641092));
#84425=CARTESIAN_POINT('Ctrl Pts',(140.,-11.1818124546495,-2.21970048183203));
#84426=CARTESIAN_POINT('Ctrl Pts',(140.292275926391,-11.46474228053,-2.2955113001914));
#84427=CARTESIAN_POINT('Ctrl Pts',(140.6,-11.7625631611684,-2.37531216464759));
#84428=CARTESIAN_POINT('',(160.,-10.8192983730066,-2.12256512641092));
#84429=CARTESIAN_POINT('Origin',(160.,-11.3496284588966,-3.04112377995461));
#84430=CARTESIAN_POINT('Origin',(140.3,0.,0.));
#84431=CARTESIAN_POINT('Ctrl Pts',(140.6,-11.9765395670035,-0.749999999999999));
#84432=CARTESIAN_POINT('Ctrl Pts',(140.292275932325,-11.6682127091966,-0.749999999999999));
#84433=CARTESIAN_POINT('Ctrl Pts',(140.,-11.3753021937881,-0.749999999999999));
#84434=CARTESIAN_POINT('Origin',(139.,-12.5,-0.749999999999998));
#84435=CARTESIAN_POINT('',(160.,-11.,-0.749999999999999));
#84436=CARTESIAN_POINT('',(160.,-12.5,-0.749999999999998));
#84437=CARTESIAN_POINT('',(139.,-11.,-0.749999999999999));
#84438=CARTESIAN_POINT('Origin',(139.,-11.,-0.749999999999999));
#84439=CARTESIAN_POINT('',(160.,-11.,0.750000000000001));
#84440=CARTESIAN_POINT('',(160.,-11.,-0.749999999999999));
#84441=CARTESIAN_POINT('',(139.,-11.,0.750000000000001));
#84442=CARTESIAN_POINT('Origin',(139.,-11.,0.750000000000001));
#84443=CARTESIAN_POINT('Ctrl Pts',(140.,-11.3753021937881,0.750000000000002));
#84444=CARTESIAN_POINT('Ctrl Pts',(140.292275932325,-11.6682127091966,0.750000000000002));
#84445=CARTESIAN_POINT('Ctrl Pts',(140.6,-11.9765395670035,0.750000000000002));
#84446=CARTESIAN_POINT('',(160.,-11.,0.750000000000001));
#84447=CARTESIAN_POINT('Origin',(160.,-11.75,1.43895998899814E-15));
#84448=CARTESIAN_POINT('Origin',(140.3,0.,0.));
#84449=CARTESIAN_POINT('Ctrl Pts',(140.6,-11.7625631611684,2.3753121646476));
#84450=CARTESIAN_POINT('Ctrl Pts',(140.292275931144,-11.4647422851306,2.29551130142412));
#84451=CARTESIAN_POINT('Ctrl Pts',(140.,-11.1818124546495,2.21970048183204));
#84452=CARTESIAN_POINT('Origin',(139.,-12.2681871124402,2.51079369406471));
#84453=CARTESIAN_POINT('',(160.,-10.8192983730066,2.12256512641093));
#84454=CARTESIAN_POINT('',(160.,-12.2681871124402,2.51079369406471));
#84455=CARTESIAN_POINT('',(139.,-10.8192983730066,2.12256512641093));
#84456=CARTESIAN_POINT('Origin',(139.,-10.8192983730066,2.12256512641093));
#84457=CARTESIAN_POINT('',(160.,-10.4310698053529,3.57145386584453));
#84458=CARTESIAN_POINT('',(160.,-10.8192983730066,2.12256512641093));
#84459=CARTESIAN_POINT('',(139.,-10.4310698053529,3.57145386584453));
#84460=CARTESIAN_POINT('Origin',(139.,-10.4310698053529,3.57145386584453));
#84461=CARTESIAN_POINT('Ctrl Pts',(140.,-10.7935838869957,3.66858922126564));
#84462=CARTESIAN_POINT('Ctrl Pts',(140.292275930713,-11.0765137170592,3.74440004074584));
#84463=CARTESIAN_POINT('Ctrl Pts',(140.6,-11.3743345935147,3.8242009040812));
#84464=CARTESIAN_POINT('',(160.,-10.4310698053529,3.57145386584453));
#84465=CARTESIAN_POINT('Origin',(160.,-11.3496284588966,3.04112377995462));
#84466=CARTESIAN_POINT('Origin',(140.3,0.,0.));
#84467=CARTESIAN_POINT('Ctrl Pts',(140.6,-10.7469875144545,5.33875073066341));
#84468=CARTESIAN_POINT('Ctrl Pts',(140.292275935619,-10.4799686257831,5.18458730341029));
#84469=CARTESIAN_POINT('Ctrl Pts',(140.,-10.2263006755453,5.03813204405571));
#84470=CARTESIAN_POINT('Origin',(139.,-11.2003175473055,5.60048094716168));
#84471=CARTESIAN_POINT('',(160.,-9.90127944162882,4.85048094716167));
#84472=CARTESIAN_POINT('',(160.,-11.2003175473055,5.60048094716168));
#84473=CARTESIAN_POINT('',(139.,-9.90127944162882,4.85048094716167));
#84474=CARTESIAN_POINT('Origin',(139.,-9.90127944162882,4.85048094716167));
#84475=CARTESIAN_POINT('',(160.,-9.15127944162882,6.14951905283833));
#84476=CARTESIAN_POINT('',(160.,-9.90127944162882,4.85048094716167));
#84477=CARTESIAN_POINT('',(139.,-9.15127944162882,6.14951905283833));
#84478=CARTESIAN_POINT('Origin',(139.,-9.15127944162882,6.14951905283833));
#84479=CARTESIAN_POINT('Ctrl Pts',(140.,-9.47630067554532,6.33717014973237));
#84480=CARTESIAN_POINT('Ctrl Pts',(140.292275933541,-9.72996862397966,6.48362540804571));
#84481=CARTESIAN_POINT('Ctrl Pts',(140.6,-9.99698751445448,6.63778883634007));
#84482=CARTESIAN_POINT('',(160.,-9.15127944162882,6.14951905283833));
#84483=CARTESIAN_POINT('Origin',(160.,-10.1757984944672,5.875));
#84484=CARTESIAN_POINT('Origin',(140.3,0.,0.));
#84485=CARTESIAN_POINT('Ctrl Pts',(140.6,-8.99902242886706,7.93836225708724));
#84486=CARTESIAN_POINT('Ctrl Pts',(140.29227592312,-8.78100241036735,7.72034223858753));
#84487=CARTESIAN_POINT('Ctrl Pts',(140.,-8.57388340516366,7.51322323338384));
#84488=CARTESIAN_POINT('Origin',(139.,-9.36916485072175,8.30850467894193));
#84489=CARTESIAN_POINT('',(160.,-8.30850467894193,7.24784450716211));
#84490=CARTESIAN_POINT('',(160.,-9.36916485072175,8.30850467894193));
#84491=CARTESIAN_POINT('',(139.,-8.30850467894193,7.24784450716211));
#84492=CARTESIAN_POINT('Origin',(139.,-8.30850467894193,7.24784450716211));
#84493=CARTESIAN_POINT('',(160.,-7.24784450716211,8.30850467894193));
#84494=CARTESIAN_POINT('',(160.,-8.30850467894193,7.24784450716211));
#84495=CARTESIAN_POINT('',(139.,-7.24784450716211,8.30850467894193));
#84496=CARTESIAN_POINT('Origin',(139.,-7.24784450716211,8.30850467894193));
#84497=CARTESIAN_POINT('Ctrl Pts',(140.,-7.51322323338384,8.57388340516366));
#84498=CARTESIAN_POINT('Ctrl Pts',(140.292275929367,-7.72034224301365,8.78100241479348));
#84499=CARTESIAN_POINT('Ctrl Pts',(140.6,-7.93836225708724,8.99902242886706));
#84500=CARTESIAN_POINT('',(160.,-7.24784450716211,8.30850467894193));
#84501=CARTESIAN_POINT('Origin',(160.,-8.30850467894193,8.30850467894193));
#84502=CARTESIAN_POINT('Origin',(140.3,0.,0.));
#84503=CARTESIAN_POINT('Ctrl Pts',(140.6,-6.63778883634006,9.99698751445449));
#84504=CARTESIAN_POINT('Ctrl Pts',(140.29227593654,-6.48362540954844,9.72996862658248));
#84505=CARTESIAN_POINT('Ctrl Pts',(140.,-6.33717014973236,9.47630067554532));
#84506=CARTESIAN_POINT('Origin',(139.,-6.89951905283833,10.4503175473055));
#84507=CARTESIAN_POINT('',(160.,-6.14951905283833,9.15127944162883));
#84508=CARTESIAN_POINT('',(160.,-6.89951905283833,10.4503175473055));
#84509=CARTESIAN_POINT('',(139.,-6.14951905283833,9.15127944162883));
#84510=CARTESIAN_POINT('Origin',(139.,-6.14951905283833,9.15127944162883));
#84511=CARTESIAN_POINT('',(160.,-4.85048094716167,9.90127944162883));
#84512=CARTESIAN_POINT('',(160.,-6.14951905283833,9.15127944162883));
#84513=CARTESIAN_POINT('',(139.,-4.85048094716167,9.90127944162883));
#84514=CARTESIAN_POINT('Origin',(139.,-4.85048094716167,9.90127944162883));
#84515=CARTESIAN_POINT('Ctrl Pts',(140.,-5.0381320440557,10.2263006755453));
#84516=CARTESIAN_POINT('Ctrl Pts',(140.292275937175,-5.18458730418954,10.4799686271328));
#84517=CARTESIAN_POINT('Ctrl Pts',(140.6,-5.3387507306634,10.7469875144545));
#84518=CARTESIAN_POINT('',(160.,-4.85048094716167,9.90127944162883));
#84519=CARTESIAN_POINT('Origin',(160.,-5.875,10.1757984944672));
#84520=CARTESIAN_POINT('Origin',(140.3,0.,0.));
#84521=CARTESIAN_POINT('Ctrl Pts',(140.6,-3.82420090408119,11.3743345935147));
#84522=CARTESIAN_POINT('Ctrl Pts',(140.292275930439,-3.7444000406748,11.0765137167941));
#84523=CARTESIAN_POINT('Ctrl Pts',(140.,-3.66858922126564,10.7935838869957));
#84524=CARTESIAN_POINT('Origin',(139.,-3.95968243349831,11.8799585447865));
#84525=CARTESIAN_POINT('',(160.,-3.57145386584453,10.4310698053529));
#84526=CARTESIAN_POINT('',(160.,-3.95968243349831,11.8799585447865));
#84527=CARTESIAN_POINT('',(139.,-3.57145386584453,10.4310698053529));
#84528=CARTESIAN_POINT('Origin',(139.,-3.57145386584453,10.4310698053529));
#84529=CARTESIAN_POINT('',(160.,-2.12256512641093,10.8192983730066));
#84530=CARTESIAN_POINT('',(160.,-3.57145386584453,10.4310698053529));
#84531=CARTESIAN_POINT('',(139.,-2.12256512641093,10.8192983730066));
#84532=CARTESIAN_POINT('Origin',(139.,-2.12256512641093,10.8192983730066));
#84533=CARTESIAN_POINT('Ctrl Pts',(140.,-2.21970048183203,11.1818124546495));
#84534=CARTESIAN_POINT('Ctrl Pts',(140.292275926681,-2.29551130026667,11.4647422808109));
#84535=CARTESIAN_POINT('Ctrl Pts',(140.6,-2.37531216464759,11.7625631611684));
#84536=CARTESIAN_POINT('',(160.,-2.12256512641093,10.8192983730066));
#84537=CARTESIAN_POINT('Origin',(160.,-3.04112377995462,11.3496284588966));
#84538=CARTESIAN_POINT('Origin',(140.3,0.,0.));
#84539=CARTESIAN_POINT('Ctrl Pts',(140.6,-0.749999999999999,11.9765395670035));
#84540=CARTESIAN_POINT('Ctrl Pts',(140.292275932325,-0.749999999999999,
11.6682127091966));
#84541=CARTESIAN_POINT('Ctrl Pts',(140.,-0.749999999999999,11.3753021937881));
#84542=CARTESIAN_POINT('Origin',(139.,-0.749999999999999,12.5));
#84543=CARTESIAN_POINT('',(160.,-0.749999999999999,11.));
#84544=CARTESIAN_POINT('',(160.,-0.749999999999999,12.5));
#84545=CARTESIAN_POINT('',(139.,-0.749999999999999,11.));
#84546=CARTESIAN_POINT('Origin',(139.,-0.749999999999999,11.));
#84547=CARTESIAN_POINT('',(160.,0.750000000000001,11.));
#84548=CARTESIAN_POINT('',(160.,-0.749999999999999,11.));
#84549=CARTESIAN_POINT('',(139.,0.750000000000001,11.));
#84550=CARTESIAN_POINT('Origin',(139.,0.750000000000001,11.));
#84551=CARTESIAN_POINT('Ctrl Pts',(140.,0.750000000000001,11.3753021937881));
#84552=CARTESIAN_POINT('Ctrl Pts',(140.292275932325,0.750000000000001,11.6682127091966));
#84553=CARTESIAN_POINT('Ctrl Pts',(140.6,0.750000000000001,11.9765395670035));
#84554=CARTESIAN_POINT('',(160.,0.750000000000001,11.));
#84555=CARTESIAN_POINT('Origin',(160.,7.1947999449907E-16,11.75));
#84556=CARTESIAN_POINT('Origin',(140.3,0.,0.));
#84557=CARTESIAN_POINT('Ctrl Pts',(140.6,2.3753121646476,11.7625631611684));
#84558=CARTESIAN_POINT('Ctrl Pts',(140.292275926646,2.29551130025768,11.4647422807773));
#84559=CARTESIAN_POINT('Ctrl Pts',(140.,2.21970048183204,11.1818124546495));
#84560=CARTESIAN_POINT('Origin',(139.,2.51079369406471,12.2681871124402));
#84561=CARTESIAN_POINT('',(160.,2.12256512641093,10.8192983730066));
#84562=CARTESIAN_POINT('',(160.,2.51079369406471,12.2681871124402));
#84563=CARTESIAN_POINT('',(139.,2.12256512641093,10.8192983730066));
#84564=CARTESIAN_POINT('Origin',(139.,2.12256512641093,10.8192983730066));
#84565=CARTESIAN_POINT('',(160.,3.57145386584453,10.4310698053529));
#84566=CARTESIAN_POINT('',(160.,2.12256512641093,10.8192983730066));
#84567=CARTESIAN_POINT('',(139.,3.57145386584453,10.4310698053529));
#84568=CARTESIAN_POINT('Origin',(139.,3.57145386584453,10.4310698053529));
#84569=CARTESIAN_POINT('Ctrl Pts',(140.,3.66858922126564,10.7935838869957));
#84570=CARTESIAN_POINT('Ctrl Pts',(140.292275930864,3.74440004078502,11.0765137172054));
#84571=CARTESIAN_POINT('Ctrl Pts',(140.6,3.8242009040812,11.3743345935147));
#84572=CARTESIAN_POINT('',(160.,3.57145386584453,10.4310698053529));
#84573=CARTESIAN_POINT('Origin',(160.,3.04112377995462,11.3496284588966));
#84574=CARTESIAN_POINT('Origin',(140.3,0.,0.));
#84575=CARTESIAN_POINT('Ctrl Pts',(140.6,5.33875073066341,10.7469875144545));
#84576=CARTESIAN_POINT('Ctrl Pts',(140.292275928439,5.1845872998128,10.4799686195521));
#84577=CARTESIAN_POINT('Ctrl Pts',(140.,5.03813204405571,10.2263006755453));
#84578=CARTESIAN_POINT('Origin',(139.,5.60048094716167,11.2003175473055));
#84579=CARTESIAN_POINT('',(160.,4.85048094716167,9.90127944162882));
#84580=CARTESIAN_POINT('',(160.,5.60048094716167,11.2003175473055));
#84581=CARTESIAN_POINT('',(139.,4.85048094716167,9.90127944162882));
#84582=CARTESIAN_POINT('Origin',(139.,4.85048094716167,9.90127944162882));
#84583=CARTESIAN_POINT('',(160.,6.14951905283833,9.15127944162883));
#84584=CARTESIAN_POINT('',(160.,4.85048094716167,9.90127944162882));
#84585=CARTESIAN_POINT('',(139.,6.14951905283833,9.15127944162883));
#84586=CARTESIAN_POINT('Origin',(139.,6.14951905283833,9.15127944162883));
#84587=CARTESIAN_POINT('Ctrl Pts',(140.,6.33717014973236,9.47630067554532));
#84588=CARTESIAN_POINT('Ctrl Pts',(140.292275936827,6.48362540969219,9.72996862683144));
#84589=CARTESIAN_POINT('Ctrl Pts',(140.6,6.63778883634006,9.99698751445448));
#84590=CARTESIAN_POINT('',(160.,6.14951905283833,9.15127944162883));
#84591=CARTESIAN_POINT('Origin',(160.,5.875,10.1757984944672));
#84592=CARTESIAN_POINT('Origin',(140.3,0.,0.));
#84593=CARTESIAN_POINT('Ctrl Pts',(140.6,7.93836225708724,8.99902242886706));
#84594=CARTESIAN_POINT('Ctrl Pts',(140.292275929512,7.72034224311662,8.78100241489644));
#84595=CARTESIAN_POINT('Ctrl Pts',(140.,7.51322323338384,8.57388340516366));
#84596=CARTESIAN_POINT('Origin',(139.,8.30850467894193,9.36916485072176));
#84597=CARTESIAN_POINT('',(160.,7.24784450716211,8.30850467894193));
#84598=CARTESIAN_POINT('',(160.,8.30850467894193,9.36916485072176));
#84599=CARTESIAN_POINT('',(139.,7.24784450716211,8.30850467894193));
#84600=CARTESIAN_POINT('Origin',(139.,7.24784450716211,8.30850467894193));
#84601=CARTESIAN_POINT('',(160.,8.30850467894193,7.24784450716211));
#84602=CARTESIAN_POINT('',(160.,7.24784450716211,8.30850467894193));
#84603=CARTESIAN_POINT('',(139.,8.30850467894193,7.24784450716211));
#84604=CARTESIAN_POINT('Origin',(139.,8.30850467894193,7.24784450716211));
#84605=CARTESIAN_POINT('Ctrl Pts',(140.,8.57388340516366,7.51322323338384));
#84606=CARTESIAN_POINT('Ctrl Pts',(140.292275929512,8.78100241489644,7.72034224311662));
#84607=CARTESIAN_POINT('Ctrl Pts',(140.6,8.99902242886706,7.93836225708724));
#84608=CARTESIAN_POINT('',(160.,8.30850467894193,7.24784450716211));
#84609=CARTESIAN_POINT('Origin',(160.,8.30850467894193,8.30850467894193));
#84610=CARTESIAN_POINT('Origin',(140.3,0.,0.));
#84611=CARTESIAN_POINT('Ctrl Pts',(140.6,9.99698751445448,6.63778883634006));
#84612=CARTESIAN_POINT('Ctrl Pts',(140.292275932495,9.72996862307203,6.48362540752169));
#84613=CARTESIAN_POINT('Ctrl Pts',(140.,9.47630067554532,6.33717014973236));
#84614=CARTESIAN_POINT('Origin',(139.,10.4503175473055,6.89951905283833));
#84615=CARTESIAN_POINT('',(160.,9.15127944162883,6.14951905283833));
#84616=CARTESIAN_POINT('',(160.,10.4503175473055,6.89951905283833));
#84617=CARTESIAN_POINT('',(139.,9.15127944162883,6.14951905283833));
#84618=CARTESIAN_POINT('Origin',(139.,9.15127944162883,6.14951905283833));
#84619=CARTESIAN_POINT('',(160.,9.90127944162883,4.85048094716167));
#84620=CARTESIAN_POINT('',(160.,9.15127944162883,6.14951905283833));
#84621=CARTESIAN_POINT('',(139.,9.90127944162883,4.85048094716167));
#84622=CARTESIAN_POINT('Origin',(139.,9.90127944162883,4.85048094716167));
#84623=CARTESIAN_POINT('Ctrl Pts',(140.,10.2263006755453,5.0381320440557));
#84624=CARTESIAN_POINT('Ctrl Pts',(140.292275928697,10.4799686197761,5.18458729994212));
#84625=CARTESIAN_POINT('Ctrl Pts',(140.6,10.7469875144545,5.3387507306634));
#84626=CARTESIAN_POINT('',(160.,9.90127944162883,4.85048094716167));
#84627=CARTESIAN_POINT('Origin',(160.,10.1757984944672,5.875));
#84628=CARTESIAN_POINT('Origin',(140.3,0.,0.));
#84629=CARTESIAN_POINT('Ctrl Pts',(140.6,11.3743345935147,3.82420090408119));
#84630=CARTESIAN_POINT('Ctrl Pts',(140.292275930711,11.0765137170573,3.74440004074531));
#84631=CARTESIAN_POINT('Ctrl Pts',(140.,10.7935838869957,3.66858922126564));
#84632=CARTESIAN_POINT('Origin',(139.,11.8799585447865,3.95968243349831));
#84633=CARTESIAN_POINT('',(160.,10.4310698053529,3.57145386584453));
#84634=CARTESIAN_POINT('',(160.,11.8799585447865,3.95968243349831));
#84635=CARTESIAN_POINT('',(139.,10.4310698053529,3.57145386584453));
#84636=CARTESIAN_POINT('Origin',(139.,10.4310698053529,3.57145386584453));
#84637=CARTESIAN_POINT('',(160.,10.8192983730066,2.12256512641093));
#84638=CARTESIAN_POINT('',(160.,10.4310698053529,3.57145386584453));
#84639=CARTESIAN_POINT('',(139.,10.8192983730066,2.12256512641093));
#84640=CARTESIAN_POINT('Origin',(139.,10.8192983730066,2.12256512641093));
#84641=CARTESIAN_POINT('Ctrl Pts',(140.,11.1818124546495,2.21970048183203));
#84642=CARTESIAN_POINT('Ctrl Pts',(140.29227592667,11.4647422808006,2.2955113002639));
#84643=CARTESIAN_POINT('Ctrl Pts',(140.6,11.7625631611684,2.37531216464759));
#84644=CARTESIAN_POINT('',(160.,10.8192983730066,2.12256512641093));
#84645=CARTESIAN_POINT('Origin',(160.,11.3496284588966,3.04112377995462));
#84646=CARTESIAN_POINT('Origin',(140.3,0.,0.));
#84647=CARTESIAN_POINT('Ctrl Pts',(140.6,11.9765395670035,0.75));
#84648=CARTESIAN_POINT('Ctrl Pts',(140.292275932325,11.6682127091966,0.75));
#84649=CARTESIAN_POINT('Ctrl Pts',(140.,11.3753021937881,0.75));
#84650=CARTESIAN_POINT('Origin',(139.,12.5,0.75));
#84651=CARTESIAN_POINT('',(160.,11.,0.75));
#84652=CARTESIAN_POINT('',(160.,12.5,0.75));
#84653=CARTESIAN_POINT('',(139.,11.,0.75));
#84654=CARTESIAN_POINT('Origin',(139.,11.,0.75));
#84655=CARTESIAN_POINT('',(160.,11.,-0.75));
#84656=CARTESIAN_POINT('',(160.,11.,0.75));
#84657=CARTESIAN_POINT('',(139.,11.,-0.75));
#84658=CARTESIAN_POINT('Origin',(139.,11.,-0.75));
#84659=CARTESIAN_POINT('',(160.,11.,-0.75));
#84660=CARTESIAN_POINT('Origin',(160.,11.75,0.));
#84661=CARTESIAN_POINT('Origin',(536.,0.,0.));
#90347=UNCERTAINTY_MEASURE_WITH_UNIT(LENGTH_MEASURE(0.01),#90375,
'DISTANCE_ACCURACY_VALUE',
'Maximum model space distance between geometric entities at asserted c
onnectivities');
#90355=UNCERTAINTY_MEASURE_WITH_UNIT(LENGTH_MEASURE(0.01),#90375,
'DISTANCE_ACCURACY_VALUE',
'Maximum model space distance between geometric entities at asserted c
onnectivities');
#90366=(
GEOMETRIC_REPRESENTATION_CONTEXT(3)
GLOBAL_UNCERTAINTY_ASSIGNED_CONTEXT((#90347))
GLOBAL_UNIT_ASSIGNED_CONTEXT((#90375,#90377,#90378))
REPRESENTATION_CONTEXT('','3D')
);
#90374=(
GEOMETRIC_REPRESENTATION_CONTEXT(3)
GLOBAL_UNCERTAINTY_ASSIGNED_CONTEXT((#90355))
GLOBAL_UNIT_ASSIGNED_CONTEXT((#90375,#90377,#90378))
REPRESENTATION_CONTEXT('','3D')
);
#90375=(
LENGTH_UNIT()
NAMED_UNIT(*)
SI_UNIT(.MILLI.,.METRE.)
);
#90377=(
NAMED_UNIT(*)
PLANE_ANGLE_UNIT()
SI_UNIT($,.RADIAN.)
);
#90378=(
NAMED_UNIT(*)
SI_UNIT($,.STERADIAN.)
SOLID_ANGLE_UNIT()
);
#90389=SHAPE_DEFINITION_REPRESENTATION(#90407,#90450);
#90407=PRODUCT_DEFINITION_SHAPE('',$,#90469);
#90450=SHAPE_REPRESENTATION('',(#43845),#90366);
#90458=PRODUCT_DEFINITION_CONTEXT('part definition',#90514,'design');
#90469=PRODUCT_DEFINITION('2026-10-11-12-53-11-424','10_Axle_Bar_Shaft',
#90487,#90458);
#90487=PRODUCT_DEFINITION_FORMATION('',$,#90526);
#90514=APPLICATION_CONTEXT(
'Core Data for Automotive Mechanical Design Process');
#90515=PRODUCT_CONTEXT('part definition',#90514,'mechanical');
#90526=PRODUCT('2026-10-11-12-53-11-424','10_Axle_Bar_Shaft',$,(#90515));
#90681=COLOUR_RGB('Grey',0.48,0.52,0.57);
#90682=FILL_AREA_STYLE_COLOUR('',#90681);
#90683=FILL_AREA_STYLE('',(#90682));
#90684=SURFACE_STYLE_FILL_AREA(#90683);
#90685=SURFACE_SIDE_STYLE('',(#90684));
#90686=SURFACE_STYLE_USAGE(.BOTH.,#90685);
#90687=PRESENTATION_STYLE_ASSIGNMENT((#90686));
ENDSEC;
END-ISO-10303-21;
